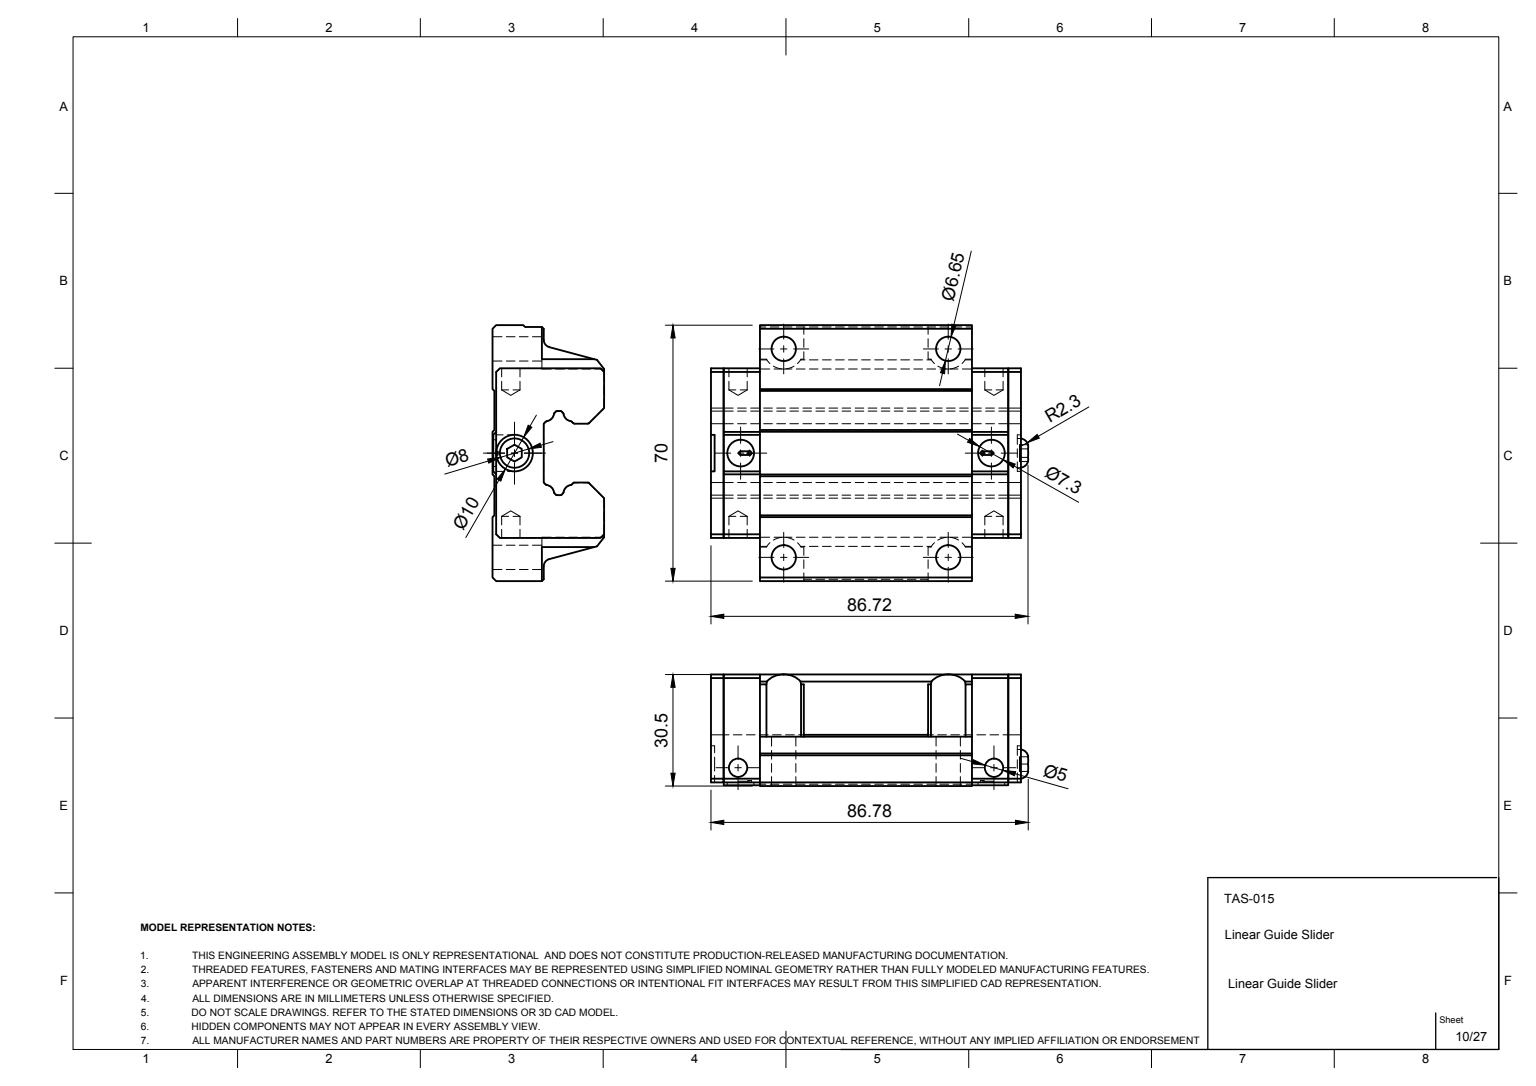
ISO-10303-21;
HEADER;
/* Generated by software containing ST-Developer
 * from STEP Tools, Inc. (www.steptools.com) 
 */

FILE_DESCRIPTION(
/* description */ ('STEP AP214'),
/* implementation_level */ '2;1');

FILE_NAME(
/* name */ 'Linear Guide Slider.step',
/* time_stamp */ '2026-11-15T14:49:54-08:00',
/* author */ (''),
/* organization */ (''),
/* preprocessor_version */ 'ST-DEVELOPER v20.2',
/* originating_system */ 'Autodesk Translation Framework v15.17.0.0',
/* authorisation */ '');

FILE_SCHEMA (('AUTOMOTIVE_DESIGN { 1 0 10303 214 3 1 1 }'));
ENDSEC;

DATA;
#10=MECHANICAL_DESIGN_GEOMETRIC_PRESENTATION_REPRESENTATION('',(#1105),#66721);
#82=(
BOUNDED_CURVE()
B_SPLINE_CURVE(2,(#37654,#37655,#37656),.UNSPECIFIED.,.F.,.F.)
B_SPLINE_CURVE_WITH_KNOTS((3,3),(-1.29356557390797,0.),.UNSPECIFIED.)
CURVE()
GEOMETRIC_REPRESENTATION_ITEM()
RATIONAL_B_SPLINE_CURVE((0.954658532851732,0.77704632554749,1.))
REPRESENTATION_ITEM('')
);
#109=B_SPLINE_CURVE_WITH_KNOTS('',3,(#37621,#37622,#37623,#37624,#37625,
#37626,#37627,#37628,#37629,#37630),.UNSPECIFIED.,.F.,.F.,(4,2,2,2,4),(-0.991617660219933,
-0.988360888345703,-0.882558915285875,-0.776756942226048,-0.773500170351817),
 .UNSPECIFIED.);
#110=B_SPLINE_CURVE_WITH_KNOTS('',3,(#37632,#37633,#37634,#37635,#37636,
#37637,#37638,#37639,#37640,#37641),.UNSPECIFIED.,.F.,.F.,(4,2,2,2,4),(-0.991617660219933,
-0.988360888345703,-0.882558915285875,-0.776756942226048,-0.773500170351817),
 .UNSPECIFIED.);
#111=B_SPLINE_CURVE_WITH_KNOTS('',3,(#37643,#37644,#37645,#37646,#37647,
#37648,#37649,#37650,#37651,#37652),.UNSPECIFIED.,.F.,.F.,(4,2,2,2,4),(-0.991617660219934,
-0.988360888345704,-0.882558915285876,-0.776756942226048,-0.773500170351818),
 .UNSPECIFIED.);
#112=B_SPLINE_CURVE_WITH_KNOTS('',3,(#37661,#37662,#37663,#37664,#37665,
#37666,#37667,#37668,#37669,#37670),.UNSPECIFIED.,.F.,.F.,(4,2,2,2,4),(0.773500170351818,
0.776756942226048,0.882558915285876,0.988360888345703,0.991617660219934),
 .UNSPECIFIED.);
#113=B_SPLINE_CURVE_WITH_KNOTS('',3,(#37672,#37673,#37674,#37675,#37676,
#37677,#37678,#37679,#37680,#37681),.UNSPECIFIED.,.F.,.F.,(4,2,2,2,4),(0.773500170351817,
0.776756942226048,0.882558915285875,0.988360888345703,0.991617660219933),
 .UNSPECIFIED.);
#114=B_SPLINE_CURVE_WITH_KNOTS('',3,(#37682,#37683,#37684,#37685,#37686,
#37687,#37688,#37689,#37690,#37691),.UNSPECIFIED.,.F.,.F.,(4,2,2,2,4),(0.773500170351818,
0.776756942226048,0.882558915285876,0.988360888345704,0.991617660219934),
 .UNSPECIFIED.);
#402=(
BOUNDED_SURFACE()
B_SPLINE_SURFACE(2,2,((#37592,#37593,#37594,#37595,#37596,#37597,#37598,
#37599,#37600),(#37601,#37602,#37603,#37604,#37605,#37606,#37607,#37608,
#37609),(#37610,#37611,#37612,#37613,#37614,#37615,#37616,#37617,#37618)),
 .UNSPECIFIED.,.F.,.T.,.F.)
B_SPLINE_SURFACE_WITH_KNOTS((3,3),(3,2,2,2,3),(0.,1.43998883071719),(-3.14159265358979,
-1.5707963267949,0.,1.5707963267949,3.14159265358979),.UNSPECIFIED.)
GEOMETRIC_REPRESENTATION_ITEM()
RATIONAL_B_SPLINE_SURFACE(((1.,0.707106781186548,1.,0.707106781186548,1.,
0.707106781186548,1.,0.707106781186548,1.),(0.751809411556116,0.531609533071198,
0.751809411556116,0.531609533071198,0.751809411556116,0.531609533071198,
0.751809411556116,0.531609533071198,0.751809411556116),(1.,0.707106781186548,
1.,0.707106781186548,1.,0.707106781186548,1.,0.707106781186548,1.)))
REPRESENTATION_ITEM('')
SURFACE()
);
#524=CONICAL_SURFACE('',#26602,2.5,1.02974425867665);
#525=CONICAL_SURFACE('',#26603,2.5,1.02974425867665);
#526=CONICAL_SURFACE('',#26629,2.5,1.02974425867665);
#527=CONICAL_SURFACE('',#26630,2.5,1.02974425867665);
#642=ELLIPSE('',#26643,6.97960018289555,5.49999999999817);
#643=ELLIPSE('',#26645,6.97960018289945,5.50000000000025);
#644=ELLIPSE('',#26646,6.97960018289465,5.49999999999756);
#645=ELLIPSE('',#26648,6.97960018289959,5.50000000000032);
#646=ELLIPSE('',#26649,6.97960018289765,5.49999999999922);
#647=ELLIPSE('',#26651,6.9796001828989,5.49999999999987);
#648=ELLIPSE('',#26972,21.2503681783598,5.50000000000001);
#649=ELLIPSE('',#26973,21.2503681783597,5.5);
#650=ELLIPSE('',#26978,21.2503681783597,5.5);
#651=ELLIPSE('',#26983,21.2503681783597,5.5);
#652=ELLIPSE('',#26985,21.2503681783597,5.49999999999999);
#653=ELLIPSE('',#26986,21.2503681783597,5.5);
#654=ELLIPSE('',#27079,21.2503681783598,5.50000000000001);
#655=ELLIPSE('',#27081,21.2503681783597,5.49999999999999);
#656=ELLIPSE('',#27086,6.97960018290351,5.50000000000224);
#657=ELLIPSE('',#27091,6.97960018290198,5.50000000000146);
#1043=SHAPE_REPRESENTATION_RELATIONSHIP('SRR','None',#66901,#1074);
#1074=ADVANCED_BREP_SHAPE_REPRESENTATION('',(#1140),#66692);
#1105=STYLED_ITEM('',(#67095),#1140);
#1140=MANIFOLD_SOLID_BREP('Body1',#25671);
#1277=FACE_BOUND('',#4113,.T.);
#1278=FACE_BOUND('',#4116,.T.);
#1279=FACE_BOUND('',#4131,.T.);
#1280=FACE_BOUND('',#4229,.T.);
#1281=FACE_BOUND('',#4242,.T.);
#1282=FACE_BOUND('',#4250,.T.);
#1283=FACE_BOUND('',#4253,.T.);
#1284=FACE_BOUND('',#4258,.T.);
#1285=FACE_BOUND('',#4306,.T.);
#1286=FACE_BOUND('',#4311,.T.);
#1287=FACE_BOUND('',#4313,.T.);
#1288=FACE_BOUND('',#4320,.T.);
#1289=FACE_BOUND('',#4321,.T.);
#1290=FACE_BOUND('',#4330,.T.);
#1291=FACE_BOUND('',#4331,.T.);
#1292=FACE_BOUND('',#4337,.T.);
#1293=FACE_BOUND('',#4343,.T.);
#1294=FACE_BOUND('',#4350,.T.);
#1295=FACE_BOUND('',#4355,.T.);
#1296=FACE_BOUND('',#4390,.T.);
#1297=FACE_BOUND('',#4402,.T.);
#1298=FACE_BOUND('',#4404,.T.);
#1637=PLANE('',#26642);
#1638=PLANE('',#26644);
#1639=PLANE('',#26647);
#1640=PLANE('',#26650);
#1641=PLANE('',#26652);
#1642=PLANE('',#26653);
#1643=PLANE('',#26654);
#1644=PLANE('',#26655);
#1645=PLANE('',#26656);
#1646=PLANE('',#26657);
#1647=PLANE('',#26658);
#1648=PLANE('',#26659);
#1649=PLANE('',#26660);
#1650=PLANE('',#26661);
#1651=PLANE('',#26662);
#1652=PLANE('',#26663);
#1653=PLANE('',#26664);
#1654=PLANE('',#26665);
#1655=PLANE('',#26666);
#1656=PLANE('',#26667);
#1657=PLANE('',#26668);
#1658=PLANE('',#26729);
#1659=PLANE('',#26730);
#1660=PLANE('',#26731);
#1661=PLANE('',#26732);
#1662=PLANE('',#26733);
#1663=PLANE('',#26734);
#1664=PLANE('',#26735);
#1665=PLANE('',#26736);
#1666=PLANE('',#26737);
#1667=PLANE('',#26738);
#1668=PLANE('',#26739);
#1669=PLANE('',#26740);
#1670=PLANE('',#26741);
#1671=PLANE('',#26742);
#1672=PLANE('',#26743);
#1673=PLANE('',#26744);
#1674=PLANE('',#26745);
#1675=PLANE('',#26766);
#1676=PLANE('',#26769);
#1677=PLANE('',#26772);
#1678=PLANE('',#26779);
#1679=PLANE('',#26782);
#1680=PLANE('',#26785);
#1681=PLANE('',#26792);
#1682=PLANE('',#26793);
#1683=PLANE('',#26794);
#1684=PLANE('',#26801);
#1685=PLANE('',#26804);
#1686=PLANE('',#26807);
#1687=PLANE('',#26814);
#1688=PLANE('',#26817);
#1689=PLANE('',#26820);
#1690=PLANE('',#26821);
#1691=PLANE('',#26822);
#1692=PLANE('',#26823);
#1693=PLANE('',#26824);
#1694=PLANE('',#26825);
#1695=PLANE('',#26826);
#1696=PLANE('',#26827);
#1697=PLANE('',#26828);
#1698=PLANE('',#26829);
#1699=PLANE('',#26830);
#1700=PLANE('',#26831);
#1701=PLANE('',#26833);
#1702=PLANE('',#26855);
#1703=PLANE('',#26856);
#1704=PLANE('',#26859);
#1705=PLANE('',#26860);
#1706=PLANE('',#26862);
#1707=PLANE('',#26863);
#1708=PLANE('',#26864);
#1709=PLANE('',#26865);
#1710=PLANE('',#26866);
#1711=PLANE('',#26867);
#1712=PLANE('',#26868);
#1713=PLANE('',#26869);
#1714=PLANE('',#26870);
#1715=PLANE('',#26871);
#1716=PLANE('',#26874);
#1717=PLANE('',#26877);
#1718=PLANE('',#26884);
#1719=PLANE('',#26887);
#1720=PLANE('',#26890);
#1721=PLANE('',#26897);
#1722=PLANE('',#26898);
#1723=PLANE('',#26899);
#1724=PLANE('',#26906);
#1725=PLANE('',#26909);
#1726=PLANE('',#26912);
#1727=PLANE('',#26919);
#1728=PLANE('',#26922);
#1729=PLANE('',#26925);
#1730=PLANE('',#26926);
#1731=PLANE('',#26927);
#1732=PLANE('',#26928);
#1733=PLANE('',#26929);
#1734=PLANE('',#26930);
#1735=PLANE('',#26936);
#1736=PLANE('',#26937);
#1737=PLANE('',#26938);
#1738=PLANE('',#26939);
#1739=PLANE('',#26943);
#1740=PLANE('',#26964);
#1741=PLANE('',#26965);
#1742=PLANE('',#26966);
#1743=PLANE('',#26967);
#1744=PLANE('',#26968);
#1745=PLANE('',#26969);
#1746=PLANE('',#26970);
#1747=PLANE('',#26971);
#1748=PLANE('',#26974);
#1749=PLANE('',#26976);
#1750=PLANE('',#26977);
#1751=PLANE('',#26979);
#1752=PLANE('',#26980);
#1753=PLANE('',#26982);
#1754=PLANE('',#26984);
#1755=PLANE('',#26987);
#1756=PLANE('',#26988);
#1757=PLANE('',#26989);
#1758=PLANE('',#26990);
#1759=PLANE('',#26991);
#1760=PLANE('',#26992);
#1761=PLANE('',#26993);
#1762=PLANE('',#26994);
#1763=PLANE('',#26995);
#1764=PLANE('',#26996);
#1765=PLANE('',#26999);
#1766=PLANE('',#27002);
#1767=PLANE('',#27009);
#1768=PLANE('',#27012);
#1769=PLANE('',#27015);
#1770=PLANE('',#27022);
#1771=PLANE('',#27023);
#1772=PLANE('',#27024);
#1773=PLANE('',#27031);
#1774=PLANE('',#27034);
#1775=PLANE('',#27037);
#1776=PLANE('',#27044);
#1777=PLANE('',#27047);
#1778=PLANE('',#27050);
#1779=PLANE('',#27051);
#1780=PLANE('',#27052);
#1781=PLANE('',#27053);
#1782=PLANE('',#27054);
#1783=PLANE('',#27055);
#1784=PLANE('',#27056);
#1785=PLANE('',#27057);
#1786=PLANE('',#27058);
#1787=PLANE('',#27059);
#1788=PLANE('',#27060);
#1789=PLANE('',#27061);
#1790=PLANE('',#27062);
#1791=PLANE('',#27063);
#1792=PLANE('',#27064);
#1793=PLANE('',#27065);
#1794=PLANE('',#27066);
#1795=PLANE('',#27067);
#1796=PLANE('',#27068);
#1797=PLANE('',#27069);
#1798=PLANE('',#27070);
#1799=PLANE('',#27071);
#1800=PLANE('',#27072);
#1801=PLANE('',#27073);
#1802=PLANE('',#27074);
#1803=PLANE('',#27075);
#1804=PLANE('',#27077);
#1805=PLANE('',#27078);
#1806=PLANE('',#27080);
#1807=PLANE('',#27082);
#1808=PLANE('',#27083);
#1809=PLANE('',#27085);
#1810=PLANE('',#27087);
#1811=PLANE('',#27088);
#1812=PLANE('',#27089);
#1813=PLANE('',#27090);
#1814=PLANE('',#27092);
#1815=PLANE('',#27113);
#1816=PLANE('',#27114);
#1817=PLANE('',#27115);
#1818=PLANE('',#27116);
#1819=PLANE('',#27117);
#1820=PLANE('',#27118);
#1821=PLANE('',#27123);
#1822=PLANE('',#27124);
#1823=PLANE('',#27125);
#1824=PLANE('',#27136);
#1825=PLANE('',#27137);
#1826=PLANE('',#27144);
#1827=PLANE('',#27145);
#1828=PLANE('',#27156);
#1829=PLANE('',#27157);
#1830=PLANE('',#27158);
#1831=PLANE('',#27169);
#1832=PLANE('',#27170);
#1833=PLANE('',#27171);
#1834=PLANE('',#27172);
#1835=PLANE('',#27173);
#1836=PLANE('',#27174);
#1837=PLANE('',#27175);
#1838=PLANE('',#27176);
#1839=PLANE('',#27177);
#1840=PLANE('',#27178);
#1841=PLANE('',#27179);
#1842=PLANE('',#27180);
#1843=PLANE('',#27181);
#1844=PLANE('',#27182);
#1845=PLANE('',#27183);
#1846=PLANE('',#27186);
#1847=PLANE('',#27187);
#2501=FACE_OUTER_BOUND('',#4052,.T.);
#2502=FACE_OUTER_BOUND('',#4053,.T.);
#2503=FACE_OUTER_BOUND('',#4054,.T.);
#2504=FACE_OUTER_BOUND('',#4055,.T.);
#2505=FACE_OUTER_BOUND('',#4056,.T.);
#2506=FACE_OUTER_BOUND('',#4057,.T.);
#2507=FACE_OUTER_BOUND('',#4058,.T.);
#2508=FACE_OUTER_BOUND('',#4059,.T.);
#2509=FACE_OUTER_BOUND('',#4060,.T.);
#2510=FACE_OUTER_BOUND('',#4061,.T.);
#2511=FACE_OUTER_BOUND('',#4062,.T.);
#2512=FACE_OUTER_BOUND('',#4063,.T.);
#2513=FACE_OUTER_BOUND('',#4064,.T.);
#2514=FACE_OUTER_BOUND('',#4065,.T.);
#2515=FACE_OUTER_BOUND('',#4066,.T.);
#2516=FACE_OUTER_BOUND('',#4067,.T.);
#2517=FACE_OUTER_BOUND('',#4068,.T.);
#2518=FACE_OUTER_BOUND('',#4069,.T.);
#2519=FACE_OUTER_BOUND('',#4070,.T.);
#2520=FACE_OUTER_BOUND('',#4071,.T.);
#2521=FACE_OUTER_BOUND('',#4072,.T.);
#2522=FACE_OUTER_BOUND('',#4073,.T.);
#2523=FACE_OUTER_BOUND('',#4074,.T.);
#2524=FACE_OUTER_BOUND('',#4075,.T.);
#2525=FACE_OUTER_BOUND('',#4076,.T.);
#2526=FACE_OUTER_BOUND('',#4077,.T.);
#2527=FACE_OUTER_BOUND('',#4078,.T.);
#2528=FACE_OUTER_BOUND('',#4079,.T.);
#2529=FACE_OUTER_BOUND('',#4080,.T.);
#2530=FACE_OUTER_BOUND('',#4081,.T.);
#2531=FACE_OUTER_BOUND('',#4082,.T.);
#2532=FACE_OUTER_BOUND('',#4083,.T.);
#2533=FACE_OUTER_BOUND('',#4084,.T.);
#2534=FACE_OUTER_BOUND('',#4085,.T.);
#2535=FACE_OUTER_BOUND('',#4086,.T.);
#2536=FACE_OUTER_BOUND('',#4087,.T.);
#2537=FACE_OUTER_BOUND('',#4088,.T.);
#2538=FACE_OUTER_BOUND('',#4089,.T.);
#2539=FACE_OUTER_BOUND('',#4090,.T.);
#2540=FACE_OUTER_BOUND('',#4091,.T.);
#2541=FACE_OUTER_BOUND('',#4092,.T.);
#2542=FACE_OUTER_BOUND('',#4093,.T.);
#2543=FACE_OUTER_BOUND('',#4094,.T.);
#2544=FACE_OUTER_BOUND('',#4095,.T.);
#2545=FACE_OUTER_BOUND('',#4096,.T.);
#2546=FACE_OUTER_BOUND('',#4097,.T.);
#2547=FACE_OUTER_BOUND('',#4098,.T.);
#2548=FACE_OUTER_BOUND('',#4099,.T.);
#2549=FACE_OUTER_BOUND('',#4100,.T.);
#2550=FACE_OUTER_BOUND('',#4101,.T.);
#2551=FACE_OUTER_BOUND('',#4102,.T.);
#2552=FACE_OUTER_BOUND('',#4103,.T.);
#2553=FACE_OUTER_BOUND('',#4104,.T.);
#2554=FACE_OUTER_BOUND('',#4105,.T.);
#2555=FACE_OUTER_BOUND('',#4106,.T.);
#2556=FACE_OUTER_BOUND('',#4107,.T.);
#2557=FACE_OUTER_BOUND('',#4108,.T.);
#2558=FACE_OUTER_BOUND('',#4109,.T.);
#2559=FACE_OUTER_BOUND('',#4110,.T.);
#2560=FACE_OUTER_BOUND('',#4111,.T.);
#2561=FACE_OUTER_BOUND('',#4112,.T.);
#2562=FACE_OUTER_BOUND('',#4114,.T.);
#2563=FACE_OUTER_BOUND('',#4115,.T.);
#2564=FACE_OUTER_BOUND('',#4117,.T.);
#2565=FACE_OUTER_BOUND('',#4118,.T.);
#2566=FACE_OUTER_BOUND('',#4119,.T.);
#2567=FACE_OUTER_BOUND('',#4120,.T.);
#2568=FACE_OUTER_BOUND('',#4121,.T.);
#2569=FACE_OUTER_BOUND('',#4122,.T.);
#2570=FACE_OUTER_BOUND('',#4123,.T.);
#2571=FACE_OUTER_BOUND('',#4124,.T.);
#2572=FACE_OUTER_BOUND('',#4125,.T.);
#2573=FACE_OUTER_BOUND('',#4126,.T.);
#2574=FACE_OUTER_BOUND('',#4127,.T.);
#2575=FACE_OUTER_BOUND('',#4128,.T.);
#2576=FACE_OUTER_BOUND('',#4129,.T.);
#2577=FACE_OUTER_BOUND('',#4130,.T.);
#2578=FACE_OUTER_BOUND('',#4132,.T.);
#2579=FACE_OUTER_BOUND('',#4133,.T.);
#2580=FACE_OUTER_BOUND('',#4134,.T.);
#2581=FACE_OUTER_BOUND('',#4135,.T.);
#2582=FACE_OUTER_BOUND('',#4136,.T.);
#2583=FACE_OUTER_BOUND('',#4137,.T.);
#2584=FACE_OUTER_BOUND('',#4138,.T.);
#2585=FACE_OUTER_BOUND('',#4139,.T.);
#2586=FACE_OUTER_BOUND('',#4140,.T.);
#2587=FACE_OUTER_BOUND('',#4141,.T.);
#2588=FACE_OUTER_BOUND('',#4142,.T.);
#2589=FACE_OUTER_BOUND('',#4143,.T.);
#2590=FACE_OUTER_BOUND('',#4144,.T.);
#2591=FACE_OUTER_BOUND('',#4145,.T.);
#2592=FACE_OUTER_BOUND('',#4146,.T.);
#2593=FACE_OUTER_BOUND('',#4147,.T.);
#2594=FACE_OUTER_BOUND('',#4148,.T.);
#2595=FACE_OUTER_BOUND('',#4149,.T.);
#2596=FACE_OUTER_BOUND('',#4150,.T.);
#2597=FACE_OUTER_BOUND('',#4151,.T.);
#2598=FACE_OUTER_BOUND('',#4152,.T.);
#2599=FACE_OUTER_BOUND('',#4153,.T.);
#2600=FACE_OUTER_BOUND('',#4154,.T.);
#2601=FACE_OUTER_BOUND('',#4155,.T.);
#2602=FACE_OUTER_BOUND('',#4156,.T.);
#2603=FACE_OUTER_BOUND('',#4157,.T.);
#2604=FACE_OUTER_BOUND('',#4158,.T.);
#2605=FACE_OUTER_BOUND('',#4159,.T.);
#2606=FACE_OUTER_BOUND('',#4160,.T.);
#2607=FACE_OUTER_BOUND('',#4161,.T.);
#2608=FACE_OUTER_BOUND('',#4162,.T.);
#2609=FACE_OUTER_BOUND('',#4163,.T.);
#2610=FACE_OUTER_BOUND('',#4164,.T.);
#2611=FACE_OUTER_BOUND('',#4165,.T.);
#2612=FACE_OUTER_BOUND('',#4166,.T.);
#2613=FACE_OUTER_BOUND('',#4167,.T.);
#2614=FACE_OUTER_BOUND('',#4168,.T.);
#2615=FACE_OUTER_BOUND('',#4169,.T.);
#2616=FACE_OUTER_BOUND('',#4170,.T.);
#2617=FACE_OUTER_BOUND('',#4171,.T.);
#2618=FACE_OUTER_BOUND('',#4172,.T.);
#2619=FACE_OUTER_BOUND('',#4173,.T.);
#2620=FACE_OUTER_BOUND('',#4174,.T.);
#2621=FACE_OUTER_BOUND('',#4175,.T.);
#2622=FACE_OUTER_BOUND('',#4176,.T.);
#2623=FACE_OUTER_BOUND('',#4177,.T.);
#2624=FACE_OUTER_BOUND('',#4178,.T.);
#2625=FACE_OUTER_BOUND('',#4179,.T.);
#2626=FACE_OUTER_BOUND('',#4180,.T.);
#2627=FACE_OUTER_BOUND('',#4181,.T.);
#2628=FACE_OUTER_BOUND('',#4182,.T.);
#2629=FACE_OUTER_BOUND('',#4183,.T.);
#2630=FACE_OUTER_BOUND('',#4184,.T.);
#2631=FACE_OUTER_BOUND('',#4185,.T.);
#2632=FACE_OUTER_BOUND('',#4186,.T.);
#2633=FACE_OUTER_BOUND('',#4187,.T.);
#2634=FACE_OUTER_BOUND('',#4188,.T.);
#2635=FACE_OUTER_BOUND('',#4189,.T.);
#2636=FACE_OUTER_BOUND('',#4190,.T.);
#2637=FACE_OUTER_BOUND('',#4191,.T.);
#2638=FACE_OUTER_BOUND('',#4192,.T.);
#2639=FACE_OUTER_BOUND('',#4193,.T.);
#2640=FACE_OUTER_BOUND('',#4194,.T.);
#2641=FACE_OUTER_BOUND('',#4195,.T.);
#2642=FACE_OUTER_BOUND('',#4196,.T.);
#2643=FACE_OUTER_BOUND('',#4197,.T.);
#2644=FACE_OUTER_BOUND('',#4198,.T.);
#2645=FACE_OUTER_BOUND('',#4199,.T.);
#2646=FACE_OUTER_BOUND('',#4200,.T.);
#2647=FACE_OUTER_BOUND('',#4201,.T.);
#2648=FACE_OUTER_BOUND('',#4202,.T.);
#2649=FACE_OUTER_BOUND('',#4203,.T.);
#2650=FACE_OUTER_BOUND('',#4204,.T.);
#2651=FACE_OUTER_BOUND('',#4205,.T.);
#2652=FACE_OUTER_BOUND('',#4206,.T.);
#2653=FACE_OUTER_BOUND('',#4207,.T.);
#2654=FACE_OUTER_BOUND('',#4208,.T.);
#2655=FACE_OUTER_BOUND('',#4209,.T.);
#2656=FACE_OUTER_BOUND('',#4210,.T.);
#2657=FACE_OUTER_BOUND('',#4211,.T.);
#2658=FACE_OUTER_BOUND('',#4212,.T.);
#2659=FACE_OUTER_BOUND('',#4213,.T.);
#2660=FACE_OUTER_BOUND('',#4214,.T.);
#2661=FACE_OUTER_BOUND('',#4215,.T.);
#2662=FACE_OUTER_BOUND('',#4216,.T.);
#2663=FACE_OUTER_BOUND('',#4217,.T.);
#2664=FACE_OUTER_BOUND('',#4218,.T.);
#2665=FACE_OUTER_BOUND('',#4219,.T.);
#2666=FACE_OUTER_BOUND('',#4220,.T.);
#2667=FACE_OUTER_BOUND('',#4221,.T.);
#2668=FACE_OUTER_BOUND('',#4222,.T.);
#2669=FACE_OUTER_BOUND('',#4223,.T.);
#2670=FACE_OUTER_BOUND('',#4224,.T.);
#2671=FACE_OUTER_BOUND('',#4225,.T.);
#2672=FACE_OUTER_BOUND('',#4226,.T.);
#2673=FACE_OUTER_BOUND('',#4227,.T.);
#2674=FACE_OUTER_BOUND('',#4228,.T.);
#2675=FACE_OUTER_BOUND('',#4230,.T.);
#2676=FACE_OUTER_BOUND('',#4231,.T.);
#2677=FACE_OUTER_BOUND('',#4232,.T.);
#2678=FACE_OUTER_BOUND('',#4233,.T.);
#2679=FACE_OUTER_BOUND('',#4234,.T.);
#2680=FACE_OUTER_BOUND('',#4235,.T.);
#2681=FACE_OUTER_BOUND('',#4236,.T.);
#2682=FACE_OUTER_BOUND('',#4237,.T.);
#2683=FACE_OUTER_BOUND('',#4238,.T.);
#2684=FACE_OUTER_BOUND('',#4239,.T.);
#2685=FACE_OUTER_BOUND('',#4240,.T.);
#2686=FACE_OUTER_BOUND('',#4241,.T.);
#2687=FACE_OUTER_BOUND('',#4243,.T.);
#2688=FACE_OUTER_BOUND('',#4244,.T.);
#2689=FACE_OUTER_BOUND('',#4245,.T.);
#2690=FACE_OUTER_BOUND('',#4246,.T.);
#2691=FACE_OUTER_BOUND('',#4247,.T.);
#2692=FACE_OUTER_BOUND('',#4248,.T.);
#2693=FACE_OUTER_BOUND('',#4249,.T.);
#2694=FACE_OUTER_BOUND('',#4251,.T.);
#2695=FACE_OUTER_BOUND('',#4252,.T.);
#2696=FACE_OUTER_BOUND('',#4254,.T.);
#2697=FACE_OUTER_BOUND('',#4255,.T.);
#2698=FACE_OUTER_BOUND('',#4256,.T.);
#2699=FACE_OUTER_BOUND('',#4257,.T.);
#2700=FACE_OUTER_BOUND('',#4259,.T.);
#2701=FACE_OUTER_BOUND('',#4260,.T.);
#2702=FACE_OUTER_BOUND('',#4261,.T.);
#2703=FACE_OUTER_BOUND('',#4262,.T.);
#2704=FACE_OUTER_BOUND('',#4263,.T.);
#2705=FACE_OUTER_BOUND('',#4264,.T.);
#2706=FACE_OUTER_BOUND('',#4265,.T.);
#2707=FACE_OUTER_BOUND('',#4266,.T.);
#2708=FACE_OUTER_BOUND('',#4267,.T.);
#2709=FACE_OUTER_BOUND('',#4268,.T.);
#2710=FACE_OUTER_BOUND('',#4269,.T.);
#2711=FACE_OUTER_BOUND('',#4270,.T.);
#2712=FACE_OUTER_BOUND('',#4271,.T.);
#2713=FACE_OUTER_BOUND('',#4272,.T.);
#2714=FACE_OUTER_BOUND('',#4273,.T.);
#2715=FACE_OUTER_BOUND('',#4274,.T.);
#2716=FACE_OUTER_BOUND('',#4275,.T.);
#2717=FACE_OUTER_BOUND('',#4276,.T.);
#2718=FACE_OUTER_BOUND('',#4277,.T.);
#2719=FACE_OUTER_BOUND('',#4278,.T.);
#2720=FACE_OUTER_BOUND('',#4279,.T.);
#2721=FACE_OUTER_BOUND('',#4280,.T.);
#2722=FACE_OUTER_BOUND('',#4281,.T.);
#2723=FACE_OUTER_BOUND('',#4282,.T.);
#2724=FACE_OUTER_BOUND('',#4283,.T.);
#2725=FACE_OUTER_BOUND('',#4284,.T.);
#2726=FACE_OUTER_BOUND('',#4285,.T.);
#2727=FACE_OUTER_BOUND('',#4286,.T.);
#2728=FACE_OUTER_BOUND('',#4287,.T.);
#2729=FACE_OUTER_BOUND('',#4288,.T.);
#2730=FACE_OUTER_BOUND('',#4289,.T.);
#2731=FACE_OUTER_BOUND('',#4290,.T.);
#2732=FACE_OUTER_BOUND('',#4291,.T.);
#2733=FACE_OUTER_BOUND('',#4292,.T.);
#2734=FACE_OUTER_BOUND('',#4293,.T.);
#2735=FACE_OUTER_BOUND('',#4294,.T.);
#2736=FACE_OUTER_BOUND('',#4295,.T.);
#2737=FACE_OUTER_BOUND('',#4296,.T.);
#2738=FACE_OUTER_BOUND('',#4297,.T.);
#2739=FACE_OUTER_BOUND('',#4298,.T.);
#2740=FACE_OUTER_BOUND('',#4299,.T.);
#2741=FACE_OUTER_BOUND('',#4300,.T.);
#2742=FACE_OUTER_BOUND('',#4301,.T.);
#2743=FACE_OUTER_BOUND('',#4302,.T.);
#2744=FACE_OUTER_BOUND('',#4303,.T.);
#2745=FACE_OUTER_BOUND('',#4304,.T.);
#2746=FACE_OUTER_BOUND('',#4305,.T.);
#2747=FACE_OUTER_BOUND('',#4307,.T.);
#2748=FACE_OUTER_BOUND('',#4308,.T.);
#2749=FACE_OUTER_BOUND('',#4309,.T.);
#2750=FACE_OUTER_BOUND('',#4310,.T.);
#2751=FACE_OUTER_BOUND('',#4312,.T.);
#2752=FACE_OUTER_BOUND('',#4314,.T.);
#2753=FACE_OUTER_BOUND('',#4315,.T.);
#2754=FACE_OUTER_BOUND('',#4316,.T.);
#2755=FACE_OUTER_BOUND('',#4317,.T.);
#2756=FACE_OUTER_BOUND('',#4318,.T.);
#2757=FACE_OUTER_BOUND('',#4319,.T.);
#2758=FACE_OUTER_BOUND('',#4322,.T.);
#2759=FACE_OUTER_BOUND('',#4323,.T.);
#2760=FACE_OUTER_BOUND('',#4324,.T.);
#2761=FACE_OUTER_BOUND('',#4325,.T.);
#2762=FACE_OUTER_BOUND('',#4326,.T.);
#2763=FACE_OUTER_BOUND('',#4327,.T.);
#2764=FACE_OUTER_BOUND('',#4328,.T.);
#2765=FACE_OUTER_BOUND('',#4329,.T.);
#2766=FACE_OUTER_BOUND('',#4332,.T.);
#2767=FACE_OUTER_BOUND('',#4333,.T.);
#2768=FACE_OUTER_BOUND('',#4334,.T.);
#2769=FACE_OUTER_BOUND('',#4335,.T.);
#2770=FACE_OUTER_BOUND('',#4336,.T.);
#2771=FACE_OUTER_BOUND('',#4338,.T.);
#2772=FACE_OUTER_BOUND('',#4339,.T.);
#2773=FACE_OUTER_BOUND('',#4340,.T.);
#2774=FACE_OUTER_BOUND('',#4341,.T.);
#2775=FACE_OUTER_BOUND('',#4342,.T.);
#2776=FACE_OUTER_BOUND('',#4344,.T.);
#2777=FACE_OUTER_BOUND('',#4345,.T.);
#2778=FACE_OUTER_BOUND('',#4346,.T.);
#2779=FACE_OUTER_BOUND('',#4347,.T.);
#2780=FACE_OUTER_BOUND('',#4348,.T.);
#2781=FACE_OUTER_BOUND('',#4349,.T.);
#2782=FACE_OUTER_BOUND('',#4351,.T.);
#2783=FACE_OUTER_BOUND('',#4352,.T.);
#2784=FACE_OUTER_BOUND('',#4353,.T.);
#2785=FACE_OUTER_BOUND('',#4354,.T.);
#2786=FACE_OUTER_BOUND('',#4356,.T.);
#2787=FACE_OUTER_BOUND('',#4357,.T.);
#2788=FACE_OUTER_BOUND('',#4358,.T.);
#2789=FACE_OUTER_BOUND('',#4359,.T.);
#2790=FACE_OUTER_BOUND('',#4360,.T.);
#2791=FACE_OUTER_BOUND('',#4361,.T.);
#2792=FACE_OUTER_BOUND('',#4362,.T.);
#2793=FACE_OUTER_BOUND('',#4363,.T.);
#2794=FACE_OUTER_BOUND('',#4364,.T.);
#2795=FACE_OUTER_BOUND('',#4365,.T.);
#2796=FACE_OUTER_BOUND('',#4366,.T.);
#2797=FACE_OUTER_BOUND('',#4367,.T.);
#2798=FACE_OUTER_BOUND('',#4368,.T.);
#2799=FACE_OUTER_BOUND('',#4369,.T.);
#2800=FACE_OUTER_BOUND('',#4370,.T.);
#2801=FACE_OUTER_BOUND('',#4371,.T.);
#2802=FACE_OUTER_BOUND('',#4372,.T.);
#2803=FACE_OUTER_BOUND('',#4373,.T.);
#2804=FACE_OUTER_BOUND('',#4374,.T.);
#2805=FACE_OUTER_BOUND('',#4375,.T.);
#2806=FACE_OUTER_BOUND('',#4376,.T.);
#2807=FACE_OUTER_BOUND('',#4377,.T.);
#2808=FACE_OUTER_BOUND('',#4378,.T.);
#2809=FACE_OUTER_BOUND('',#4379,.T.);
#2810=FACE_OUTER_BOUND('',#4380,.T.);
#2811=FACE_OUTER_BOUND('',#4381,.T.);
#2812=FACE_OUTER_BOUND('',#4382,.T.);
#2813=FACE_OUTER_BOUND('',#4383,.T.);
#2814=FACE_OUTER_BOUND('',#4384,.T.);
#2815=FACE_OUTER_BOUND('',#4385,.T.);
#2816=FACE_OUTER_BOUND('',#4386,.T.);
#2817=FACE_OUTER_BOUND('',#4387,.T.);
#2818=FACE_OUTER_BOUND('',#4388,.T.);
#2819=FACE_OUTER_BOUND('',#4389,.T.);
#2820=FACE_OUTER_BOUND('',#4391,.T.);
#2821=FACE_OUTER_BOUND('',#4392,.T.);
#2822=FACE_OUTER_BOUND('',#4393,.T.);
#2823=FACE_OUTER_BOUND('',#4394,.T.);
#2824=FACE_OUTER_BOUND('',#4395,.T.);
#2825=FACE_OUTER_BOUND('',#4396,.T.);
#2826=FACE_OUTER_BOUND('',#4397,.T.);
#2827=FACE_OUTER_BOUND('',#4398,.T.);
#2828=FACE_OUTER_BOUND('',#4399,.T.);
#2829=FACE_OUTER_BOUND('',#4400,.T.);
#2830=FACE_OUTER_BOUND('',#4401,.T.);
#2831=FACE_OUTER_BOUND('',#4403,.T.);
#2832=FACE_OUTER_BOUND('',#4405,.T.);
#2833=FACE_OUTER_BOUND('',#4406,.T.);
#2834=FACE_OUTER_BOUND('',#4407,.T.);
#2835=FACE_OUTER_BOUND('',#4408,.T.);
#2836=FACE_OUTER_BOUND('',#4409,.T.);
#2837=FACE_OUTER_BOUND('',#4410,.T.);
#2838=FACE_OUTER_BOUND('',#4411,.T.);
#2839=FACE_OUTER_BOUND('',#4412,.T.);
#4052=EDGE_LOOP('',(#17884,#17885,#17886,#17887));
#4053=EDGE_LOOP('',(#17888,#17889,#17890,#17891));
#4054=EDGE_LOOP('',(#17892,#17893,#17894,#17895));
#4055=EDGE_LOOP('',(#17896,#17897,#17898));
#4056=EDGE_LOOP('',(#17899,#17900,#17901));
#4057=EDGE_LOOP('',(#17902,#17903,#17904,#17905));
#4058=EDGE_LOOP('',(#17906,#17907,#17908,#17909));
#4059=EDGE_LOOP('',(#17910,#17911,#17912,#17913));
#4060=EDGE_LOOP('',(#17914,#17915,#17916,#17917));
#4061=EDGE_LOOP('',(#17918,#17919,#17920,#17921));
#4062=EDGE_LOOP('',(#17922,#17923,#17924,#17925));
#4063=EDGE_LOOP('',(#17926,#17927,#17928,#17929));
#4064=EDGE_LOOP('',(#17930,#17931,#17932,#17933,#17934,#17935,#17936));
#4065=EDGE_LOOP('',(#17937,#17938,#17939));
#4066=EDGE_LOOP('',(#17940,#17941,#17942));
#4067=EDGE_LOOP('',(#17943,#17944,#17945,#17946,#17947,#17948,#17949));
#4068=EDGE_LOOP('',(#17950,#17951,#17952,#17953,#17954,#17955,#17956,#17957,
#17958,#17959));
#4069=EDGE_LOOP('',(#17960,#17961,#17962,#17963,#17964));
#4070=EDGE_LOOP('',(#17965,#17966,#17967,#17968));
#4071=EDGE_LOOP('',(#17969,#17970,#17971,#17972));
#4072=EDGE_LOOP('',(#17973,#17974,#17975,#17976));
#4073=EDGE_LOOP('',(#17977,#17978,#17979,#17980));
#4074=EDGE_LOOP('',(#17981,#17982,#17983,#17984));
#4075=EDGE_LOOP('',(#17985,#17986,#17987,#17988));
#4076=EDGE_LOOP('',(#17989,#17990,#17991,#17992));
#4077=EDGE_LOOP('',(#17993,#17994,#17995,#17996));
#4078=EDGE_LOOP('',(#17997,#17998,#17999,#18000));
#4079=EDGE_LOOP('',(#18001,#18002,#18003,#18004));
#4080=EDGE_LOOP('',(#18005,#18006,#18007,#18008));
#4081=EDGE_LOOP('',(#18009,#18010,#18011,#18012));
#4082=EDGE_LOOP('',(#18013,#18014,#18015,#18016));
#4083=EDGE_LOOP('',(#18017,#18018,#18019,#18020));
#4084=EDGE_LOOP('',(#18021,#18022,#18023,#18024));
#4085=EDGE_LOOP('',(#18025,#18026,#18027,#18028));
#4086=EDGE_LOOP('',(#18029,#18030,#18031,#18032));
#4087=EDGE_LOOP('',(#18033,#18034,#18035,#18036));
#4088=EDGE_LOOP('',(#18037,#18038,#18039,#18040));
#4089=EDGE_LOOP('',(#18041,#18042,#18043,#18044));
#4090=EDGE_LOOP('',(#18045,#18046,#18047,#18048));
#4091=EDGE_LOOP('',(#18049,#18050,#18051,#18052));
#4092=EDGE_LOOP('',(#18053,#18054,#18055,#18056));
#4093=EDGE_LOOP('',(#18057,#18058,#18059,#18060));
#4094=EDGE_LOOP('',(#18061,#18062,#18063,#18064));
#4095=EDGE_LOOP('',(#18065,#18066,#18067,#18068));
#4096=EDGE_LOOP('',(#18069,#18070,#18071,#18072));
#4097=EDGE_LOOP('',(#18073,#18074,#18075,#18076));
#4098=EDGE_LOOP('',(#18077,#18078,#18079,#18080));
#4099=EDGE_LOOP('',(#18081,#18082,#18083,#18084));
#4100=EDGE_LOOP('',(#18085,#18086,#18087,#18088));
#4101=EDGE_LOOP('',(#18089,#18090,#18091,#18092));
#4102=EDGE_LOOP('',(#18093,#18094,#18095,#18096));
#4103=EDGE_LOOP('',(#18097,#18098,#18099,#18100));
#4104=EDGE_LOOP('',(#18101,#18102,#18103,#18104));
#4105=EDGE_LOOP('',(#18105,#18106,#18107,#18108));
#4106=EDGE_LOOP('',(#18109,#18110,#18111,#18112));
#4107=EDGE_LOOP('',(#18113,#18114,#18115,#18116));
#4108=EDGE_LOOP('',(#18117,#18118,#18119,#18120));
#4109=EDGE_LOOP('',(#18121,#18122,#18123,#18124));
#4110=EDGE_LOOP('',(#18125,#18126,#18127,#18128));
#4111=EDGE_LOOP('',(#18129,#18130,#18131,#18132));
#4112=EDGE_LOOP('',(#18133));
#4113=EDGE_LOOP('',(#18134));
#4114=EDGE_LOOP('',(#18135,#18136,#18137,#18138));
#4115=EDGE_LOOP('',(#18139,#18140,#18141,#18142,#18143,#18144,#18145,#18146,
#18147,#18148,#18149,#18150,#18151,#18152,#18153,#18154,#18155,#18156,#18157,
#18158,#18159,#18160,#18161,#18162,#18163,#18164,#18165,#18166,#18167,#18168,
#18169,#18170,#18171,#18172,#18173,#18174,#18175,#18176,#18177,#18178,#18179,
#18180,#18181,#18182));
#4116=EDGE_LOOP('',(#18183));
#4117=EDGE_LOOP('',(#18184,#18185,#18186,#18187));
#4118=EDGE_LOOP('',(#18188,#18189,#18190,#18191));
#4119=EDGE_LOOP('',(#18192,#18193,#18194,#18195));
#4120=EDGE_LOOP('',(#18196,#18197,#18198,#18199));
#4121=EDGE_LOOP('',(#18200,#18201,#18202,#18203));
#4122=EDGE_LOOP('',(#18204,#18205,#18206,#18207));
#4123=EDGE_LOOP('',(#18208,#18209,#18210,#18211));
#4124=EDGE_LOOP('',(#18212,#18213,#18214,#18215));
#4125=EDGE_LOOP('',(#18216,#18217,#18218,#18219));
#4126=EDGE_LOOP('',(#18220,#18221,#18222,#18223));
#4127=EDGE_LOOP('',(#18224,#18225,#18226,#18227));
#4128=EDGE_LOOP('',(#18228,#18229,#18230,#18231));
#4129=EDGE_LOOP('',(#18232,#18233,#18234,#18235,#18236,#18237));
#4130=EDGE_LOOP('',(#18238,#18239,#18240,#18241,#18242,#18243,#18244,#18245,
#18246,#18247,#18248,#18249,#18250,#18251,#18252,#18253,#18254,#18255,#18256,
#18257,#18258,#18259,#18260,#18261,#18262,#18263,#18264,#18265,#18266,#18267,
#18268,#18269,#18270,#18271,#18272,#18273,#18274,#18275,#18276,#18277,#18278,
#18279,#18280,#18281));
#4131=EDGE_LOOP('',(#18282,#18283,#18284,#18285,#18286,#18287,#18288,#18289,
#18290,#18291,#18292,#18293,#18294,#18295,#18296,#18297,#18298,#18299,#18300,
#18301,#18302,#18303,#18304,#18305,#18306,#18307,#18308,#18309,#18310,#18311,
#18312,#18313,#18314,#18315,#18316,#18317,#18318,#18319,#18320,#18321,#18322,
#18323,#18324,#18325));
#4132=EDGE_LOOP('',(#18326,#18327,#18328,#18329));
#4133=EDGE_LOOP('',(#18330,#18331,#18332,#18333));
#4134=EDGE_LOOP('',(#18334,#18335,#18336,#18337));
#4135=EDGE_LOOP('',(#18338,#18339,#18340,#18341));
#4136=EDGE_LOOP('',(#18342,#18343,#18344,#18345));
#4137=EDGE_LOOP('',(#18346,#18347,#18348,#18349));
#4138=EDGE_LOOP('',(#18350,#18351,#18352,#18353));
#4139=EDGE_LOOP('',(#18354,#18355,#18356,#18357));
#4140=EDGE_LOOP('',(#18358,#18359,#18360,#18361));
#4141=EDGE_LOOP('',(#18362,#18363,#18364,#18365));
#4142=EDGE_LOOP('',(#18366,#18367,#18368,#18369));
#4143=EDGE_LOOP('',(#18370,#18371,#18372,#18373));
#4144=EDGE_LOOP('',(#18374,#18375,#18376,#18377));
#4145=EDGE_LOOP('',(#18378,#18379,#18380,#18381));
#4146=EDGE_LOOP('',(#18382,#18383,#18384,#18385));
#4147=EDGE_LOOP('',(#18386,#18387,#18388,#18389));
#4148=EDGE_LOOP('',(#18390,#18391,#18392,#18393));
#4149=EDGE_LOOP('',(#18394,#18395,#18396,#18397));
#4150=EDGE_LOOP('',(#18398,#18399,#18400,#18401));
#4151=EDGE_LOOP('',(#18402,#18403,#18404,#18405));
#4152=EDGE_LOOP('',(#18406,#18407,#18408,#18409));
#4153=EDGE_LOOP('',(#18410,#18411,#18412,#18413));
#4154=EDGE_LOOP('',(#18414,#18415,#18416,#18417));
#4155=EDGE_LOOP('',(#18418,#18419,#18420,#18421));
#4156=EDGE_LOOP('',(#18422,#18423,#18424,#18425));
#4157=EDGE_LOOP('',(#18426,#18427,#18428,#18429));
#4158=EDGE_LOOP('',(#18430,#18431,#18432,#18433));
#4159=EDGE_LOOP('',(#18434,#18435,#18436,#18437));
#4160=EDGE_LOOP('',(#18438,#18439,#18440,#18441));
#4161=EDGE_LOOP('',(#18442,#18443,#18444,#18445));
#4162=EDGE_LOOP('',(#18446,#18447,#18448,#18449));
#4163=EDGE_LOOP('',(#18450,#18451,#18452,#18453));
#4164=EDGE_LOOP('',(#18454,#18455,#18456,#18457));
#4165=EDGE_LOOP('',(#18458,#18459,#18460,#18461));
#4166=EDGE_LOOP('',(#18462,#18463,#18464,#18465));
#4167=EDGE_LOOP('',(#18466,#18467,#18468,#18469));
#4168=EDGE_LOOP('',(#18470,#18471,#18472,#18473));
#4169=EDGE_LOOP('',(#18474,#18475,#18476,#18477));
#4170=EDGE_LOOP('',(#18478,#18479,#18480,#18481));
#4171=EDGE_LOOP('',(#18482,#18483,#18484,#18485));
#4172=EDGE_LOOP('',(#18486,#18487,#18488,#18489));
#4173=EDGE_LOOP('',(#18490,#18491,#18492,#18493));
#4174=EDGE_LOOP('',(#18494,#18495,#18496,#18497));
#4175=EDGE_LOOP('',(#18498,#18499,#18500,#18501));
#4176=EDGE_LOOP('',(#18502));
#4177=EDGE_LOOP('',(#18503,#18504,#18505,#18506));
#4178=EDGE_LOOP('',(#18507,#18508,#18509,#18510,#18511,#18512,#18513,#18514,
#18515,#18516,#18517,#18518,#18519,#18520,#18521,#18522,#18523,#18524,#18525,
#18526,#18527,#18528,#18529,#18530,#18531,#18532,#18533,#18534,#18535,#18536,
#18537,#18538,#18539,#18540,#18541,#18542,#18543,#18544,#18545,#18546,#18547,
#18548,#18549,#18550,#18551,#18552,#18553,#18554));
#4179=EDGE_LOOP('',(#18555,#18556,#18557,#18558));
#4180=EDGE_LOOP('',(#18559,#18560,#18561,#18562));
#4181=EDGE_LOOP('',(#18563,#18564,#18565,#18566));
#4182=EDGE_LOOP('',(#18567));
#4183=EDGE_LOOP('',(#18568,#18569,#18570,#18571));
#4184=EDGE_LOOP('',(#18572,#18573,#18574,#18575));
#4185=EDGE_LOOP('',(#18576,#18577,#18578,#18579));
#4186=EDGE_LOOP('',(#18580,#18581,#18582,#18583));
#4187=EDGE_LOOP('',(#18584,#18585,#18586,#18587));
#4188=EDGE_LOOP('',(#18588,#18589,#18590,#18591,#18592,#18593,#18594,#18595));
#4189=EDGE_LOOP('',(#18596,#18597,#18598,#18599));
#4190=EDGE_LOOP('',(#18600,#18601,#18602,#18603));
#4191=EDGE_LOOP('',(#18604,#18605,#18606,#18607));
#4192=EDGE_LOOP('',(#18608,#18609,#18610,#18611));
#4193=EDGE_LOOP('',(#18612,#18613,#18614,#18615));
#4194=EDGE_LOOP('',(#18616,#18617,#18618,#18619));
#4195=EDGE_LOOP('',(#18620,#18621,#18622,#18623));
#4196=EDGE_LOOP('',(#18624,#18625,#18626,#18627));
#4197=EDGE_LOOP('',(#18628,#18629,#18630,#18631));
#4198=EDGE_LOOP('',(#18632,#18633,#18634,#18635));
#4199=EDGE_LOOP('',(#18636,#18637,#18638,#18639));
#4200=EDGE_LOOP('',(#18640,#18641,#18642,#18643));
#4201=EDGE_LOOP('',(#18644,#18645,#18646,#18647));
#4202=EDGE_LOOP('',(#18648,#18649,#18650,#18651));
#4203=EDGE_LOOP('',(#18652,#18653,#18654,#18655));
#4204=EDGE_LOOP('',(#18656,#18657,#18658,#18659));
#4205=EDGE_LOOP('',(#18660,#18661,#18662,#18663));
#4206=EDGE_LOOP('',(#18664,#18665,#18666,#18667));
#4207=EDGE_LOOP('',(#18668,#18669,#18670,#18671));
#4208=EDGE_LOOP('',(#18672,#18673,#18674,#18675));
#4209=EDGE_LOOP('',(#18676,#18677,#18678,#18679));
#4210=EDGE_LOOP('',(#18680,#18681,#18682,#18683));
#4211=EDGE_LOOP('',(#18684,#18685,#18686,#18687));
#4212=EDGE_LOOP('',(#18688,#18689,#18690,#18691));
#4213=EDGE_LOOP('',(#18692,#18693,#18694,#18695));
#4214=EDGE_LOOP('',(#18696,#18697,#18698,#18699));
#4215=EDGE_LOOP('',(#18700,#18701,#18702,#18703));
#4216=EDGE_LOOP('',(#18704,#18705,#18706,#18707));
#4217=EDGE_LOOP('',(#18708,#18709,#18710,#18711));
#4218=EDGE_LOOP('',(#18712,#18713,#18714,#18715));
#4219=EDGE_LOOP('',(#18716,#18717,#18718,#18719));
#4220=EDGE_LOOP('',(#18720,#18721,#18722,#18723));
#4221=EDGE_LOOP('',(#18724,#18725,#18726,#18727));
#4222=EDGE_LOOP('',(#18728,#18729,#18730,#18731));
#4223=EDGE_LOOP('',(#18732,#18733,#18734,#18735));
#4224=EDGE_LOOP('',(#18736,#18737,#18738,#18739));
#4225=EDGE_LOOP('',(#18740,#18741,#18742,#18743));
#4226=EDGE_LOOP('',(#18744,#18745,#18746,#18747));
#4227=EDGE_LOOP('',(#18748,#18749,#18750,#18751));
#4228=EDGE_LOOP('',(#18752));
#4229=EDGE_LOOP('',(#18753,#18754,#18755,#18756));
#4230=EDGE_LOOP('',(#18757,#18758,#18759,#18760));
#4231=EDGE_LOOP('',(#18761,#18762,#18763,#18764));
#4232=EDGE_LOOP('',(#18765,#18766,#18767,#18768));
#4233=EDGE_LOOP('',(#18769,#18770,#18771,#18772));
#4234=EDGE_LOOP('',(#18773,#18774,#18775,#18776));
#4235=EDGE_LOOP('',(#18777,#18778,#18779,#18780));
#4236=EDGE_LOOP('',(#18781,#18782,#18783,#18784,#18785,#18786));
#4237=EDGE_LOOP('',(#18787,#18788,#18789,#18790));
#4238=EDGE_LOOP('',(#18791,#18792,#18793,#18794));
#4239=EDGE_LOOP('',(#18795,#18796,#18797,#18798,#18799,#18800));
#4240=EDGE_LOOP('',(#18801,#18802,#18803,#18804));
#4241=EDGE_LOOP('',(#18805,#18806,#18807,#18808,#18809,#18810,#18811,#18812,
#18813,#18814,#18815,#18816,#18817,#18818,#18819,#18820,#18821,#18822,#18823,
#18824,#18825,#18826,#18827,#18828,#18829,#18830,#18831,#18832,#18833,#18834,
#18835,#18836,#18837,#18838,#18839,#18840,#18841,#18842,#18843,#18844,#18845,
#18846,#18847,#18848));
#4242=EDGE_LOOP('',(#18849,#18850,#18851,#18852,#18853,#18854,#18855,#18856,
#18857,#18858,#18859,#18860,#18861,#18862,#18863,#18864,#18865,#18866,#18867,
#18868,#18869,#18870,#18871,#18872,#18873,#18874,#18875,#18876,#18877,#18878,
#18879,#18880,#18881,#18882,#18883,#18884,#18885,#18886,#18887,#18888,#18889,
#18890,#18891,#18892));
#4243=EDGE_LOOP('',(#18893,#18894,#18895,#18896));
#4244=EDGE_LOOP('',(#18897,#18898,#18899,#18900));
#4245=EDGE_LOOP('',(#18901,#18902,#18903,#18904,#18905,#18906));
#4246=EDGE_LOOP('',(#18907,#18908,#18909,#18910));
#4247=EDGE_LOOP('',(#18911,#18912,#18913,#18914,#18915,#18916));
#4248=EDGE_LOOP('',(#18917,#18918,#18919,#18920));
#4249=EDGE_LOOP('',(#18921));
#4250=EDGE_LOOP('',(#18922,#18923,#18924,#18925));
#4251=EDGE_LOOP('',(#18926,#18927,#18928,#18929,#18930,#18931,#18932,#18933));
#4252=EDGE_LOOP('',(#18934,#18935,#18936,#18937,#18938,#18939));
#4253=EDGE_LOOP('',(#18940));
#4254=EDGE_LOOP('',(#18941,#18942,#18943,#18944));
#4255=EDGE_LOOP('',(#18945,#18946,#18947,#18948));
#4256=EDGE_LOOP('',(#18949,#18950,#18951,#18952));
#4257=EDGE_LOOP('',(#18953,#18954,#18955,#18956,#18957,#18958));
#4258=EDGE_LOOP('',(#18959));
#4259=EDGE_LOOP('',(#18960,#18961,#18962,#18963));
#4260=EDGE_LOOP('',(#18964,#18965,#18966,#18967,#18968,#18969,#18970,#18971));
#4261=EDGE_LOOP('',(#18972,#18973,#18974,#18975));
#4262=EDGE_LOOP('',(#18976,#18977,#18978,#18979));
#4263=EDGE_LOOP('',(#18980,#18981,#18982,#18983));
#4264=EDGE_LOOP('',(#18984,#18985,#18986,#18987));
#4265=EDGE_LOOP('',(#18988,#18989,#18990,#18991));
#4266=EDGE_LOOP('',(#18992,#18993,#18994,#18995));
#4267=EDGE_LOOP('',(#18996,#18997,#18998,#18999));
#4268=EDGE_LOOP('',(#19000,#19001,#19002,#19003));
#4269=EDGE_LOOP('',(#19004,#19005,#19006,#19007));
#4270=EDGE_LOOP('',(#19008,#19009,#19010,#19011));
#4271=EDGE_LOOP('',(#19012,#19013,#19014,#19015));
#4272=EDGE_LOOP('',(#19016,#19017,#19018,#19019));
#4273=EDGE_LOOP('',(#19020,#19021,#19022,#19023));
#4274=EDGE_LOOP('',(#19024,#19025,#19026,#19027));
#4275=EDGE_LOOP('',(#19028,#19029,#19030,#19031));
#4276=EDGE_LOOP('',(#19032,#19033,#19034,#19035));
#4277=EDGE_LOOP('',(#19036,#19037,#19038,#19039));
#4278=EDGE_LOOP('',(#19040,#19041,#19042,#19043));
#4279=EDGE_LOOP('',(#19044,#19045,#19046,#19047));
#4280=EDGE_LOOP('',(#19048,#19049,#19050,#19051));
#4281=EDGE_LOOP('',(#19052,#19053,#19054,#19055));
#4282=EDGE_LOOP('',(#19056,#19057,#19058,#19059));
#4283=EDGE_LOOP('',(#19060,#19061,#19062,#19063));
#4284=EDGE_LOOP('',(#19064,#19065,#19066,#19067));
#4285=EDGE_LOOP('',(#19068,#19069,#19070,#19071));
#4286=EDGE_LOOP('',(#19072,#19073,#19074,#19075));
#4287=EDGE_LOOP('',(#19076,#19077,#19078,#19079));
#4288=EDGE_LOOP('',(#19080,#19081,#19082,#19083));
#4289=EDGE_LOOP('',(#19084,#19085,#19086,#19087));
#4290=EDGE_LOOP('',(#19088,#19089,#19090,#19091));
#4291=EDGE_LOOP('',(#19092,#19093,#19094,#19095));
#4292=EDGE_LOOP('',(#19096,#19097,#19098,#19099));
#4293=EDGE_LOOP('',(#19100,#19101,#19102,#19103));
#4294=EDGE_LOOP('',(#19104,#19105,#19106,#19107));
#4295=EDGE_LOOP('',(#19108,#19109,#19110,#19111));
#4296=EDGE_LOOP('',(#19112,#19113,#19114,#19115));
#4297=EDGE_LOOP('',(#19116,#19117,#19118,#19119));
#4298=EDGE_LOOP('',(#19120,#19121,#19122,#19123));
#4299=EDGE_LOOP('',(#19124,#19125,#19126,#19127));
#4300=EDGE_LOOP('',(#19128,#19129,#19130,#19131));
#4301=EDGE_LOOP('',(#19132,#19133,#19134,#19135));
#4302=EDGE_LOOP('',(#19136,#19137,#19138,#19139));
#4303=EDGE_LOOP('',(#19140,#19141,#19142,#19143));
#4304=EDGE_LOOP('',(#19144,#19145,#19146,#19147));
#4305=EDGE_LOOP('',(#19148,#19149,#19150,#19151));
#4306=EDGE_LOOP('',(#19152));
#4307=EDGE_LOOP('',(#19153,#19154,#19155,#19156));
#4308=EDGE_LOOP('',(#19157,#19158,#19159,#19160));
#4309=EDGE_LOOP('',(#19161,#19162,#19163,#19164));
#4310=EDGE_LOOP('',(#19165,#19166,#19167,#19168));
#4311=EDGE_LOOP('',(#19169));
#4312=EDGE_LOOP('',(#19170,#19171,#19172,#19173));
#4313=EDGE_LOOP('',(#19174));
#4314=EDGE_LOOP('',(#19175,#19176,#19177,#19178));
#4315=EDGE_LOOP('',(#19179,#19180,#19181,#19182));
#4316=EDGE_LOOP('',(#19183,#19184,#19185,#19186));
#4317=EDGE_LOOP('',(#19187,#19188,#19189,#19190,#19191,#19192));
#4318=EDGE_LOOP('',(#19193,#19194,#19195,#19196));
#4319=EDGE_LOOP('',(#19197,#19198,#19199,#19200));
#4320=EDGE_LOOP('',(#19201));
#4321=EDGE_LOOP('',(#19202));
#4322=EDGE_LOOP('',(#19203,#19204,#19205,#19206));
#4323=EDGE_LOOP('',(#19207,#19208,#19209,#19210));
#4324=EDGE_LOOP('',(#19211,#19212,#19213,#19214));
#4325=EDGE_LOOP('',(#19215,#19216,#19217,#19218));
#4326=EDGE_LOOP('',(#19219,#19220,#19221,#19222));
#4327=EDGE_LOOP('',(#19223,#19224,#19225,#19226));
#4328=EDGE_LOOP('',(#19227,#19228,#19229,#19230));
#4329=EDGE_LOOP('',(#19231,#19232,#19233,#19234));
#4330=EDGE_LOOP('',(#19235));
#4331=EDGE_LOOP('',(#19236));
#4332=EDGE_LOOP('',(#19237,#19238,#19239,#19240));
#4333=EDGE_LOOP('',(#19241,#19242,#19243,#19244));
#4334=EDGE_LOOP('',(#19245,#19246,#19247,#19248));
#4335=EDGE_LOOP('',(#19249,#19250,#19251,#19252,#19253,#19254));
#4336=EDGE_LOOP('',(#19255,#19256,#19257,#19258,#19259,#19260));
#4337=EDGE_LOOP('',(#19261));
#4338=EDGE_LOOP('',(#19262,#19263,#19264,#19265));
#4339=EDGE_LOOP('',(#19266,#19267,#19268,#19269));
#4340=EDGE_LOOP('',(#19270,#19271,#19272,#19273));
#4341=EDGE_LOOP('',(#19274,#19275,#19276,#19277));
#4342=EDGE_LOOP('',(#19278,#19279,#19280,#19281,#19282,#19283));
#4343=EDGE_LOOP('',(#19284));
#4344=EDGE_LOOP('',(#19285,#19286,#19287,#19288));
#4345=EDGE_LOOP('',(#19289,#19290,#19291,#19292));
#4346=EDGE_LOOP('',(#19293,#19294,#19295,#19296));
#4347=EDGE_LOOP('',(#19297,#19298,#19299,#19300,#19301,#19302,#19303,#19304,
#19305,#19306,#19307,#19308,#19309,#19310,#19311,#19312,#19313,#19314,#19315,
#19316,#19317,#19318,#19319,#19320,#19321,#19322,#19323,#19324,#19325,#19326,
#19327,#19328,#19329,#19330,#19331,#19332));
#4348=EDGE_LOOP('',(#19333,#19334,#19335,#19336));
#4349=EDGE_LOOP('',(#19337,#19338,#19339,#19340,#19341,#19342,#19343,#19344,
#19345,#19346,#19347,#19348,#19349,#19350,#19351,#19352,#19353,#19354,#19355,
#19356,#19357,#19358,#19359,#19360,#19361,#19362,#19363,#19364,#19365,#19366,
#19367,#19368,#19369,#19370,#19371,#19372,#19373,#19374,#19375,#19376,#19377,
#19378,#19379,#19380,#19381,#19382,#19383,#19384));
#4350=EDGE_LOOP('',(#19385,#19386,#19387,#19388,#19389,#19390,#19391,#19392,
#19393,#19394,#19395,#19396,#19397,#19398,#19399,#19400,#19401,#19402,#19403,
#19404,#19405,#19406,#19407,#19408,#19409,#19410,#19411,#19412,#19413,#19414,
#19415,#19416,#19417,#19418,#19419,#19420,#19421,#19422,#19423,#19424,#19425,
#19426,#19427,#19428));
#4351=EDGE_LOOP('',(#19429,#19430,#19431,#19432,#19433,#19434,#19435,#19436,
#19437,#19438,#19439,#19440,#19441,#19442,#19443,#19444,#19445,#19446,#19447,
#19448,#19449,#19450,#19451,#19452,#19453,#19454,#19455,#19456,#19457,#19458,
#19459,#19460,#19461,#19462,#19463,#19464));
#4352=EDGE_LOOP('',(#19465,#19466,#19467,#19468));
#4353=EDGE_LOOP('',(#19469,#19470,#19471,#19472));
#4354=EDGE_LOOP('',(#19473,#19474,#19475,#19476));
#4355=EDGE_LOOP('',(#19477));
#4356=EDGE_LOOP('',(#19478,#19479,#19480,#19481));
#4357=EDGE_LOOP('',(#19482,#19483,#19484,#19485));
#4358=EDGE_LOOP('',(#19486,#19487,#19488,#19489));
#4359=EDGE_LOOP('',(#19490,#19491,#19492,#19493));
#4360=EDGE_LOOP('',(#19494,#19495,#19496,#19497));
#4361=EDGE_LOOP('',(#19498,#19499,#19500,#19501));
#4362=EDGE_LOOP('',(#19502,#19503,#19504,#19505,#19506,#19507,#19508,#19509,
#19510,#19511));
#4363=EDGE_LOOP('',(#19512,#19513,#19514,#19515));
#4364=EDGE_LOOP('',(#19516,#19517,#19518,#19519));
#4365=EDGE_LOOP('',(#19520,#19521,#19522,#19523));
#4366=EDGE_LOOP('',(#19524,#19525,#19526,#19527));
#4367=EDGE_LOOP('',(#19528,#19529,#19530,#19531));
#4368=EDGE_LOOP('',(#19532,#19533,#19534,#19535));
#4369=EDGE_LOOP('',(#19536,#19537,#19538,#19539));
#4370=EDGE_LOOP('',(#19540,#19541,#19542,#19543));
#4371=EDGE_LOOP('',(#19544,#19545,#19546,#19547));
#4372=EDGE_LOOP('',(#19548,#19549,#19550,#19551));
#4373=EDGE_LOOP('',(#19552,#19553,#19554,#19555));
#4374=EDGE_LOOP('',(#19556,#19557,#19558,#19559));
#4375=EDGE_LOOP('',(#19560,#19561,#19562,#19563));
#4376=EDGE_LOOP('',(#19564,#19565,#19566,#19567));
#4377=EDGE_LOOP('',(#19568,#19569,#19570,#19571));
#4378=EDGE_LOOP('',(#19572,#19573,#19574,#19575));
#4379=EDGE_LOOP('',(#19576,#19577,#19578,#19579));
#4380=EDGE_LOOP('',(#19580,#19581,#19582,#19583));
#4381=EDGE_LOOP('',(#19584,#19585,#19586,#19587));
#4382=EDGE_LOOP('',(#19588,#19589,#19590,#19591));
#4383=EDGE_LOOP('',(#19592,#19593,#19594,#19595));
#4384=EDGE_LOOP('',(#19596,#19597,#19598,#19599));
#4385=EDGE_LOOP('',(#19600,#19601,#19602,#19603));
#4386=EDGE_LOOP('',(#19604,#19605,#19606,#19607));
#4387=EDGE_LOOP('',(#19608,#19609,#19610,#19611));
#4388=EDGE_LOOP('',(#19612,#19613,#19614,#19615));
#4389=EDGE_LOOP('',(#19616,#19617,#19618,#19619));
#4390=EDGE_LOOP('',(#19620));
#4391=EDGE_LOOP('',(#19621,#19622,#19623,#19624));
#4392=EDGE_LOOP('',(#19625,#19626,#19627,#19628));
#4393=EDGE_LOOP('',(#19629,#19630,#19631,#19632,#19633,#19634,#19635,#19636,
#19637,#19638));
#4394=EDGE_LOOP('',(#19639,#19640,#19641,#19642));
#4395=EDGE_LOOP('',(#19643,#19644,#19645,#19646));
#4396=EDGE_LOOP('',(#19647,#19648,#19649,#19650));
#4397=EDGE_LOOP('',(#19651,#19652,#19653,#19654));
#4398=EDGE_LOOP('',(#19655,#19656,#19657,#19658));
#4399=EDGE_LOOP('',(#19659,#19660,#19661,#19662));
#4400=EDGE_LOOP('',(#19663,#19664,#19665,#19666));
#4401=EDGE_LOOP('',(#19667,#19668,#19669,#19670));
#4402=EDGE_LOOP('',(#19671));
#4403=EDGE_LOOP('',(#19672,#19673,#19674,#19675,#19676,#19677,#19678,#19679,
#19680,#19681,#19682,#19683,#19684,#19685,#19686,#19687,#19688,#19689,#19690,
#19691,#19692,#19693,#19694,#19695,#19696,#19697,#19698,#19699,#19700,#19701,
#19702,#19703,#19704,#19705,#19706,#19707,#19708,#19709,#19710,#19711,#19712,
#19713,#19714,#19715,#19716,#19717,#19718,#19719));
#4404=EDGE_LOOP('',(#19720,#19721,#19722,#19723,#19724,#19725,#19726,#19727,
#19728,#19729,#19730,#19731,#19732,#19733,#19734,#19735,#19736,#19737,#19738,
#19739,#19740,#19741,#19742,#19743,#19744,#19745,#19746,#19747,#19748,#19749,
#19750,#19751,#19752,#19753,#19754,#19755,#19756,#19757,#19758,#19759,#19760,
#19761,#19762,#19763));
#4405=EDGE_LOOP('',(#19764,#19765,#19766,#19767));
#4406=EDGE_LOOP('',(#19768,#19769,#19770,#19771));
#4407=EDGE_LOOP('',(#19772,#19773,#19774,#19775));
#4408=EDGE_LOOP('',(#19776,#19777,#19778,#19779));
#4409=EDGE_LOOP('',(#19780,#19781,#19782,#19783,#19784,#19785,#19786));
#4410=EDGE_LOOP('',(#19787,#19788,#19789,#19790,#19791,#19792,#19793));
#4411=EDGE_LOOP('',(#19794,#19795,#19796,#19797,#19798,#19799,#19800));
#4412=EDGE_LOOP('',(#19801,#19802,#19803,#19804,#19805,#19806,#19807));
#5822=LINE('',#37500,#7811);
#5823=LINE('',#37506,#7812);
#5824=LINE('',#37512,#7813);
#5825=LINE('',#37516,#7814);
#5826=LINE('',#37519,#7815);
#5827=LINE('',#37524,#7816);
#5828=LINE('',#37530,#7817);
#5829=LINE('',#37536,#7818);
#5830=LINE('',#37542,#7819);
#5831=LINE('',#37548,#7820);
#5832=LINE('',#37554,#7821);
#5833=LINE('',#37560,#7822);
#5834=LINE('',#37566,#7823);
#5835=LINE('',#37570,#7824);
#5836=LINE('',#37573,#7825);
#5837=LINE('',#37576,#7826);
#5838=LINE('',#37579,#7827);
#5839=LINE('',#37584,#7828);
#5840=LINE('',#37586,#7829);
#5841=LINE('',#37590,#7830);
#5842=LINE('',#37695,#7831);
#5843=LINE('',#37700,#7832);
#5844=LINE('',#37707,#7833);
#5845=LINE('',#37709,#7834);
#5846=LINE('',#37710,#7835);
#5847=LINE('',#37715,#7836);
#5848=LINE('',#37718,#7837);
#5849=LINE('',#37724,#7838);
#5850=LINE('',#37727,#7839);
#5851=LINE('',#37732,#7840);
#5852=LINE('',#37734,#7841);
#5853=LINE('',#37735,#7842);
#5854=LINE('',#37739,#7843);
#5855=LINE('',#37741,#7844);
#5856=LINE('',#37743,#7845);
#5857=LINE('',#37744,#7846);
#5858=LINE('',#37748,#7847);
#5859=LINE('',#37750,#7848);
#5860=LINE('',#37752,#7849);
#5861=LINE('',#37753,#7850);
#5862=LINE('',#37757,#7851);
#5863=LINE('',#37759,#7852);
#5864=LINE('',#37761,#7853);
#5865=LINE('',#37762,#7854);
#5866=LINE('',#37766,#7855);
#5867=LINE('',#37768,#7856);
#5868=LINE('',#37770,#7857);
#5869=LINE('',#37771,#7858);
#5870=LINE('',#37775,#7859);
#5871=LINE('',#37777,#7860);
#5872=LINE('',#37779,#7861);
#5873=LINE('',#37780,#7862);
#5874=LINE('',#37784,#7863);
#5875=LINE('',#37786,#7864);
#5876=LINE('',#37788,#7865);
#5877=LINE('',#37789,#7866);
#5878=LINE('',#37793,#7867);
#5879=LINE('',#37795,#7868);
#5880=LINE('',#37797,#7869);
#5881=LINE('',#37798,#7870);
#5882=LINE('',#37802,#7871);
#5883=LINE('',#37804,#7872);
#5884=LINE('',#37806,#7873);
#5885=LINE('',#37807,#7874);
#5886=LINE('',#37811,#7875);
#5887=LINE('',#37813,#7876);
#5888=LINE('',#37815,#7877);
#5889=LINE('',#37816,#7878);
#5890=LINE('',#37819,#7879);
#5891=LINE('',#37821,#7880);
#5892=LINE('',#37822,#7881);
#5893=LINE('',#37826,#7882);
#5894=LINE('',#37828,#7883);
#5895=LINE('',#37830,#7884);
#5896=LINE('',#37831,#7885);
#5897=LINE('',#37834,#7886);
#5898=LINE('',#37836,#7887);
#5899=LINE('',#37837,#7888);
#5900=LINE('',#37841,#7889);
#5901=LINE('',#37843,#7890);
#5902=LINE('',#37845,#7891);
#5903=LINE('',#37846,#7892);
#5904=LINE('',#37850,#7893);
#5905=LINE('',#37852,#7894);
#5906=LINE('',#37854,#7895);
#5907=LINE('',#37855,#7896);
#5908=LINE('',#37859,#7897);
#5909=LINE('',#37861,#7898);
#5910=LINE('',#37863,#7899);
#5911=LINE('',#37864,#7900);
#5912=LINE('',#37868,#7901);
#5913=LINE('',#37870,#7902);
#5914=LINE('',#37872,#7903);
#5915=LINE('',#37873,#7904);
#5916=LINE('',#37875,#7905);
#5917=LINE('',#37876,#7906);
#5918=LINE('',#37882,#7907);
#5919=LINE('',#37885,#7908);
#5920=LINE('',#37891,#7909);
#5921=LINE('',#37894,#7910);
#5922=LINE('',#37900,#7911);
#5923=LINE('',#37903,#7912);
#5924=LINE('',#37909,#7913);
#5925=LINE('',#37912,#7914);
#5926=LINE('',#37965,#7915);
#5927=LINE('',#37967,#7916);
#5928=LINE('',#37969,#7917);
#5929=LINE('',#37970,#7918);
#5930=LINE('',#37973,#7919);
#5931=LINE('',#37975,#7920);
#5932=LINE('',#37976,#7921);
#5933=LINE('',#37978,#7922);
#5934=LINE('',#37980,#7923);
#5935=LINE('',#37981,#7924);
#5936=LINE('',#37984,#7925);
#5937=LINE('',#37985,#7926);
#5938=LINE('',#37988,#7927);
#5939=LINE('',#37989,#7928);
#5940=LINE('',#37991,#7929);
#5941=LINE('',#37994,#7930);
#5942=LINE('',#37995,#7931);
#5943=LINE('',#37998,#7932);
#5944=LINE('',#37999,#7933);
#5945=LINE('',#38001,#7934);
#5946=LINE('',#38004,#7935);
#5947=LINE('',#38006,#7936);
#5948=LINE('',#38007,#7937);
#5949=LINE('',#38010,#7938);
#5950=LINE('',#38011,#7939);
#5951=LINE('',#38014,#7940);
#5952=LINE('',#38015,#7941);
#5953=LINE('',#38018,#7942);
#5954=LINE('',#38019,#7943);
#5955=LINE('',#38022,#7944);
#5956=LINE('',#38023,#7945);
#5957=LINE('',#38025,#7946);
#5958=LINE('',#38030,#7947);
#5959=LINE('',#38034,#7948);
#5960=LINE('',#38038,#7949);
#5961=LINE('',#38046,#7950);
#5962=LINE('',#38050,#7951);
#5963=LINE('',#38054,#7952);
#5964=LINE('',#38062,#7953);
#5965=LINE('',#38064,#7954);
#5966=LINE('',#38066,#7955);
#5967=LINE('',#38074,#7956);
#5968=LINE('',#38078,#7957);
#5969=LINE('',#38082,#7958);
#5970=LINE('',#38090,#7959);
#5971=LINE('',#38094,#7960);
#5972=LINE('',#38098,#7961);
#5973=LINE('',#38100,#7962);
#5974=LINE('',#38102,#7963);
#5975=LINE('',#38104,#7964);
#5976=LINE('',#38106,#7965);
#5977=LINE('',#38108,#7966);
#5978=LINE('',#38110,#7967);
#5979=LINE('',#38112,#7968);
#5980=LINE('',#38114,#7969);
#5981=LINE('',#38115,#7970);
#5982=LINE('',#38119,#7971);
#5983=LINE('',#38120,#7972);
#5984=LINE('',#38121,#7973);
#5985=LINE('',#38125,#7974);
#5986=LINE('',#38128,#7975);
#5987=LINE('',#38129,#7976);
#5988=LINE('',#38133,#7977);
#5989=LINE('',#38136,#7978);
#5990=LINE('',#38137,#7979);
#5991=LINE('',#38141,#7980);
#5992=LINE('',#38145,#7981);
#5993=LINE('',#38149,#7982);
#5994=LINE('',#38152,#7983);
#5995=LINE('',#38153,#7984);
#5996=LINE('',#38157,#7985);
#5997=LINE('',#38160,#7986);
#5998=LINE('',#38161,#7987);
#5999=LINE('',#38165,#7988);
#6000=LINE('',#38168,#7989);
#6001=LINE('',#38169,#7990);
#6002=LINE('',#38173,#7991);
#6003=LINE('',#38177,#7992);
#6004=LINE('',#38181,#7993);
#6005=LINE('',#38184,#7994);
#6006=LINE('',#38185,#7995);
#6007=LINE('',#38188,#7996);
#6008=LINE('',#38189,#7997);
#6009=LINE('',#38192,#7998);
#6010=LINE('',#38193,#7999);
#6011=LINE('',#38197,#8000);
#6012=LINE('',#38201,#8001);
#6013=LINE('',#38205,#8002);
#6014=LINE('',#38208,#8003);
#6015=LINE('',#38209,#8004);
#6016=LINE('',#38213,#8005);
#6017=LINE('',#38216,#8006);
#6018=LINE('',#38217,#8007);
#6019=LINE('',#38221,#8008);
#6020=LINE('',#38224,#8009);
#6021=LINE('',#38225,#8010);
#6022=LINE('',#38229,#8011);
#6023=LINE('',#38233,#8012);
#6024=LINE('',#38237,#8013);
#6025=LINE('',#38240,#8014);
#6026=LINE('',#38241,#8015);
#6027=LINE('',#38245,#8016);
#6028=LINE('',#38248,#8017);
#6029=LINE('',#38249,#8018);
#6030=LINE('',#38253,#8019);
#6031=LINE('',#38256,#8020);
#6032=LINE('',#38257,#8021);
#6033=LINE('',#38260,#8022);
#6034=LINE('',#38261,#8023);
#6035=LINE('',#38264,#8024);
#6036=LINE('',#38265,#8025);
#6037=LINE('',#38268,#8026);
#6038=LINE('',#38269,#8027);
#6039=LINE('',#38272,#8028);
#6040=LINE('',#38273,#8029);
#6041=LINE('',#38276,#8030);
#6042=LINE('',#38277,#8031);
#6043=LINE('',#38280,#8032);
#6044=LINE('',#38281,#8033);
#6045=LINE('',#38284,#8034);
#6046=LINE('',#38285,#8035);
#6047=LINE('',#38288,#8036);
#6048=LINE('',#38289,#8037);
#6049=LINE('',#38291,#8038);
#6050=LINE('',#38295,#8039);
#6051=LINE('',#38298,#8040);
#6052=LINE('',#38302,#8041);
#6053=LINE('',#38304,#8042);
#6054=LINE('',#38308,#8043);
#6055=LINE('',#38310,#8044);
#6056=LINE('',#38312,#8045);
#6057=LINE('',#38314,#8046);
#6058=LINE('',#38316,#8047);
#6059=LINE('',#38318,#8048);
#6060=LINE('',#38320,#8049);
#6061=LINE('',#38324,#8050);
#6062=LINE('',#38328,#8051);
#6063=LINE('',#38336,#8052);
#6064=LINE('',#38340,#8053);
#6065=LINE('',#38344,#8054);
#6066=LINE('',#38352,#8055);
#6067=LINE('',#38354,#8056);
#6068=LINE('',#38356,#8057);
#6069=LINE('',#38364,#8058);
#6070=LINE('',#38368,#8059);
#6071=LINE('',#38372,#8060);
#6072=LINE('',#38380,#8061);
#6073=LINE('',#38384,#8062);
#6074=LINE('',#38388,#8063);
#6075=LINE('',#38390,#8064);
#6076=LINE('',#38392,#8065);
#6077=LINE('',#38394,#8066);
#6078=LINE('',#38395,#8067);
#6079=LINE('',#38398,#8068);
#6080=LINE('',#38399,#8069);
#6081=LINE('',#38402,#8070);
#6082=LINE('',#38403,#8071);
#6083=LINE('',#38409,#8072);
#6084=LINE('',#38412,#8073);
#6085=LINE('',#38416,#8074);
#6086=LINE('',#38417,#8075);
#6087=LINE('',#38418,#8076);
#6088=LINE('',#38421,#8077);
#6089=LINE('',#38422,#8078);
#6090=LINE('',#38425,#8079);
#6091=LINE('',#38426,#8080);
#6092=LINE('',#38429,#8081);
#6093=LINE('',#38430,#8082);
#6094=LINE('',#38434,#8083);
#6095=LINE('',#38435,#8084);
#6096=LINE('',#38437,#8085);
#6097=LINE('',#38438,#8086);
#6098=LINE('',#38439,#8087);
#6099=LINE('',#38442,#8088);
#6100=LINE('',#38443,#8089);
#6101=LINE('',#38446,#8090);
#6102=LINE('',#38447,#8091);
#6103=LINE('',#38450,#8092);
#6104=LINE('',#38451,#8093);
#6105=LINE('',#38454,#8094);
#6106=LINE('',#38455,#8095);
#6107=LINE('',#38458,#8096);
#6108=LINE('',#38459,#8097);
#6109=LINE('',#38463,#8098);
#6110=LINE('',#38466,#8099);
#6111=LINE('',#38467,#8100);
#6112=LINE('',#38471,#8101);
#6113=LINE('',#38474,#8102);
#6114=LINE('',#38475,#8103);
#6115=LINE('',#38479,#8104);
#6116=LINE('',#38483,#8105);
#6117=LINE('',#38487,#8106);
#6118=LINE('',#38490,#8107);
#6119=LINE('',#38491,#8108);
#6120=LINE('',#38495,#8109);
#6121=LINE('',#38498,#8110);
#6122=LINE('',#38499,#8111);
#6123=LINE('',#38503,#8112);
#6124=LINE('',#38506,#8113);
#6125=LINE('',#38507,#8114);
#6126=LINE('',#38511,#8115);
#6127=LINE('',#38515,#8116);
#6128=LINE('',#38519,#8117);
#6129=LINE('',#38522,#8118);
#6130=LINE('',#38523,#8119);
#6131=LINE('',#38526,#8120);
#6132=LINE('',#38527,#8121);
#6133=LINE('',#38530,#8122);
#6134=LINE('',#38531,#8123);
#6135=LINE('',#38535,#8124);
#6136=LINE('',#38539,#8125);
#6137=LINE('',#38543,#8126);
#6138=LINE('',#38546,#8127);
#6139=LINE('',#38547,#8128);
#6140=LINE('',#38551,#8129);
#6141=LINE('',#38554,#8130);
#6142=LINE('',#38555,#8131);
#6143=LINE('',#38559,#8132);
#6144=LINE('',#38562,#8133);
#6145=LINE('',#38563,#8134);
#6146=LINE('',#38567,#8135);
#6147=LINE('',#38571,#8136);
#6148=LINE('',#38575,#8137);
#6149=LINE('',#38578,#8138);
#6150=LINE('',#38579,#8139);
#6151=LINE('',#38583,#8140);
#6152=LINE('',#38586,#8141);
#6153=LINE('',#38587,#8142);
#6154=LINE('',#38591,#8143);
#6155=LINE('',#38593,#8144);
#6156=LINE('',#38598,#8145);
#6157=LINE('',#38600,#8146);
#6158=LINE('',#38602,#8147);
#6159=LINE('',#38603,#8148);
#6160=LINE('',#38607,#8149);
#6161=LINE('',#38609,#8150);
#6162=LINE('',#38611,#8151);
#6163=LINE('',#38612,#8152);
#6164=LINE('',#38615,#8153);
#6165=LINE('',#38616,#8154);
#6166=LINE('',#38619,#8155);
#6167=LINE('',#38620,#8156);
#6168=LINE('',#38628,#8157);
#6169=LINE('',#38631,#8158);
#6170=LINE('',#38633,#8159);
#6171=LINE('',#38635,#8160);
#6172=LINE('',#38636,#8161);
#6173=LINE('',#38639,#8162);
#6174=LINE('',#38641,#8163);
#6175=LINE('',#38642,#8164);
#6176=LINE('',#38646,#8165);
#6177=LINE('',#38648,#8166);
#6178=LINE('',#38650,#8167);
#6179=LINE('',#38651,#8168);
#6180=LINE('',#38654,#8169);
#6181=LINE('',#38657,#8170);
#6182=LINE('',#38658,#8171);
#6183=LINE('',#38661,#8172);
#6184=LINE('',#38666,#8173);
#6185=LINE('',#38668,#8174);
#6186=LINE('',#38670,#8175);
#6187=LINE('',#38672,#8176);
#6188=LINE('',#38674,#8177);
#6189=LINE('',#38676,#8178);
#6190=LINE('',#38678,#8179);
#6191=LINE('',#38680,#8180);
#6192=LINE('',#38682,#8181);
#6193=LINE('',#38684,#8182);
#6194=LINE('',#38688,#8183);
#6195=LINE('',#38692,#8184);
#6196=LINE('',#38700,#8185);
#6197=LINE('',#38704,#8186);
#6198=LINE('',#38708,#8187);
#6199=LINE('',#38716,#8188);
#6200=LINE('',#38718,#8189);
#6201=LINE('',#38720,#8190);
#6202=LINE('',#38728,#8191);
#6203=LINE('',#38732,#8192);
#6204=LINE('',#38736,#8193);
#6205=LINE('',#38744,#8194);
#6206=LINE('',#38748,#8195);
#6207=LINE('',#38751,#8196);
#6208=LINE('',#38754,#8197);
#6209=LINE('',#38755,#8198);
#6210=LINE('',#38758,#8199);
#6211=LINE('',#38759,#8200);
#6212=LINE('',#38763,#8201);
#6213=LINE('',#38764,#8202);
#6214=LINE('',#38765,#8203);
#6215=LINE('',#38768,#8204);
#6216=LINE('',#38770,#8205);
#6217=LINE('',#38771,#8206);
#6218=LINE('',#38774,#8207);
#6219=LINE('',#38776,#8208);
#6220=LINE('',#38777,#8209);
#6221=LINE('',#38780,#8210);
#6222=LINE('',#38782,#8211);
#6223=LINE('',#38783,#8212);
#6224=LINE('',#38792,#8213);
#6225=LINE('',#38794,#8214);
#6226=LINE('',#38795,#8215);
#6227=LINE('',#38799,#8216);
#6228=LINE('',#38800,#8217);
#6229=LINE('',#38801,#8218);
#6230=LINE('',#38806,#8219);
#6231=LINE('',#38807,#8220);
#6232=LINE('',#38811,#8221);
#6233=LINE('',#38812,#8222);
#6234=LINE('',#38813,#8223);
#6235=LINE('',#38816,#8224);
#6236=LINE('',#38817,#8225);
#6237=LINE('',#38823,#8226);
#6238=LINE('',#38824,#8227);
#6239=LINE('',#38831,#8228);
#6240=LINE('',#38832,#8229);
#6241=LINE('',#38833,#8230);
#6242=LINE('',#38836,#8231);
#6243=LINE('',#38837,#8232);
#6244=LINE('',#38840,#8233);
#6245=LINE('',#38841,#8234);
#6246=LINE('',#38844,#8235);
#6247=LINE('',#38845,#8236);
#6248=LINE('',#38848,#8237);
#6249=LINE('',#38849,#8238);
#6250=LINE('',#38852,#8239);
#6251=LINE('',#38853,#8240);
#6252=LINE('',#38856,#8241);
#6253=LINE('',#38857,#8242);
#6254=LINE('',#38860,#8243);
#6255=LINE('',#38861,#8244);
#6256=LINE('',#38864,#8245);
#6257=LINE('',#38865,#8246);
#6258=LINE('',#38868,#8247);
#6259=LINE('',#38869,#8248);
#6260=LINE('',#38873,#8249);
#6261=LINE('',#38876,#8250);
#6262=LINE('',#38877,#8251);
#6263=LINE('',#38881,#8252);
#6264=LINE('',#38884,#8253);
#6265=LINE('',#38885,#8254);
#6266=LINE('',#38889,#8255);
#6267=LINE('',#38893,#8256);
#6268=LINE('',#38897,#8257);
#6269=LINE('',#38900,#8258);
#6270=LINE('',#38901,#8259);
#6271=LINE('',#38905,#8260);
#6272=LINE('',#38908,#8261);
#6273=LINE('',#38909,#8262);
#6274=LINE('',#38913,#8263);
#6275=LINE('',#38916,#8264);
#6276=LINE('',#38917,#8265);
#6277=LINE('',#38921,#8266);
#6278=LINE('',#38925,#8267);
#6279=LINE('',#38929,#8268);
#6280=LINE('',#38932,#8269);
#6281=LINE('',#38933,#8270);
#6282=LINE('',#38936,#8271);
#6283=LINE('',#38937,#8272);
#6284=LINE('',#38940,#8273);
#6285=LINE('',#38941,#8274);
#6286=LINE('',#38945,#8275);
#6287=LINE('',#38949,#8276);
#6288=LINE('',#38953,#8277);
#6289=LINE('',#38956,#8278);
#6290=LINE('',#38957,#8279);
#6291=LINE('',#38961,#8280);
#6292=LINE('',#38964,#8281);
#6293=LINE('',#38965,#8282);
#6294=LINE('',#38969,#8283);
#6295=LINE('',#38972,#8284);
#6296=LINE('',#38973,#8285);
#6297=LINE('',#38977,#8286);
#6298=LINE('',#38981,#8287);
#6299=LINE('',#38985,#8288);
#6300=LINE('',#38988,#8289);
#6301=LINE('',#38989,#8290);
#6302=LINE('',#38993,#8291);
#6303=LINE('',#38996,#8292);
#6304=LINE('',#38997,#8293);
#6305=LINE('',#39001,#8294);
#6306=LINE('',#39003,#8295);
#6307=LINE('',#39007,#8296);
#6308=LINE('',#39009,#8297);
#6309=LINE('',#39011,#8298);
#6310=LINE('',#39012,#8299);
#6311=LINE('',#39015,#8300);
#6312=LINE('',#39017,#8301);
#6313=LINE('',#39018,#8302);
#6314=LINE('',#39021,#8303);
#6315=LINE('',#39023,#8304);
#6316=LINE('',#39024,#8305);
#6317=LINE('',#39027,#8306);
#6318=LINE('',#39029,#8307);
#6319=LINE('',#39030,#8308);
#6320=LINE('',#39033,#8309);
#6321=LINE('',#39035,#8310);
#6322=LINE('',#39036,#8311);
#6323=LINE('',#39040,#8312);
#6324=LINE('',#39042,#8313);
#6325=LINE('',#39044,#8314);
#6326=LINE('',#39045,#8315);
#6327=LINE('',#39048,#8316);
#6328=LINE('',#39050,#8317);
#6329=LINE('',#39051,#8318);
#6330=LINE('',#39054,#8319);
#6331=LINE('',#39056,#8320);
#6332=LINE('',#39057,#8321);
#6333=LINE('',#39059,#8322);
#6334=LINE('',#39060,#8323);
#6335=LINE('',#39063,#8324);
#6336=LINE('',#39065,#8325);
#6337=LINE('',#39067,#8326);
#6338=LINE('',#39068,#8327);
#6339=LINE('',#39071,#8328);
#6340=LINE('',#39073,#8329);
#6341=LINE('',#39074,#8330);
#6342=LINE('',#39078,#8331);
#6343=LINE('',#39079,#8332);
#6344=LINE('',#39080,#8333);
#6345=LINE('',#39084,#8334);
#6346=LINE('',#39085,#8335);
#6347=LINE('',#39086,#8336);
#6348=LINE('',#39090,#8337);
#6349=LINE('',#39091,#8338);
#6350=LINE('',#39092,#8339);
#6351=LINE('',#39096,#8340);
#6352=LINE('',#39097,#8341);
#6353=LINE('',#39098,#8342);
#6354=LINE('',#39101,#8343);
#6355=LINE('',#39103,#8344);
#6356=LINE('',#39104,#8345);
#6357=LINE('',#39108,#8346);
#6358=LINE('',#39109,#8347);
#6359=LINE('',#39110,#8348);
#6360=LINE('',#39114,#8349);
#6361=LINE('',#39115,#8350);
#6362=LINE('',#39116,#8351);
#6363=LINE('',#39120,#8352);
#6364=LINE('',#39121,#8353);
#6365=LINE('',#39122,#8354);
#6366=LINE('',#39125,#8355);
#6367=LINE('',#39127,#8356);
#6368=LINE('',#39128,#8357);
#6369=LINE('',#39131,#8358);
#6370=LINE('',#39133,#8359);
#6371=LINE('',#39134,#8360);
#6372=LINE('',#39137,#8361);
#6373=LINE('',#39139,#8362);
#6374=LINE('',#39140,#8363);
#6375=LINE('',#39143,#8364);
#6376=LINE('',#39145,#8365);
#6377=LINE('',#39146,#8366);
#6378=LINE('',#39149,#8367);
#6379=LINE('',#39150,#8368);
#6380=LINE('',#39151,#8369);
#6381=LINE('',#39156,#8370);
#6382=LINE('',#39157,#8371);
#6383=LINE('',#39161,#8372);
#6384=LINE('',#39162,#8373);
#6385=LINE('',#39163,#8374);
#6386=LINE('',#39168,#8375);
#6387=LINE('',#39169,#8376);
#6388=LINE('',#39174,#8377);
#6389=LINE('',#39175,#8378);
#6390=LINE('',#39179,#8379);
#6391=LINE('',#39180,#8380);
#6392=LINE('',#39181,#8381);
#6393=LINE('',#39183,#8382);
#6394=LINE('',#39188,#8383);
#6395=LINE('',#39189,#8384);
#6396=LINE('',#39192,#8385);
#6397=LINE('',#39194,#8386);
#6398=LINE('',#39195,#8387);
#6399=LINE('',#39198,#8388);
#6400=LINE('',#39200,#8389);
#6401=LINE('',#39201,#8390);
#6402=LINE('',#39203,#8391);
#6403=LINE('',#39205,#8392);
#6404=LINE('',#39206,#8393);
#6405=LINE('',#39209,#8394);
#6406=LINE('',#39212,#8395);
#6407=LINE('',#39214,#8396);
#6408=LINE('',#39218,#8397);
#6409=LINE('',#39222,#8398);
#6410=LINE('',#39230,#8399);
#6411=LINE('',#39234,#8400);
#6412=LINE('',#39238,#8401);
#6413=LINE('',#39246,#8402);
#6414=LINE('',#39248,#8403);
#6415=LINE('',#39250,#8404);
#6416=LINE('',#39258,#8405);
#6417=LINE('',#39262,#8406);
#6418=LINE('',#39266,#8407);
#6419=LINE('',#39274,#8408);
#6420=LINE('',#39278,#8409);
#6421=LINE('',#39282,#8410);
#6422=LINE('',#39283,#8411);
#6423=LINE('',#39286,#8412);
#6424=LINE('',#39288,#8413);
#6425=LINE('',#39290,#8414);
#6426=LINE('',#39292,#8415);
#6427=LINE('',#39294,#8416);
#6428=LINE('',#39296,#8417);
#6429=LINE('',#39298,#8418);
#6430=LINE('',#39300,#8419);
#6431=LINE('',#39302,#8420);
#6432=LINE('',#39304,#8421);
#6433=LINE('',#39306,#8422);
#6434=LINE('',#39308,#8423);
#6435=LINE('',#39309,#8424);
#6436=LINE('',#39313,#8425);
#6437=LINE('',#39314,#8426);
#6438=LINE('',#39315,#8427);
#6439=LINE('',#39319,#8428);
#6440=LINE('',#39320,#8429);
#6441=LINE('',#39321,#8430);
#6442=LINE('',#39324,#8431);
#6443=LINE('',#39325,#8432);
#6444=LINE('',#39328,#8433);
#6445=LINE('',#39329,#8434);
#6446=LINE('',#39332,#8435);
#6447=LINE('',#39333,#8436);
#6448=LINE('',#39336,#8437);
#6449=LINE('',#39339,#8438);
#6450=LINE('',#39342,#8439);
#6451=LINE('',#39345,#8440);
#6452=LINE('',#39347,#8441);
#6453=LINE('',#39350,#8442);
#6454=LINE('',#39351,#8443);
#6455=LINE('',#39353,#8444);
#6456=LINE('',#39358,#8445);
#6457=LINE('',#39359,#8446);
#6458=LINE('',#39364,#8447);
#6459=LINE('',#39365,#8448);
#6460=LINE('',#39372,#8449);
#6461=LINE('',#39373,#8450);
#6462=LINE('',#39378,#8451);
#6463=LINE('',#39379,#8452);
#6464=LINE('',#39381,#8453);
#6465=LINE('',#39383,#8454);
#6466=LINE('',#39388,#8455);
#6467=LINE('',#39389,#8456);
#6468=LINE('',#39394,#8457);
#6469=LINE('',#39395,#8458);
#6470=LINE('',#39400,#8459);
#6471=LINE('',#39402,#8460);
#6472=LINE('',#39403,#8461);
#6473=LINE('',#39405,#8462);
#6474=LINE('',#39410,#8463);
#6475=LINE('',#39411,#8464);
#6476=LINE('',#39416,#8465);
#6477=LINE('',#39417,#8466);
#6478=LINE('',#39424,#8467);
#6479=LINE('',#39425,#8468);
#6480=LINE('',#39430,#8469);
#6481=LINE('',#39431,#8470);
#6482=LINE('',#39433,#8471);
#6483=LINE('',#39435,#8472);
#6484=LINE('',#39437,#8473);
#6485=LINE('',#39442,#8474);
#6486=LINE('',#39443,#8475);
#6487=LINE('',#39448,#8476);
#6488=LINE('',#39449,#8477);
#6489=LINE('',#39454,#8478);
#6490=LINE('',#39457,#8479);
#6491=LINE('',#39460,#8480);
#6492=LINE('',#39463,#8481);
#6493=LINE('',#39467,#8482);
#6494=LINE('',#39468,#8483);
#6495=LINE('',#39469,#8484);
#6496=LINE('',#39472,#8485);
#6497=LINE('',#39473,#8486);
#6498=LINE('',#39476,#8487);
#6499=LINE('',#39477,#8488);
#6500=LINE('',#39479,#8489);
#6501=LINE('',#39482,#8490);
#6502=LINE('',#39483,#8491);
#6503=LINE('',#39485,#8492);
#6504=LINE('',#39487,#8493);
#6505=LINE('',#39489,#8494);
#6506=LINE('',#39491,#8495);
#6507=LINE('',#39493,#8496);
#6508=LINE('',#39495,#8497);
#6509=LINE('',#39498,#8498);
#6510=LINE('',#39499,#8499);
#6511=LINE('',#39501,#8500);
#6512=LINE('',#39505,#8501);
#6513=LINE('',#39506,#8502);
#6514=LINE('',#39510,#8503);
#6515=LINE('',#39512,#8504);
#7811=VECTOR('',#30203,2.5);
#7812=VECTOR('',#30210,2.5);
#7813=VECTOR('',#30217,3.65);
#7814=VECTOR('',#30222,2.5);
#7815=VECTOR('',#30225,2.5);
#7816=VECTOR('',#30230,3.32349999999999);
#7817=VECTOR('',#30237,3.3235);
#7818=VECTOR('',#30244,3.32349999999999);
#7819=VECTOR('',#30251,3.3235);
#7820=VECTOR('',#30258,2.5);
#7821=VECTOR('',#30265,2.5);
#7822=VECTOR('',#30272,3.65);
#7823=VECTOR('',#30279,0.500000000000006);
#7824=VECTOR('',#30282,1000.);
#7825=VECTOR('',#30285,1000.);
#7826=VECTOR('',#30288,2.5);
#7827=VECTOR('',#30291,2.5);
#7828=VECTOR('',#30296,0.5);
#7829=VECTOR('',#30297,1000.);
#7830=VECTOR('',#30300,1000.);
#7831=VECTOR('',#30311,4.);
#7832=VECTOR('',#30316,4.99995);
#7833=VECTOR('',#30323,1000.);
#7834=VECTOR('',#30324,1000.);
#7835=VECTOR('',#30325,1000.);
#7836=VECTOR('',#30330,1000.);
#7837=VECTOR('',#30333,1000.);
#7838=VECTOR('',#30338,1000.);
#7839=VECTOR('',#30341,1000.);
#7840=VECTOR('',#30346,1000.);
#7841=VECTOR('',#30347,1000.);
#7842=VECTOR('',#30348,1000.);
#7843=VECTOR('',#30351,1000.);
#7844=VECTOR('',#30352,1000.);
#7845=VECTOR('',#30353,1000.);
#7846=VECTOR('',#30354,1000.);
#7847=VECTOR('',#30357,1000.);
#7848=VECTOR('',#30358,1000.);
#7849=VECTOR('',#30359,1000.);
#7850=VECTOR('',#30360,1000.);
#7851=VECTOR('',#30363,1000.);
#7852=VECTOR('',#30364,1000.);
#7853=VECTOR('',#30365,1000.);
#7854=VECTOR('',#30366,1000.);
#7855=VECTOR('',#30369,1000.);
#7856=VECTOR('',#30370,1000.);
#7857=VECTOR('',#30371,1000.);
#7858=VECTOR('',#30372,1000.);
#7859=VECTOR('',#30375,1000.);
#7860=VECTOR('',#30376,1000.);
#7861=VECTOR('',#30377,1000.);
#7862=VECTOR('',#30378,1000.);
#7863=VECTOR('',#30381,1000.);
#7864=VECTOR('',#30382,1000.);
#7865=VECTOR('',#30383,1000.);
#7866=VECTOR('',#30384,1000.);
#7867=VECTOR('',#30387,1000.);
#7868=VECTOR('',#30388,1000.);
#7869=VECTOR('',#30389,1000.);
#7870=VECTOR('',#30390,1000.);
#7871=VECTOR('',#30393,1000.);
#7872=VECTOR('',#30394,1000.);
#7873=VECTOR('',#30395,1000.);
#7874=VECTOR('',#30396,1000.);
#7875=VECTOR('',#30399,1000.);
#7876=VECTOR('',#30400,1000.);
#7877=VECTOR('',#30401,1000.);
#7878=VECTOR('',#30402,1000.);
#7879=VECTOR('',#30405,1000.);
#7880=VECTOR('',#30406,1000.);
#7881=VECTOR('',#30407,1000.);
#7882=VECTOR('',#30410,1000.);
#7883=VECTOR('',#30411,1000.);
#7884=VECTOR('',#30412,1000.);
#7885=VECTOR('',#30413,1000.);
#7886=VECTOR('',#30416,1000.);
#7887=VECTOR('',#30417,1000.);
#7888=VECTOR('',#30418,1000.);
#7889=VECTOR('',#30421,1000.);
#7890=VECTOR('',#30422,1000.);
#7891=VECTOR('',#30423,1000.);
#7892=VECTOR('',#30424,1000.);
#7893=VECTOR('',#30427,1000.);
#7894=VECTOR('',#30428,1000.);
#7895=VECTOR('',#30429,1000.);
#7896=VECTOR('',#30430,1000.);
#7897=VECTOR('',#30433,1000.);
#7898=VECTOR('',#30434,1000.);
#7899=VECTOR('',#30435,1000.);
#7900=VECTOR('',#30436,1000.);
#7901=VECTOR('',#30439,1000.);
#7902=VECTOR('',#30440,1000.);
#7903=VECTOR('',#30441,1000.);
#7904=VECTOR('',#30442,1000.);
#7905=VECTOR('',#30445,1000.);
#7906=VECTOR('',#30446,1000.);
#7907=VECTOR('',#30451,1000.);
#7908=VECTOR('',#30454,1000.);
#7909=VECTOR('',#30459,1000.);
#7910=VECTOR('',#30462,1000.);
#7911=VECTOR('',#30467,1000.);
#7912=VECTOR('',#30470,1000.);
#7913=VECTOR('',#30475,1000.);
#7914=VECTOR('',#30478,1000.);
#7915=VECTOR('',#30579,1000.);
#7916=VECTOR('',#30580,1000.);
#7917=VECTOR('',#30581,1000.);
#7918=VECTOR('',#30582,1000.);
#7919=VECTOR('',#30585,1000.);
#7920=VECTOR('',#30586,1000.);
#7921=VECTOR('',#30587,1000.);
#7922=VECTOR('',#30588,1000.);
#7923=VECTOR('',#30589,1000.);
#7924=VECTOR('',#30590,1000.);
#7925=VECTOR('',#30593,1000.);
#7926=VECTOR('',#30594,1000.);
#7927=VECTOR('',#30597,1000.);
#7928=VECTOR('',#30598,1000.);
#7929=VECTOR('',#30601,1000.);
#7930=VECTOR('',#30604,1000.);
#7931=VECTOR('',#30605,1000.);
#7932=VECTOR('',#30608,1000.);
#7933=VECTOR('',#30609,1000.);
#7934=VECTOR('',#30612,1000.);
#7935=VECTOR('',#30615,1000.);
#7936=VECTOR('',#30616,1000.);
#7937=VECTOR('',#30617,1000.);
#7938=VECTOR('',#30620,1000.);
#7939=VECTOR('',#30621,1000.);
#7940=VECTOR('',#30624,1000.);
#7941=VECTOR('',#30625,1000.);
#7942=VECTOR('',#30628,1000.);
#7943=VECTOR('',#30629,1000.);
#7944=VECTOR('',#30632,1000.);
#7945=VECTOR('',#30633,1000.);
#7946=VECTOR('',#30636,1000.);
#7947=VECTOR('',#30641,1000.);
#7948=VECTOR('',#30644,1000.);
#7949=VECTOR('',#30647,1000.);
#7950=VECTOR('',#30654,1000.);
#7951=VECTOR('',#30657,1000.);
#7952=VECTOR('',#30660,1000.);
#7953=VECTOR('',#30667,1000.);
#7954=VECTOR('',#30668,1000.);
#7955=VECTOR('',#30669,1000.);
#7956=VECTOR('',#30676,1000.);
#7957=VECTOR('',#30679,1000.);
#7958=VECTOR('',#30682,1000.);
#7959=VECTOR('',#30689,1000.);
#7960=VECTOR('',#30692,1000.);
#7961=VECTOR('',#30695,1000.);
#7962=VECTOR('',#30696,1000.);
#7963=VECTOR('',#30697,1000.);
#7964=VECTOR('',#30698,1000.);
#7965=VECTOR('',#30699,1000.);
#7966=VECTOR('',#30700,1000.);
#7967=VECTOR('',#30701,1000.);
#7968=VECTOR('',#30702,1000.);
#7969=VECTOR('',#30703,1000.);
#7970=VECTOR('',#30704,1000.);
#7971=VECTOR('',#30707,1000.);
#7972=VECTOR('',#30708,1000.);
#7973=VECTOR('',#30709,1000.);
#7974=VECTOR('',#30714,1000.);
#7975=VECTOR('',#30717,1000.);
#7976=VECTOR('',#30718,1000.);
#7977=VECTOR('',#30723,1000.);
#7978=VECTOR('',#30726,1000.);
#7979=VECTOR('',#30727,1000.);
#7980=VECTOR('',#30732,1000.);
#7981=VECTOR('',#30737,1000.);
#7982=VECTOR('',#30742,1000.);
#7983=VECTOR('',#30745,1000.);
#7984=VECTOR('',#30746,1000.);
#7985=VECTOR('',#30751,1000.);
#7986=VECTOR('',#30754,1000.);
#7987=VECTOR('',#30755,1000.);
#7988=VECTOR('',#30760,1000.);
#7989=VECTOR('',#30763,1000.);
#7990=VECTOR('',#30764,1000.);
#7991=VECTOR('',#30769,1000.);
#7992=VECTOR('',#30774,1000.);
#7993=VECTOR('',#30779,1000.);
#7994=VECTOR('',#30782,1000.);
#7995=VECTOR('',#30783,1000.);
#7996=VECTOR('',#30786,1000.);
#7997=VECTOR('',#30787,1000.);
#7998=VECTOR('',#30790,1000.);
#7999=VECTOR('',#30791,1000.);
#8000=VECTOR('',#30796,1000.);
#8001=VECTOR('',#30801,1000.);
#8002=VECTOR('',#30806,1000.);
#8003=VECTOR('',#30809,1000.);
#8004=VECTOR('',#30810,1000.);
#8005=VECTOR('',#30815,1000.);
#8006=VECTOR('',#30818,1000.);
#8007=VECTOR('',#30819,1000.);
#8008=VECTOR('',#30824,1000.);
#8009=VECTOR('',#30827,1000.);
#8010=VECTOR('',#30828,1000.);
#8011=VECTOR('',#30833,1000.);
#8012=VECTOR('',#30838,1000.);
#8013=VECTOR('',#30843,1000.);
#8014=VECTOR('',#30846,1000.);
#8015=VECTOR('',#30847,1000.);
#8016=VECTOR('',#30852,1000.);
#8017=VECTOR('',#30855,1000.);
#8018=VECTOR('',#30856,1000.);
#8019=VECTOR('',#30861,1000.);
#8020=VECTOR('',#30864,1000.);
#8021=VECTOR('',#30865,1000.);
#8022=VECTOR('',#30868,1000.);
#8023=VECTOR('',#30869,1000.);
#8024=VECTOR('',#30872,1000.);
#8025=VECTOR('',#30873,1000.);
#8026=VECTOR('',#30876,1000.);
#8027=VECTOR('',#30877,1000.);
#8028=VECTOR('',#30880,1000.);
#8029=VECTOR('',#30881,1000.);
#8030=VECTOR('',#30884,1000.);
#8031=VECTOR('',#30885,1000.);
#8032=VECTOR('',#30888,1000.);
#8033=VECTOR('',#30889,1000.);
#8034=VECTOR('',#30892,1000.);
#8035=VECTOR('',#30893,1000.);
#8036=VECTOR('',#30896,1000.);
#8037=VECTOR('',#30897,1000.);
#8038=VECTOR('',#30900,1000.);
#8039=VECTOR('',#30905,1000.);
#8040=VECTOR('',#30908,1000.);
#8041=VECTOR('',#30911,1000.);
#8042=VECTOR('',#30912,1000.);
#8043=VECTOR('',#30915,1000.);
#8044=VECTOR('',#30916,1000.);
#8045=VECTOR('',#30917,1000.);
#8046=VECTOR('',#30918,1000.);
#8047=VECTOR('',#30919,1000.);
#8048=VECTOR('',#30920,1000.);
#8049=VECTOR('',#30921,1000.);
#8050=VECTOR('',#30924,1000.);
#8051=VECTOR('',#30927,1000.);
#8052=VECTOR('',#30934,1000.);
#8053=VECTOR('',#30937,1000.);
#8054=VECTOR('',#30940,1000.);
#8055=VECTOR('',#30947,1000.);
#8056=VECTOR('',#30948,1000.);
#8057=VECTOR('',#30949,1000.);
#8058=VECTOR('',#30956,1000.);
#8059=VECTOR('',#30959,1000.);
#8060=VECTOR('',#30962,1000.);
#8061=VECTOR('',#30969,1000.);
#8062=VECTOR('',#30972,1000.);
#8063=VECTOR('',#30975,1000.);
#8064=VECTOR('',#30976,1000.);
#8065=VECTOR('',#30977,1000.);
#8066=VECTOR('',#30978,1000.);
#8067=VECTOR('',#30979,1000.);
#8068=VECTOR('',#30982,1000.);
#8069=VECTOR('',#30983,1000.);
#8070=VECTOR('',#30986,1000.);
#8071=VECTOR('',#30987,1000.);
#8072=VECTOR('',#30996,1000.);
#8073=VECTOR('',#30999,1000.);
#8074=VECTOR('',#31002,1000.);
#8075=VECTOR('',#31003,1000.);
#8076=VECTOR('',#31004,1000.);
#8077=VECTOR('',#31007,1000.);
#8078=VECTOR('',#31008,1000.);
#8079=VECTOR('',#31011,1000.);
#8080=VECTOR('',#31012,1000.);
#8081=VECTOR('',#31015,1000.);
#8082=VECTOR('',#31016,1000.);
#8083=VECTOR('',#31019,1000.);
#8084=VECTOR('',#31020,1000.);
#8085=VECTOR('',#31021,1000.);
#8086=VECTOR('',#31022,1000.);
#8087=VECTOR('',#31023,1000.);
#8088=VECTOR('',#31026,1000.);
#8089=VECTOR('',#31027,1000.);
#8090=VECTOR('',#31030,1000.);
#8091=VECTOR('',#31031,1000.);
#8092=VECTOR('',#31034,1000.);
#8093=VECTOR('',#31035,1000.);
#8094=VECTOR('',#31038,1000.);
#8095=VECTOR('',#31039,1000.);
#8096=VECTOR('',#31042,1000.);
#8097=VECTOR('',#31043,1000.);
#8098=VECTOR('',#31048,1000.);
#8099=VECTOR('',#31051,1000.);
#8100=VECTOR('',#31052,1000.);
#8101=VECTOR('',#31057,1000.);
#8102=VECTOR('',#31060,1000.);
#8103=VECTOR('',#31061,1000.);
#8104=VECTOR('',#31066,1000.);
#8105=VECTOR('',#31071,1000.);
#8106=VECTOR('',#31076,1000.);
#8107=VECTOR('',#31079,1000.);
#8108=VECTOR('',#31080,1000.);
#8109=VECTOR('',#31085,1000.);
#8110=VECTOR('',#31088,1000.);
#8111=VECTOR('',#31089,1000.);
#8112=VECTOR('',#31094,1000.);
#8113=VECTOR('',#31097,1000.);
#8114=VECTOR('',#31098,1000.);
#8115=VECTOR('',#31103,1000.);
#8116=VECTOR('',#31108,1000.);
#8117=VECTOR('',#31113,1000.);
#8118=VECTOR('',#31116,1000.);
#8119=VECTOR('',#31117,1000.);
#8120=VECTOR('',#31120,1000.);
#8121=VECTOR('',#31121,1000.);
#8122=VECTOR('',#31124,1000.);
#8123=VECTOR('',#31125,1000.);
#8124=VECTOR('',#31130,1000.);
#8125=VECTOR('',#31135,1000.);
#8126=VECTOR('',#31140,1000.);
#8127=VECTOR('',#31143,1000.);
#8128=VECTOR('',#31144,1000.);
#8129=VECTOR('',#31149,1000.);
#8130=VECTOR('',#31152,1000.);
#8131=VECTOR('',#31153,1000.);
#8132=VECTOR('',#31158,1000.);
#8133=VECTOR('',#31161,1000.);
#8134=VECTOR('',#31162,1000.);
#8135=VECTOR('',#31167,1000.);
#8136=VECTOR('',#31172,1000.);
#8137=VECTOR('',#31177,1000.);
#8138=VECTOR('',#31180,1000.);
#8139=VECTOR('',#31181,1000.);
#8140=VECTOR('',#31186,1000.);
#8141=VECTOR('',#31189,1000.);
#8142=VECTOR('',#31190,1000.);
#8143=VECTOR('',#31195,1000.);
#8144=VECTOR('',#31198,1000.);
#8145=VECTOR('',#31203,1000.);
#8146=VECTOR('',#31204,1000.);
#8147=VECTOR('',#31205,1000.);
#8148=VECTOR('',#31206,1000.);
#8149=VECTOR('',#31209,1000.);
#8150=VECTOR('',#31210,1000.);
#8151=VECTOR('',#31211,1000.);
#8152=VECTOR('',#31212,1000.);
#8153=VECTOR('',#31215,1000.);
#8154=VECTOR('',#31216,1000.);
#8155=VECTOR('',#31219,1000.);
#8156=VECTOR('',#31220,1000.);
#8157=VECTOR('',#31231,1000.);
#8158=VECTOR('',#31234,1000.);
#8159=VECTOR('',#31235,1000.);
#8160=VECTOR('',#31236,1000.);
#8161=VECTOR('',#31237,1000.);
#8162=VECTOR('',#31240,1000.);
#8163=VECTOR('',#31241,1000.);
#8164=VECTOR('',#31242,1000.);
#8165=VECTOR('',#31245,1000.);
#8166=VECTOR('',#31246,1000.);
#8167=VECTOR('',#31247,1000.);
#8168=VECTOR('',#31248,1000.);
#8169=VECTOR('',#31251,1000.);
#8170=VECTOR('',#31254,1000.);
#8171=VECTOR('',#31255,1000.);
#8172=VECTOR('',#31258,1000.);
#8173=VECTOR('',#31263,1000.);
#8174=VECTOR('',#31264,1000.);
#8175=VECTOR('',#31265,1000.);
#8176=VECTOR('',#31266,1000.);
#8177=VECTOR('',#31267,1000.);
#8178=VECTOR('',#31268,1000.);
#8179=VECTOR('',#31269,1000.);
#8180=VECTOR('',#31270,1000.);
#8181=VECTOR('',#31271,1000.);
#8182=VECTOR('',#31272,1000.);
#8183=VECTOR('',#31275,1000.);
#8184=VECTOR('',#31278,1000.);
#8185=VECTOR('',#31285,1000.);
#8186=VECTOR('',#31288,1000.);
#8187=VECTOR('',#31291,1000.);
#8188=VECTOR('',#31298,1000.);
#8189=VECTOR('',#31299,1000.);
#8190=VECTOR('',#31300,1000.);
#8191=VECTOR('',#31307,1000.);
#8192=VECTOR('',#31310,1000.);
#8193=VECTOR('',#31313,1000.);
#8194=VECTOR('',#31320,1000.);
#8195=VECTOR('',#31323,1000.);
#8196=VECTOR('',#31326,1000.);
#8197=VECTOR('',#31329,1000.);
#8198=VECTOR('',#31330,1000.);
#8199=VECTOR('',#31333,1000.);
#8200=VECTOR('',#31334,1000.);
#8201=VECTOR('',#31337,1000.);
#8202=VECTOR('',#31338,1000.);
#8203=VECTOR('',#31339,1000.);
#8204=VECTOR('',#31342,1000.);
#8205=VECTOR('',#31343,1000.);
#8206=VECTOR('',#31344,1000.);
#8207=VECTOR('',#31347,1000.);
#8208=VECTOR('',#31348,1000.);
#8209=VECTOR('',#31349,1000.);
#8210=VECTOR('',#31352,1000.);
#8211=VECTOR('',#31353,1000.);
#8212=VECTOR('',#31354,1000.);
#8213=VECTOR('',#31367,1000.);
#8214=VECTOR('',#31368,1000.);
#8215=VECTOR('',#31369,1000.);
#8216=VECTOR('',#31372,1000.);
#8217=VECTOR('',#31373,1000.);
#8218=VECTOR('',#31374,1000.);
#8219=VECTOR('',#31379,1000.);
#8220=VECTOR('',#31380,1000.);
#8221=VECTOR('',#31383,1000.);
#8222=VECTOR('',#31384,1000.);
#8223=VECTOR('',#31385,1000.);
#8224=VECTOR('',#31388,1000.);
#8225=VECTOR('',#31389,1000.);
#8226=VECTOR('',#31396,1000.);
#8227=VECTOR('',#31397,1000.);
#8228=VECTOR('',#31406,1000.);
#8229=VECTOR('',#31407,1000.);
#8230=VECTOR('',#31408,1000.);
#8231=VECTOR('',#31411,1000.);
#8232=VECTOR('',#31412,1000.);
#8233=VECTOR('',#31415,1000.);
#8234=VECTOR('',#31416,1000.);
#8235=VECTOR('',#31419,1000.);
#8236=VECTOR('',#31420,1000.);
#8237=VECTOR('',#31423,1000.);
#8238=VECTOR('',#31424,1000.);
#8239=VECTOR('',#31427,1000.);
#8240=VECTOR('',#31428,1000.);
#8241=VECTOR('',#31431,1000.);
#8242=VECTOR('',#31432,1000.);
#8243=VECTOR('',#31435,1000.);
#8244=VECTOR('',#31436,1000.);
#8245=VECTOR('',#31439,1000.);
#8246=VECTOR('',#31440,1000.);
#8247=VECTOR('',#31443,1000.);
#8248=VECTOR('',#31444,1000.);
#8249=VECTOR('',#31449,1000.);
#8250=VECTOR('',#31452,1000.);
#8251=VECTOR('',#31453,1000.);
#8252=VECTOR('',#31458,1000.);
#8253=VECTOR('',#31461,1000.);
#8254=VECTOR('',#31462,1000.);
#8255=VECTOR('',#31467,1000.);
#8256=VECTOR('',#31472,1000.);
#8257=VECTOR('',#31477,1000.);
#8258=VECTOR('',#31480,1000.);
#8259=VECTOR('',#31481,1000.);
#8260=VECTOR('',#31486,1000.);
#8261=VECTOR('',#31489,1000.);
#8262=VECTOR('',#31490,1000.);
#8263=VECTOR('',#31495,1000.);
#8264=VECTOR('',#31498,1000.);
#8265=VECTOR('',#31499,1000.);
#8266=VECTOR('',#31504,1000.);
#8267=VECTOR('',#31509,1000.);
#8268=VECTOR('',#31514,1000.);
#8269=VECTOR('',#31517,1000.);
#8270=VECTOR('',#31518,1000.);
#8271=VECTOR('',#31521,1000.);
#8272=VECTOR('',#31522,1000.);
#8273=VECTOR('',#31525,1000.);
#8274=VECTOR('',#31526,1000.);
#8275=VECTOR('',#31531,1000.);
#8276=VECTOR('',#31536,1000.);
#8277=VECTOR('',#31541,1000.);
#8278=VECTOR('',#31544,1000.);
#8279=VECTOR('',#31545,1000.);
#8280=VECTOR('',#31550,1000.);
#8281=VECTOR('',#31553,1000.);
#8282=VECTOR('',#31554,1000.);
#8283=VECTOR('',#31559,1000.);
#8284=VECTOR('',#31562,1000.);
#8285=VECTOR('',#31563,1000.);
#8286=VECTOR('',#31568,1000.);
#8287=VECTOR('',#31573,1000.);
#8288=VECTOR('',#31578,1000.);
#8289=VECTOR('',#31581,1000.);
#8290=VECTOR('',#31582,1000.);
#8291=VECTOR('',#31587,1000.);
#8292=VECTOR('',#31590,1000.);
#8293=VECTOR('',#31591,1000.);
#8294=VECTOR('',#31596,1000.);
#8295=VECTOR('',#31599,1000.);
#8296=VECTOR('',#31602,1000.);
#8297=VECTOR('',#31603,1000.);
#8298=VECTOR('',#31604,1000.);
#8299=VECTOR('',#31605,1000.);
#8300=VECTOR('',#31608,1000.);
#8301=VECTOR('',#31609,1000.);
#8302=VECTOR('',#31610,1000.);
#8303=VECTOR('',#31613,1000.);
#8304=VECTOR('',#31614,1000.);
#8305=VECTOR('',#31615,1000.);
#8306=VECTOR('',#31618,1000.);
#8307=VECTOR('',#31619,1000.);
#8308=VECTOR('',#31620,1000.);
#8309=VECTOR('',#31623,1000.);
#8310=VECTOR('',#31624,1000.);
#8311=VECTOR('',#31625,1000.);
#8312=VECTOR('',#31628,1000.);
#8313=VECTOR('',#31629,1000.);
#8314=VECTOR('',#31630,1000.);
#8315=VECTOR('',#31631,1000.);
#8316=VECTOR('',#31634,1000.);
#8317=VECTOR('',#31635,1000.);
#8318=VECTOR('',#31636,1000.);
#8319=VECTOR('',#31639,1000.);
#8320=VECTOR('',#31640,1000.);
#8321=VECTOR('',#31641,1000.);
#8322=VECTOR('',#31644,1000.);
#8323=VECTOR('',#31645,1000.);
#8324=VECTOR('',#31648,1000.);
#8325=VECTOR('',#31649,1000.);
#8326=VECTOR('',#31650,1000.);
#8327=VECTOR('',#31651,1000.);
#8328=VECTOR('',#31654,1000.);
#8329=VECTOR('',#31655,1000.);
#8330=VECTOR('',#31656,1000.);
#8331=VECTOR('',#31659,1000.);
#8332=VECTOR('',#31660,1000.);
#8333=VECTOR('',#31661,1000.);
#8334=VECTOR('',#31664,1000.);
#8335=VECTOR('',#31665,1000.);
#8336=VECTOR('',#31666,1000.);
#8337=VECTOR('',#31669,1000.);
#8338=VECTOR('',#31670,1000.);
#8339=VECTOR('',#31671,1000.);
#8340=VECTOR('',#31674,1000.);
#8341=VECTOR('',#31675,1000.);
#8342=VECTOR('',#31676,1000.);
#8343=VECTOR('',#31679,1000.);
#8344=VECTOR('',#31680,1000.);
#8345=VECTOR('',#31681,1000.);
#8346=VECTOR('',#31684,1000.);
#8347=VECTOR('',#31685,1000.);
#8348=VECTOR('',#31686,1000.);
#8349=VECTOR('',#31689,1000.);
#8350=VECTOR('',#31690,1000.);
#8351=VECTOR('',#31691,1000.);
#8352=VECTOR('',#31694,1000.);
#8353=VECTOR('',#31695,1000.);
#8354=VECTOR('',#31696,1000.);
#8355=VECTOR('',#31699,1000.);
#8356=VECTOR('',#31700,1000.);
#8357=VECTOR('',#31701,1000.);
#8358=VECTOR('',#31704,1000.);
#8359=VECTOR('',#31705,1000.);
#8360=VECTOR('',#31706,1000.);
#8361=VECTOR('',#31709,1000.);
#8362=VECTOR('',#31710,1000.);
#8363=VECTOR('',#31711,1000.);
#8364=VECTOR('',#31714,1000.);
#8365=VECTOR('',#31715,1000.);
#8366=VECTOR('',#31716,1000.);
#8367=VECTOR('',#31719,1000.);
#8368=VECTOR('',#31720,1000.);
#8369=VECTOR('',#31721,1000.);
#8370=VECTOR('',#31726,1000.);
#8371=VECTOR('',#31727,1000.);
#8372=VECTOR('',#31730,1000.);
#8373=VECTOR('',#31731,1000.);
#8374=VECTOR('',#31732,1000.);
#8375=VECTOR('',#31737,1000.);
#8376=VECTOR('',#31738,1000.);
#8377=VECTOR('',#31743,1000.);
#8378=VECTOR('',#31744,1000.);
#8379=VECTOR('',#31747,1000.);
#8380=VECTOR('',#31748,1000.);
#8381=VECTOR('',#31749,1000.);
#8382=VECTOR('',#31752,1000.);
#8383=VECTOR('',#31759,1000.);
#8384=VECTOR('',#31760,1000.);
#8385=VECTOR('',#31763,1000.);
#8386=VECTOR('',#31764,1000.);
#8387=VECTOR('',#31765,1000.);
#8388=VECTOR('',#31768,1000.);
#8389=VECTOR('',#31769,1000.);
#8390=VECTOR('',#31770,1000.);
#8391=VECTOR('',#31773,1000.);
#8392=VECTOR('',#31774,1000.);
#8393=VECTOR('',#31775,1000.);
#8394=VECTOR('',#31780,1000.);
#8395=VECTOR('',#31783,1000.);
#8396=VECTOR('',#31784,1000.);
#8397=VECTOR('',#31787,1000.);
#8398=VECTOR('',#31790,1000.);
#8399=VECTOR('',#31797,1000.);
#8400=VECTOR('',#31800,1000.);
#8401=VECTOR('',#31803,1000.);
#8402=VECTOR('',#31810,1000.);
#8403=VECTOR('',#31811,1000.);
#8404=VECTOR('',#31812,1000.);
#8405=VECTOR('',#31819,1000.);
#8406=VECTOR('',#31822,1000.);
#8407=VECTOR('',#31825,1000.);
#8408=VECTOR('',#31832,1000.);
#8409=VECTOR('',#31835,1000.);
#8410=VECTOR('',#31838,1000.);
#8411=VECTOR('',#31839,1000.);
#8412=VECTOR('',#31842,1000.);
#8413=VECTOR('',#31843,1000.);
#8414=VECTOR('',#31844,1000.);
#8415=VECTOR('',#31845,1000.);
#8416=VECTOR('',#31846,1000.);
#8417=VECTOR('',#31847,1000.);
#8418=VECTOR('',#31848,1000.);
#8419=VECTOR('',#31849,1000.);
#8420=VECTOR('',#31850,1000.);
#8421=VECTOR('',#31851,1000.);
#8422=VECTOR('',#31852,1000.);
#8423=VECTOR('',#31853,1000.);
#8424=VECTOR('',#31854,1000.);
#8425=VECTOR('',#31857,1000.);
#8426=VECTOR('',#31858,1000.);
#8427=VECTOR('',#31859,1000.);
#8428=VECTOR('',#31862,1000.);
#8429=VECTOR('',#31863,1000.);
#8430=VECTOR('',#31864,1000.);
#8431=VECTOR('',#31867,1000.);
#8432=VECTOR('',#31868,1000.);
#8433=VECTOR('',#31871,1000.);
#8434=VECTOR('',#31872,1000.);
#8435=VECTOR('',#31875,1000.);
#8436=VECTOR('',#31876,1000.);
#8437=VECTOR('',#31879,1000.);
#8438=VECTOR('',#31882,1000.);
#8439=VECTOR('',#31885,1000.);
#8440=VECTOR('',#31888,1000.);
#8441=VECTOR('',#31891,1000.);
#8442=VECTOR('',#31894,1000.);
#8443=VECTOR('',#31895,1000.);
#8444=VECTOR('',#31898,1000.);
#8445=VECTOR('',#31903,1000.);
#8446=VECTOR('',#31904,1000.);
#8447=VECTOR('',#31909,1000.);
#8448=VECTOR('',#31910,1000.);
#8449=VECTOR('',#31919,1000.);
#8450=VECTOR('',#31920,1000.);
#8451=VECTOR('',#31925,1000.);
#8452=VECTOR('',#31926,1000.);
#8453=VECTOR('',#31929,1000.);
#8454=VECTOR('',#31932,1000.);
#8455=VECTOR('',#31937,1000.);
#8456=VECTOR('',#31938,1000.);
#8457=VECTOR('',#31943,1000.);
#8458=VECTOR('',#31944,1000.);
#8459=VECTOR('',#31951,1000.);
#8460=VECTOR('',#31952,1000.);
#8461=VECTOR('',#31953,1000.);
#8462=VECTOR('',#31956,1000.);
#8463=VECTOR('',#31961,1000.);
#8464=VECTOR('',#31962,1000.);
#8465=VECTOR('',#31967,1000.);
#8466=VECTOR('',#31968,1000.);
#8467=VECTOR('',#31977,1000.);
#8468=VECTOR('',#31978,1000.);
#8469=VECTOR('',#31983,1000.);
#8470=VECTOR('',#31984,1000.);
#8471=VECTOR('',#31987,1000.);
#8472=VECTOR('',#31990,1000.);
#8473=VECTOR('',#31993,1000.);
#8474=VECTOR('',#31998,1000.);
#8475=VECTOR('',#31999,1000.);
#8476=VECTOR('',#32004,1000.);
#8477=VECTOR('',#32005,1000.);
#8478=VECTOR('',#32012,1000.);
#8479=VECTOR('',#32015,1000.);
#8480=VECTOR('',#32018,1000.);
#8481=VECTOR('',#32021,1000.);
#8482=VECTOR('',#32024,1000.);
#8483=VECTOR('',#32025,1000.);
#8484=VECTOR('',#32026,1000.);
#8485=VECTOR('',#32029,1000.);
#8486=VECTOR('',#32030,1000.);
#8487=VECTOR('',#32033,1000.);
#8488=VECTOR('',#32034,1000.);
#8489=VECTOR('',#32037,1000.);
#8490=VECTOR('',#32040,1000.);
#8491=VECTOR('',#32041,1000.);
#8492=VECTOR('',#32044,1000.);
#8493=VECTOR('',#32047,1000.);
#8494=VECTOR('',#32050,1000.);
#8495=VECTOR('',#32053,1000.);
#8496=VECTOR('',#32056,1000.);
#8497=VECTOR('',#32059,1000.);
#8498=VECTOR('',#32062,1000.);
#8499=VECTOR('',#32063,1000.);
#8500=VECTOR('',#32066,1000.);
#8501=VECTOR('',#32071,1000.);
#8502=VECTOR('',#32072,1000.);
#8503=VECTOR('',#32077,1000.);
#8504=VECTOR('',#32080,1000.);
#9707=CIRCLE('',#26594,2.5);
#9708=CIRCLE('',#26595,2.5);
#9709=CIRCLE('',#26597,2.5);
#9710=CIRCLE('',#26598,2.5);
#9711=CIRCLE('',#26600,3.65);
#9712=CIRCLE('',#26601,3.65);
#9713=CIRCLE('',#26605,3.3235);
#9714=CIRCLE('',#26606,3.3235);
#9715=CIRCLE('',#26608,3.3235);
#9716=CIRCLE('',#26609,3.3235);
#9717=CIRCLE('',#26611,3.3235);
#9718=CIRCLE('',#26612,3.32349999999999);
#9719=CIRCLE('',#26614,3.32349999999999);
#9720=CIRCLE('',#26615,3.3235);
#9721=CIRCLE('',#26617,2.5);
#9722=CIRCLE('',#26618,2.5);
#9723=CIRCLE('',#26620,2.5);
#9724=CIRCLE('',#26621,2.5);
#9725=CIRCLE('',#26623,3.65);
#9726=CIRCLE('',#26624,3.65);
#9727=CIRCLE('',#26626,0.500000000000004);
#9728=CIRCLE('',#26627,0.500000000000004);
#9729=CIRCLE('',#26628,0.500000000000006);
#9730=CIRCLE('',#26632,0.5);
#9731=CIRCLE('',#26633,0.5);
#9732=CIRCLE('',#26634,0.5);
#9733=CIRCLE('',#26635,4.);
#9734=CIRCLE('',#26636,4.);
#9735=CIRCLE('',#26638,4.);
#9736=CIRCLE('',#26640,4.99995);
#9737=CIRCLE('',#26641,4.99995);
#9738=CIRCLE('',#26670,2.3);
#9739=CIRCLE('',#26671,2.3);
#9740=CIRCLE('',#26673,2.3);
#9741=CIRCLE('',#26674,2.3);
#9742=CIRCLE('',#26676,2.3);
#9743=CIRCLE('',#26677,2.3);
#9744=CIRCLE('',#26679,2.3);
#9745=CIRCLE('',#26680,2.3);
#9746=CIRCLE('',#26682,0.5);
#9747=CIRCLE('',#26683,0.5);
#9748=CIRCLE('',#26685,0.5);
#9749=CIRCLE('',#26686,0.5);
#9750=CIRCLE('',#26688,0.5);
#9751=CIRCLE('',#26689,0.5);
#9752=CIRCLE('',#26691,0.5);
#9753=CIRCLE('',#26692,0.5);
#9754=CIRCLE('',#26694,0.5);
#9755=CIRCLE('',#26695,0.5);
#9756=CIRCLE('',#26697,0.5);
#9757=CIRCLE('',#26698,0.5);
#9758=CIRCLE('',#26700,0.5);
#9759=CIRCLE('',#26701,0.5);
#9760=CIRCLE('',#26703,0.5);
#9761=CIRCLE('',#26704,0.5);
#9762=CIRCLE('',#26706,0.5);
#9763=CIRCLE('',#26707,0.5);
#9764=CIRCLE('',#26709,0.5);
#9765=CIRCLE('',#26710,0.5);
#9766=CIRCLE('',#26712,0.5);
#9767=CIRCLE('',#26713,0.5);
#9768=CIRCLE('',#26715,0.499999999999999);
#9769=CIRCLE('',#26716,0.5);
#9770=CIRCLE('',#26718,0.5);
#9771=CIRCLE('',#26719,0.5);
#9772=CIRCLE('',#26721,0.5);
#9773=CIRCLE('',#26722,0.5);
#9774=CIRCLE('',#26724,0.5);
#9775=CIRCLE('',#26725,0.5);
#9776=CIRCLE('',#26727,0.500000000000001);
#9777=CIRCLE('',#26728,0.5);
#9778=CIRCLE('',#26746,0.450000000000001);
#9779=CIRCLE('',#26747,0.450000000000001);
#9780=CIRCLE('',#26748,0.55);
#9781=CIRCLE('',#26749,2.25);
#9782=CIRCLE('',#26750,0.549999999999998);
#9783=CIRCLE('',#26751,0.55);
#9784=CIRCLE('',#26752,0.55);
#9785=CIRCLE('',#26753,0.55);
#9786=CIRCLE('',#26754,2.25);
#9787=CIRCLE('',#26755,0.55);
#9788=CIRCLE('',#26756,0.550000000000001);
#9789=CIRCLE('',#26757,2.25);
#9790=CIRCLE('',#26758,0.550000000000002);
#9791=CIRCLE('',#26759,0.55);
#9792=CIRCLE('',#26760,0.55);
#9793=CIRCLE('',#26761,0.55);
#9794=CIRCLE('',#26762,2.25);
#9795=CIRCLE('',#26763,0.55);
#9796=CIRCLE('',#26764,0.450000000000001);
#9797=CIRCLE('',#26765,0.450000000000001);
#9798=CIRCLE('',#26768,0.450000000000001);
#9799=CIRCLE('',#26771,0.450000000000001);
#9800=CIRCLE('',#26774,0.55);
#9801=CIRCLE('',#26776,2.25);
#9802=CIRCLE('',#26778,0.549999999999998);
#9803=CIRCLE('',#26781,0.55);
#9804=CIRCLE('',#26784,0.55);
#9805=CIRCLE('',#26787,0.55);
#9806=CIRCLE('',#26789,2.25);
#9807=CIRCLE('',#26791,0.55);
#9808=CIRCLE('',#26796,0.550000000000001);
#9809=CIRCLE('',#26798,2.25);
#9810=CIRCLE('',#26800,0.550000000000002);
#9811=CIRCLE('',#26803,0.55);
#9812=CIRCLE('',#26806,0.55);
#9813=CIRCLE('',#26809,0.55);
#9814=CIRCLE('',#26811,2.25);
#9815=CIRCLE('',#26813,0.55);
#9816=CIRCLE('',#26816,0.450000000000001);
#9817=CIRCLE('',#26819,0.450000000000001);
#9818=CIRCLE('',#26832,0.5);
#9819=CIRCLE('',#26834,4.99995);
#9820=CIRCLE('',#26835,0.5);
#9821=CIRCLE('',#26836,0.5);
#9822=CIRCLE('',#26837,0.5);
#9823=CIRCLE('',#26838,2.3);
#9824=CIRCLE('',#26839,0.5);
#9825=CIRCLE('',#26840,0.5);
#9826=CIRCLE('',#26841,0.5);
#9827=CIRCLE('',#26842,0.5);
#9828=CIRCLE('',#26843,2.3);
#9829=CIRCLE('',#26844,0.5);
#9830=CIRCLE('',#26845,0.5);
#9831=CIRCLE('',#26846,2.3);
#9832=CIRCLE('',#26847,0.5);
#9833=CIRCLE('',#26848,0.5);
#9834=CIRCLE('',#26849,0.5);
#9835=CIRCLE('',#26850,0.5);
#9836=CIRCLE('',#26851,2.3);
#9837=CIRCLE('',#26852,0.5);
#9838=CIRCLE('',#26853,0.5);
#9839=CIRCLE('',#26854,0.5);
#9840=CIRCLE('',#26858,0.5);
#9841=CIRCLE('',#26861,0.500000000000006);
#9842=CIRCLE('',#26873,0.5);
#9843=CIRCLE('',#26876,0.5);
#9844=CIRCLE('',#26879,0.5);
#9845=CIRCLE('',#26881,2.3);
#9846=CIRCLE('',#26883,0.499999999999999);
#9847=CIRCLE('',#26886,0.5);
#9848=CIRCLE('',#26889,0.5);
#9849=CIRCLE('',#26892,0.5);
#9850=CIRCLE('',#26894,2.3);
#9851=CIRCLE('',#26896,0.500000000000001);
#9852=CIRCLE('',#26901,0.5);
#9853=CIRCLE('',#26903,2.3);
#9854=CIRCLE('',#26905,0.5);
#9855=CIRCLE('',#26908,0.5);
#9856=CIRCLE('',#26911,0.5);
#9857=CIRCLE('',#26914,0.5);
#9858=CIRCLE('',#26916,2.3);
#9859=CIRCLE('',#26918,0.5);
#9860=CIRCLE('',#26921,0.5);
#9861=CIRCLE('',#26924,0.5);
#9862=CIRCLE('',#26932,0.500000000000006);
#9863=CIRCLE('',#26934,2.);
#9864=CIRCLE('',#26935,2.);
#9865=CIRCLE('',#26940,2.);
#9866=CIRCLE('',#26942,2.);
#9867=CIRCLE('',#26944,0.450000000000001);
#9868=CIRCLE('',#26945,0.450000000000001);
#9869=CIRCLE('',#26946,0.55);
#9870=CIRCLE('',#26947,2.25);
#9871=CIRCLE('',#26948,0.55);
#9872=CIRCLE('',#26949,0.55);
#9873=CIRCLE('',#26950,0.55);
#9874=CIRCLE('',#26951,0.550000000000002);
#9875=CIRCLE('',#26952,2.25);
#9876=CIRCLE('',#26953,0.550000000000001);
#9877=CIRCLE('',#26954,0.55);
#9878=CIRCLE('',#26955,2.25);
#9879=CIRCLE('',#26956,0.55);
#9880=CIRCLE('',#26957,0.55);
#9881=CIRCLE('',#26958,0.55);
#9882=CIRCLE('',#26959,0.549999999999998);
#9883=CIRCLE('',#26960,2.25);
#9884=CIRCLE('',#26961,0.55);
#9885=CIRCLE('',#26962,0.450000000000001);
#9886=CIRCLE('',#26963,0.450000000000001);
#9887=CIRCLE('',#26975,5.5);
#9888=CIRCLE('',#26981,5.5);
#9889=CIRCLE('',#26998,0.450000000000001);
#9890=CIRCLE('',#27001,0.450000000000001);
#9891=CIRCLE('',#27004,0.55);
#9892=CIRCLE('',#27006,2.25);
#9893=CIRCLE('',#27008,0.55);
#9894=CIRCLE('',#27011,0.55);
#9895=CIRCLE('',#27014,0.55);
#9896=CIRCLE('',#27017,0.550000000000002);
#9897=CIRCLE('',#27019,2.25);
#9898=CIRCLE('',#27021,0.550000000000001);
#9899=CIRCLE('',#27026,0.55);
#9900=CIRCLE('',#27028,2.25);
#9901=CIRCLE('',#27030,0.55);
#9902=CIRCLE('',#27033,0.55);
#9903=CIRCLE('',#27036,0.55);
#9904=CIRCLE('',#27039,0.549999999999998);
#9905=CIRCLE('',#27041,2.25);
#9906=CIRCLE('',#27043,0.55);
#9907=CIRCLE('',#27046,0.450000000000001);
#9908=CIRCLE('',#27049,0.450000000000001);
#9909=CIRCLE('',#27076,5.50000000000001);
#9910=CIRCLE('',#27084,5.49999999999999);
#9911=CIRCLE('',#27093,0.5);
#9912=CIRCLE('',#27094,0.5);
#9913=CIRCLE('',#27095,0.5);
#9914=CIRCLE('',#27096,2.3);
#9915=CIRCLE('',#27097,0.499999999999999);
#9916=CIRCLE('',#27098,0.5);
#9917=CIRCLE('',#27099,0.5);
#9918=CIRCLE('',#27100,0.5);
#9919=CIRCLE('',#27101,2.3);
#9920=CIRCLE('',#27102,0.500000000000001);
#9921=CIRCLE('',#27103,0.5);
#9922=CIRCLE('',#27104,2.3);
#9923=CIRCLE('',#27105,0.5);
#9924=CIRCLE('',#27106,0.5);
#9925=CIRCLE('',#27107,0.5);
#9926=CIRCLE('',#27108,0.5);
#9927=CIRCLE('',#27109,2.3);
#9928=CIRCLE('',#27110,0.5);
#9929=CIRCLE('',#27111,0.5);
#9930=CIRCLE('',#27112,0.5);
#9931=CIRCLE('',#27120,0.5);
#9932=CIRCLE('',#27122,0.5);
#9933=CIRCLE('',#27127,0.5);
#9934=CIRCLE('',#27129,0.5);
#9935=CIRCLE('',#27131,2.3);
#9936=CIRCLE('',#27133,0.5);
#9937=CIRCLE('',#27135,0.5);
#9938=CIRCLE('',#27139,0.5);
#9939=CIRCLE('',#27141,0.5);
#9940=CIRCLE('',#27143,2.3);
#9941=CIRCLE('',#27147,0.500000000000001);
#9942=CIRCLE('',#27149,0.5);
#9943=CIRCLE('',#27151,2.3);
#9944=CIRCLE('',#27153,0.5);
#9945=CIRCLE('',#27155,0.5);
#9946=CIRCLE('',#27160,0.499999999999999);
#9947=CIRCLE('',#27162,0.5);
#9948=CIRCLE('',#27164,2.3);
#9949=CIRCLE('',#27166,0.5);
#9950=CIRCLE('',#27168,0.5);
#9951=CIRCLE('',#27185,4.99995);
#11068=VERTEX_POINT('',#37497);
#11069=VERTEX_POINT('',#37499);
#11070=VERTEX_POINT('',#37503);
#11071=VERTEX_POINT('',#37505);
#11072=VERTEX_POINT('',#37509);
#11073=VERTEX_POINT('',#37511);
#11074=VERTEX_POINT('',#37515);
#11075=VERTEX_POINT('',#37518);
#11076=VERTEX_POINT('',#37521);
#11077=VERTEX_POINT('',#37523);
#11078=VERTEX_POINT('',#37527);
#11079=VERTEX_POINT('',#37529);
#11080=VERTEX_POINT('',#37533);
#11081=VERTEX_POINT('',#37535);
#11082=VERTEX_POINT('',#37539);
#11083=VERTEX_POINT('',#37541);
#11084=VERTEX_POINT('',#37545);
#11085=VERTEX_POINT('',#37547);
#11086=VERTEX_POINT('',#37551);
#11087=VERTEX_POINT('',#37553);
#11088=VERTEX_POINT('',#37557);
#11089=VERTEX_POINT('',#37559);
#11090=VERTEX_POINT('',#37563);
#11091=VERTEX_POINT('',#37565);
#11092=VERTEX_POINT('',#37567);
#11093=VERTEX_POINT('',#37569);
#11094=VERTEX_POINT('',#37571);
#11095=VERTEX_POINT('',#37575);
#11096=VERTEX_POINT('',#37578);
#11097=VERTEX_POINT('',#37581);
#11098=VERTEX_POINT('',#37583);
#11099=VERTEX_POINT('',#37585);
#11100=VERTEX_POINT('',#37587);
#11101=VERTEX_POINT('',#37589);
#11102=VERTEX_POINT('',#37619);
#11103=VERTEX_POINT('',#37620);
#11104=VERTEX_POINT('',#37631);
#11105=VERTEX_POINT('',#37642);
#11106=VERTEX_POINT('',#37653);
#11107=VERTEX_POINT('',#37657);
#11108=VERTEX_POINT('',#37660);
#11109=VERTEX_POINT('',#37671);
#11110=VERTEX_POINT('',#37693);
#11111=VERTEX_POINT('',#37697);
#11112=VERTEX_POINT('',#37699);
#11113=VERTEX_POINT('',#37703);
#11114=VERTEX_POINT('',#37704);
#11115=VERTEX_POINT('',#37706);
#11116=VERTEX_POINT('',#37708);
#11117=VERTEX_POINT('',#37712);
#11118=VERTEX_POINT('',#37714);
#11119=VERTEX_POINT('',#37716);
#11120=VERTEX_POINT('',#37720);
#11121=VERTEX_POINT('',#37721);
#11122=VERTEX_POINT('',#37723);
#11123=VERTEX_POINT('',#37725);
#11124=VERTEX_POINT('',#37729);
#11125=VERTEX_POINT('',#37731);
#11126=VERTEX_POINT('',#37733);
#11127=VERTEX_POINT('',#37737);
#11128=VERTEX_POINT('',#37738);
#11129=VERTEX_POINT('',#37740);
#11130=VERTEX_POINT('',#37742);
#11131=VERTEX_POINT('',#37746);
#11132=VERTEX_POINT('',#37747);
#11133=VERTEX_POINT('',#37749);
#11134=VERTEX_POINT('',#37751);
#11135=VERTEX_POINT('',#37755);
#11136=VERTEX_POINT('',#37756);
#11137=VERTEX_POINT('',#37758);
#11138=VERTEX_POINT('',#37760);
#11139=VERTEX_POINT('',#37764);
#11140=VERTEX_POINT('',#37765);
#11141=VERTEX_POINT('',#37767);
#11142=VERTEX_POINT('',#37769);
#11143=VERTEX_POINT('',#37773);
#11144=VERTEX_POINT('',#37774);
#11145=VERTEX_POINT('',#37776);
#11146=VERTEX_POINT('',#37778);
#11147=VERTEX_POINT('',#37782);
#11148=VERTEX_POINT('',#37783);
#11149=VERTEX_POINT('',#37785);
#11150=VERTEX_POINT('',#37787);
#11151=VERTEX_POINT('',#37791);
#11152=VERTEX_POINT('',#37792);
#11153=VERTEX_POINT('',#37794);
#11154=VERTEX_POINT('',#37796);
#11155=VERTEX_POINT('',#37800);
#11156=VERTEX_POINT('',#37801);
#11157=VERTEX_POINT('',#37803);
#11158=VERTEX_POINT('',#37805);
#11159=VERTEX_POINT('',#37809);
#11160=VERTEX_POINT('',#37810);
#11161=VERTEX_POINT('',#37812);
#11162=VERTEX_POINT('',#37814);
#11163=VERTEX_POINT('',#37818);
#11164=VERTEX_POINT('',#37820);
#11165=VERTEX_POINT('',#37824);
#11166=VERTEX_POINT('',#37825);
#11167=VERTEX_POINT('',#37827);
#11168=VERTEX_POINT('',#37829);
#11169=VERTEX_POINT('',#37833);
#11170=VERTEX_POINT('',#37835);
#11171=VERTEX_POINT('',#37839);
#11172=VERTEX_POINT('',#37840);
#11173=VERTEX_POINT('',#37842);
#11174=VERTEX_POINT('',#37844);
#11175=VERTEX_POINT('',#37848);
#11176=VERTEX_POINT('',#37849);
#11177=VERTEX_POINT('',#37851);
#11178=VERTEX_POINT('',#37853);
#11179=VERTEX_POINT('',#37857);
#11180=VERTEX_POINT('',#37858);
#11181=VERTEX_POINT('',#37860);
#11182=VERTEX_POINT('',#37862);
#11183=VERTEX_POINT('',#37866);
#11184=VERTEX_POINT('',#37867);
#11185=VERTEX_POINT('',#37869);
#11186=VERTEX_POINT('',#37871);
#11187=VERTEX_POINT('',#37878);
#11188=VERTEX_POINT('',#37879);
#11189=VERTEX_POINT('',#37881);
#11190=VERTEX_POINT('',#37883);
#11191=VERTEX_POINT('',#37887);
#11192=VERTEX_POINT('',#37888);
#11193=VERTEX_POINT('',#37890);
#11194=VERTEX_POINT('',#37892);
#11195=VERTEX_POINT('',#37896);
#11196=VERTEX_POINT('',#37897);
#11197=VERTEX_POINT('',#37899);
#11198=VERTEX_POINT('',#37901);
#11199=VERTEX_POINT('',#37905);
#11200=VERTEX_POINT('',#37906);
#11201=VERTEX_POINT('',#37908);
#11202=VERTEX_POINT('',#37910);
#11203=VERTEX_POINT('',#37963);
#11204=VERTEX_POINT('',#37964);
#11205=VERTEX_POINT('',#37966);
#11206=VERTEX_POINT('',#37968);
#11207=VERTEX_POINT('',#37972);
#11208=VERTEX_POINT('',#37974);
#11209=VERTEX_POINT('',#37977);
#11210=VERTEX_POINT('',#37979);
#11211=VERTEX_POINT('',#37983);
#11212=VERTEX_POINT('',#37987);
#11213=VERTEX_POINT('',#37993);
#11214=VERTEX_POINT('',#37997);
#11215=VERTEX_POINT('',#38003);
#11216=VERTEX_POINT('',#38005);
#11217=VERTEX_POINT('',#38009);
#11218=VERTEX_POINT('',#38013);
#11219=VERTEX_POINT('',#38017);
#11220=VERTEX_POINT('',#38021);
#11221=VERTEX_POINT('',#38028);
#11222=VERTEX_POINT('',#38029);
#11223=VERTEX_POINT('',#38031);
#11224=VERTEX_POINT('',#38033);
#11225=VERTEX_POINT('',#38035);
#11226=VERTEX_POINT('',#38037);
#11227=VERTEX_POINT('',#38039);
#11228=VERTEX_POINT('',#38041);
#11229=VERTEX_POINT('',#38043);
#11230=VERTEX_POINT('',#38045);
#11231=VERTEX_POINT('',#38047);
#11232=VERTEX_POINT('',#38049);
#11233=VERTEX_POINT('',#38051);
#11234=VERTEX_POINT('',#38053);
#11235=VERTEX_POINT('',#38055);
#11236=VERTEX_POINT('',#38057);
#11237=VERTEX_POINT('',#38059);
#11238=VERTEX_POINT('',#38061);
#11239=VERTEX_POINT('',#38063);
#11240=VERTEX_POINT('',#38065);
#11241=VERTEX_POINT('',#38067);
#11242=VERTEX_POINT('',#38069);
#11243=VERTEX_POINT('',#38071);
#11244=VERTEX_POINT('',#38073);
#11245=VERTEX_POINT('',#38075);
#11246=VERTEX_POINT('',#38077);
#11247=VERTEX_POINT('',#38079);
#11248=VERTEX_POINT('',#38081);
#11249=VERTEX_POINT('',#38083);
#11250=VERTEX_POINT('',#38085);
#11251=VERTEX_POINT('',#38087);
#11252=VERTEX_POINT('',#38089);
#11253=VERTEX_POINT('',#38091);
#11254=VERTEX_POINT('',#38093);
#11255=VERTEX_POINT('',#38095);
#11256=VERTEX_POINT('',#38097);
#11257=VERTEX_POINT('',#38099);
#11258=VERTEX_POINT('',#38101);
#11259=VERTEX_POINT('',#38103);
#11260=VERTEX_POINT('',#38105);
#11261=VERTEX_POINT('',#38107);
#11262=VERTEX_POINT('',#38109);
#11263=VERTEX_POINT('',#38111);
#11264=VERTEX_POINT('',#38113);
#11265=VERTEX_POINT('',#38117);
#11266=VERTEX_POINT('',#38118);
#11267=VERTEX_POINT('',#38123);
#11268=VERTEX_POINT('',#38127);
#11269=VERTEX_POINT('',#38131);
#11270=VERTEX_POINT('',#38135);
#11271=VERTEX_POINT('',#38139);
#11272=VERTEX_POINT('',#38143);
#11273=VERTEX_POINT('',#38147);
#11274=VERTEX_POINT('',#38151);
#11275=VERTEX_POINT('',#38155);
#11276=VERTEX_POINT('',#38159);
#11277=VERTEX_POINT('',#38163);
#11278=VERTEX_POINT('',#38167);
#11279=VERTEX_POINT('',#38171);
#11280=VERTEX_POINT('',#38175);
#11281=VERTEX_POINT('',#38179);
#11282=VERTEX_POINT('',#38183);
#11283=VERTEX_POINT('',#38187);
#11284=VERTEX_POINT('',#38191);
#11285=VERTEX_POINT('',#38195);
#11286=VERTEX_POINT('',#38199);
#11287=VERTEX_POINT('',#38203);
#11288=VERTEX_POINT('',#38207);
#11289=VERTEX_POINT('',#38211);
#11290=VERTEX_POINT('',#38215);
#11291=VERTEX_POINT('',#38219);
#11292=VERTEX_POINT('',#38223);
#11293=VERTEX_POINT('',#38227);
#11294=VERTEX_POINT('',#38231);
#11295=VERTEX_POINT('',#38235);
#11296=VERTEX_POINT('',#38239);
#11297=VERTEX_POINT('',#38243);
#11298=VERTEX_POINT('',#38247);
#11299=VERTEX_POINT('',#38251);
#11300=VERTEX_POINT('',#38255);
#11301=VERTEX_POINT('',#38259);
#11302=VERTEX_POINT('',#38263);
#11303=VERTEX_POINT('',#38267);
#11304=VERTEX_POINT('',#38271);
#11305=VERTEX_POINT('',#38275);
#11306=VERTEX_POINT('',#38279);
#11307=VERTEX_POINT('',#38283);
#11308=VERTEX_POINT('',#38287);
#11309=VERTEX_POINT('',#38294);
#11310=VERTEX_POINT('',#38296);
#11311=VERTEX_POINT('',#38300);
#11312=VERTEX_POINT('',#38301);
#11313=VERTEX_POINT('',#38303);
#11314=VERTEX_POINT('',#38305);
#11315=VERTEX_POINT('',#38307);
#11316=VERTEX_POINT('',#38309);
#11317=VERTEX_POINT('',#38311);
#11318=VERTEX_POINT('',#38313);
#11319=VERTEX_POINT('',#38315);
#11320=VERTEX_POINT('',#38317);
#11321=VERTEX_POINT('',#38319);
#11322=VERTEX_POINT('',#38321);
#11323=VERTEX_POINT('',#38323);
#11324=VERTEX_POINT('',#38325);
#11325=VERTEX_POINT('',#38327);
#11326=VERTEX_POINT('',#38329);
#11327=VERTEX_POINT('',#38331);
#11328=VERTEX_POINT('',#38333);
#11329=VERTEX_POINT('',#38335);
#11330=VERTEX_POINT('',#38337);
#11331=VERTEX_POINT('',#38339);
#11332=VERTEX_POINT('',#38341);
#11333=VERTEX_POINT('',#38343);
#11334=VERTEX_POINT('',#38345);
#11335=VERTEX_POINT('',#38347);
#11336=VERTEX_POINT('',#38349);
#11337=VERTEX_POINT('',#38351);
#11338=VERTEX_POINT('',#38353);
#11339=VERTEX_POINT('',#38355);
#11340=VERTEX_POINT('',#38357);
#11341=VERTEX_POINT('',#38359);
#11342=VERTEX_POINT('',#38361);
#11343=VERTEX_POINT('',#38363);
#11344=VERTEX_POINT('',#38365);
#11345=VERTEX_POINT('',#38367);
#11346=VERTEX_POINT('',#38369);
#11347=VERTEX_POINT('',#38371);
#11348=VERTEX_POINT('',#38373);
#11349=VERTEX_POINT('',#38375);
#11350=VERTEX_POINT('',#38377);
#11351=VERTEX_POINT('',#38379);
#11352=VERTEX_POINT('',#38381);
#11353=VERTEX_POINT('',#38383);
#11354=VERTEX_POINT('',#38385);
#11355=VERTEX_POINT('',#38387);
#11356=VERTEX_POINT('',#38389);
#11357=VERTEX_POINT('',#38391);
#11358=VERTEX_POINT('',#38393);
#11359=VERTEX_POINT('',#38397);
#11360=VERTEX_POINT('',#38401);
#11361=VERTEX_POINT('',#38408);
#11362=VERTEX_POINT('',#38410);
#11363=VERTEX_POINT('',#38414);
#11364=VERTEX_POINT('',#38415);
#11365=VERTEX_POINT('',#38420);
#11366=VERTEX_POINT('',#38424);
#11367=VERTEX_POINT('',#38428);
#11368=VERTEX_POINT('',#38432);
#11369=VERTEX_POINT('',#38433);
#11370=VERTEX_POINT('',#38436);
#11371=VERTEX_POINT('',#38441);
#11372=VERTEX_POINT('',#38445);
#11373=VERTEX_POINT('',#38449);
#11374=VERTEX_POINT('',#38453);
#11375=VERTEX_POINT('',#38457);
#11376=VERTEX_POINT('',#38461);
#11377=VERTEX_POINT('',#38465);
#11378=VERTEX_POINT('',#38469);
#11379=VERTEX_POINT('',#38473);
#11380=VERTEX_POINT('',#38477);
#11381=VERTEX_POINT('',#38481);
#11382=VERTEX_POINT('',#38485);
#11383=VERTEX_POINT('',#38489);
#11384=VERTEX_POINT('',#38493);
#11385=VERTEX_POINT('',#38497);
#11386=VERTEX_POINT('',#38501);
#11387=VERTEX_POINT('',#38505);
#11388=VERTEX_POINT('',#38509);
#11389=VERTEX_POINT('',#38513);
#11390=VERTEX_POINT('',#38517);
#11391=VERTEX_POINT('',#38521);
#11392=VERTEX_POINT('',#38525);
#11393=VERTEX_POINT('',#38529);
#11394=VERTEX_POINT('',#38533);
#11395=VERTEX_POINT('',#38537);
#11396=VERTEX_POINT('',#38541);
#11397=VERTEX_POINT('',#38545);
#11398=VERTEX_POINT('',#38549);
#11399=VERTEX_POINT('',#38553);
#11400=VERTEX_POINT('',#38557);
#11401=VERTEX_POINT('',#38561);
#11402=VERTEX_POINT('',#38565);
#11403=VERTEX_POINT('',#38569);
#11404=VERTEX_POINT('',#38573);
#11405=VERTEX_POINT('',#38577);
#11406=VERTEX_POINT('',#38581);
#11407=VERTEX_POINT('',#38585);
#11408=VERTEX_POINT('',#38589);
#11409=VERTEX_POINT('',#38596);
#11410=VERTEX_POINT('',#38597);
#11411=VERTEX_POINT('',#38599);
#11412=VERTEX_POINT('',#38601);
#11413=VERTEX_POINT('',#38605);
#11414=VERTEX_POINT('',#38606);
#11415=VERTEX_POINT('',#38608);
#11416=VERTEX_POINT('',#38610);
#11417=VERTEX_POINT('',#38614);
#11418=VERTEX_POINT('',#38618);
#11419=VERTEX_POINT('',#38624);
#11420=VERTEX_POINT('',#38626);
#11421=VERTEX_POINT('',#38630);
#11422=VERTEX_POINT('',#38632);
#11423=VERTEX_POINT('',#38634);
#11424=VERTEX_POINT('',#38638);
#11425=VERTEX_POINT('',#38640);
#11426=VERTEX_POINT('',#38644);
#11427=VERTEX_POINT('',#38645);
#11428=VERTEX_POINT('',#38647);
#11429=VERTEX_POINT('',#38649);
#11430=VERTEX_POINT('',#38653);
#11431=VERTEX_POINT('',#38656);
#11432=VERTEX_POINT('',#38660);
#11433=VERTEX_POINT('',#38664);
#11434=VERTEX_POINT('',#38665);
#11435=VERTEX_POINT('',#38667);
#11436=VERTEX_POINT('',#38669);
#11437=VERTEX_POINT('',#38671);
#11438=VERTEX_POINT('',#38673);
#11439=VERTEX_POINT('',#38675);
#11440=VERTEX_POINT('',#38677);
#11441=VERTEX_POINT('',#38679);
#11442=VERTEX_POINT('',#38681);
#11443=VERTEX_POINT('',#38683);
#11444=VERTEX_POINT('',#38685);
#11445=VERTEX_POINT('',#38687);
#11446=VERTEX_POINT('',#38689);
#11447=VERTEX_POINT('',#38691);
#11448=VERTEX_POINT('',#38693);
#11449=VERTEX_POINT('',#38695);
#11450=VERTEX_POINT('',#38697);
#11451=VERTEX_POINT('',#38699);
#11452=VERTEX_POINT('',#38701);
#11453=VERTEX_POINT('',#38703);
#11454=VERTEX_POINT('',#38705);
#11455=VERTEX_POINT('',#38707);
#11456=VERTEX_POINT('',#38709);
#11457=VERTEX_POINT('',#38711);
#11458=VERTEX_POINT('',#38713);
#11459=VERTEX_POINT('',#38715);
#11460=VERTEX_POINT('',#38717);
#11461=VERTEX_POINT('',#38719);
#11462=VERTEX_POINT('',#38721);
#11463=VERTEX_POINT('',#38723);
#11464=VERTEX_POINT('',#38725);
#11465=VERTEX_POINT('',#38727);
#11466=VERTEX_POINT('',#38729);
#11467=VERTEX_POINT('',#38731);
#11468=VERTEX_POINT('',#38733);
#11469=VERTEX_POINT('',#38735);
#11470=VERTEX_POINT('',#38737);
#11471=VERTEX_POINT('',#38739);
#11472=VERTEX_POINT('',#38741);
#11473=VERTEX_POINT('',#38743);
#11474=VERTEX_POINT('',#38745);
#11475=VERTEX_POINT('',#38747);
#11476=VERTEX_POINT('',#38749);
#11477=VERTEX_POINT('',#38753);
#11478=VERTEX_POINT('',#38757);
#11479=VERTEX_POINT('',#38761);
#11480=VERTEX_POINT('',#38762);
#11481=VERTEX_POINT('',#38767);
#11482=VERTEX_POINT('',#38769);
#11483=VERTEX_POINT('',#38773);
#11484=VERTEX_POINT('',#38775);
#11485=VERTEX_POINT('',#38779);
#11486=VERTEX_POINT('',#38781);
#11487=VERTEX_POINT('',#38789);
#11488=VERTEX_POINT('',#38791);
#11489=VERTEX_POINT('',#38793);
#11490=VERTEX_POINT('',#38797);
#11491=VERTEX_POINT('',#38798);
#11492=VERTEX_POINT('',#38803);
#11493=VERTEX_POINT('',#38805);
#11494=VERTEX_POINT('',#38809);
#11495=VERTEX_POINT('',#38810);
#11496=VERTEX_POINT('',#38815);
#11497=VERTEX_POINT('',#38820);
#11498=VERTEX_POINT('',#38822);
#11499=VERTEX_POINT('',#38829);
#11500=VERTEX_POINT('',#38830);
#11501=VERTEX_POINT('',#38835);
#11502=VERTEX_POINT('',#38839);
#11503=VERTEX_POINT('',#38843);
#11504=VERTEX_POINT('',#38847);
#11505=VERTEX_POINT('',#38851);
#11506=VERTEX_POINT('',#38855);
#11507=VERTEX_POINT('',#38859);
#11508=VERTEX_POINT('',#38863);
#11509=VERTEX_POINT('',#38867);
#11510=VERTEX_POINT('',#38871);
#11511=VERTEX_POINT('',#38875);
#11512=VERTEX_POINT('',#38879);
#11513=VERTEX_POINT('',#38883);
#11514=VERTEX_POINT('',#38887);
#11515=VERTEX_POINT('',#38891);
#11516=VERTEX_POINT('',#38895);
#11517=VERTEX_POINT('',#38899);
#11518=VERTEX_POINT('',#38903);
#11519=VERTEX_POINT('',#38907);
#11520=VERTEX_POINT('',#38911);
#11521=VERTEX_POINT('',#38915);
#11522=VERTEX_POINT('',#38919);
#11523=VERTEX_POINT('',#38923);
#11524=VERTEX_POINT('',#38927);
#11525=VERTEX_POINT('',#38931);
#11526=VERTEX_POINT('',#38935);
#11527=VERTEX_POINT('',#38939);
#11528=VERTEX_POINT('',#38943);
#11529=VERTEX_POINT('',#38947);
#11530=VERTEX_POINT('',#38951);
#11531=VERTEX_POINT('',#38955);
#11532=VERTEX_POINT('',#38959);
#11533=VERTEX_POINT('',#38963);
#11534=VERTEX_POINT('',#38967);
#11535=VERTEX_POINT('',#38971);
#11536=VERTEX_POINT('',#38975);
#11537=VERTEX_POINT('',#38979);
#11538=VERTEX_POINT('',#38983);
#11539=VERTEX_POINT('',#38987);
#11540=VERTEX_POINT('',#38991);
#11541=VERTEX_POINT('',#38995);
#11542=VERTEX_POINT('',#38999);
#11543=VERTEX_POINT('',#39005);
#11544=VERTEX_POINT('',#39006);
#11545=VERTEX_POINT('',#39008);
#11546=VERTEX_POINT('',#39010);
#11547=VERTEX_POINT('',#39014);
#11548=VERTEX_POINT('',#39016);
#11549=VERTEX_POINT('',#39020);
#11550=VERTEX_POINT('',#39022);
#11551=VERTEX_POINT('',#39026);
#11552=VERTEX_POINT('',#39028);
#11553=VERTEX_POINT('',#39032);
#11554=VERTEX_POINT('',#39034);
#11555=VERTEX_POINT('',#39038);
#11556=VERTEX_POINT('',#39039);
#11557=VERTEX_POINT('',#39041);
#11558=VERTEX_POINT('',#39043);
#11559=VERTEX_POINT('',#39047);
#11560=VERTEX_POINT('',#39049);
#11561=VERTEX_POINT('',#39053);
#11562=VERTEX_POINT('',#39055);
#11563=VERTEX_POINT('',#39062);
#11564=VERTEX_POINT('',#39064);
#11565=VERTEX_POINT('',#39066);
#11566=VERTEX_POINT('',#39070);
#11567=VERTEX_POINT('',#39072);
#11568=VERTEX_POINT('',#39076);
#11569=VERTEX_POINT('',#39077);
#11570=VERTEX_POINT('',#39082);
#11571=VERTEX_POINT('',#39083);
#11572=VERTEX_POINT('',#39088);
#11573=VERTEX_POINT('',#39089);
#11574=VERTEX_POINT('',#39094);
#11575=VERTEX_POINT('',#39095);
#11576=VERTEX_POINT('',#39100);
#11577=VERTEX_POINT('',#39102);
#11578=VERTEX_POINT('',#39106);
#11579=VERTEX_POINT('',#39107);
#11580=VERTEX_POINT('',#39112);
#11581=VERTEX_POINT('',#39113);
#11582=VERTEX_POINT('',#39118);
#11583=VERTEX_POINT('',#39119);
#11584=VERTEX_POINT('',#39124);
#11585=VERTEX_POINT('',#39126);
#11586=VERTEX_POINT('',#39130);
#11587=VERTEX_POINT('',#39132);
#11588=VERTEX_POINT('',#39136);
#11589=VERTEX_POINT('',#39138);
#11590=VERTEX_POINT('',#39142);
#11591=VERTEX_POINT('',#39144);
#11592=VERTEX_POINT('',#39148);
#11593=VERTEX_POINT('',#39153);
#11594=VERTEX_POINT('',#39155);
#11595=VERTEX_POINT('',#39159);
#11596=VERTEX_POINT('',#39160);
#11597=VERTEX_POINT('',#39165);
#11598=VERTEX_POINT('',#39167);
#11599=VERTEX_POINT('',#39171);
#11600=VERTEX_POINT('',#39173);
#11601=VERTEX_POINT('',#39177);
#11602=VERTEX_POINT('',#39178);
#11603=VERTEX_POINT('',#39187);
#11604=VERTEX_POINT('',#39191);
#11605=VERTEX_POINT('',#39193);
#11606=VERTEX_POINT('',#39197);
#11607=VERTEX_POINT('',#39199);
#11608=VERTEX_POINT('',#39204);
#11609=VERTEX_POINT('',#39211);
#11610=VERTEX_POINT('',#39213);
#11611=VERTEX_POINT('',#39215);
#11612=VERTEX_POINT('',#39217);
#11613=VERTEX_POINT('',#39219);
#11614=VERTEX_POINT('',#39221);
#11615=VERTEX_POINT('',#39223);
#11616=VERTEX_POINT('',#39225);
#11617=VERTEX_POINT('',#39227);
#11618=VERTEX_POINT('',#39229);
#11619=VERTEX_POINT('',#39231);
#11620=VERTEX_POINT('',#39233);
#11621=VERTEX_POINT('',#39235);
#11622=VERTEX_POINT('',#39237);
#11623=VERTEX_POINT('',#39239);
#11624=VERTEX_POINT('',#39241);
#11625=VERTEX_POINT('',#39243);
#11626=VERTEX_POINT('',#39245);
#11627=VERTEX_POINT('',#39247);
#11628=VERTEX_POINT('',#39249);
#11629=VERTEX_POINT('',#39251);
#11630=VERTEX_POINT('',#39253);
#11631=VERTEX_POINT('',#39255);
#11632=VERTEX_POINT('',#39257);
#11633=VERTEX_POINT('',#39259);
#11634=VERTEX_POINT('',#39261);
#11635=VERTEX_POINT('',#39263);
#11636=VERTEX_POINT('',#39265);
#11637=VERTEX_POINT('',#39267);
#11638=VERTEX_POINT('',#39269);
#11639=VERTEX_POINT('',#39271);
#11640=VERTEX_POINT('',#39273);
#11641=VERTEX_POINT('',#39275);
#11642=VERTEX_POINT('',#39277);
#11643=VERTEX_POINT('',#39279);
#11644=VERTEX_POINT('',#39281);
#11645=VERTEX_POINT('',#39285);
#11646=VERTEX_POINT('',#39287);
#11647=VERTEX_POINT('',#39289);
#11648=VERTEX_POINT('',#39291);
#11649=VERTEX_POINT('',#39293);
#11650=VERTEX_POINT('',#39295);
#11651=VERTEX_POINT('',#39297);
#11652=VERTEX_POINT('',#39299);
#11653=VERTEX_POINT('',#39301);
#11654=VERTEX_POINT('',#39303);
#11655=VERTEX_POINT('',#39305);
#11656=VERTEX_POINT('',#39307);
#11657=VERTEX_POINT('',#39311);
#11658=VERTEX_POINT('',#39312);
#11659=VERTEX_POINT('',#39317);
#11660=VERTEX_POINT('',#39318);
#11661=VERTEX_POINT('',#39323);
#11662=VERTEX_POINT('',#39327);
#11663=VERTEX_POINT('',#39331);
#11664=VERTEX_POINT('',#39335);
#11665=VERTEX_POINT('',#39337);
#11666=VERTEX_POINT('',#39341);
#11667=VERTEX_POINT('',#39343);
#11668=VERTEX_POINT('',#39349);
#11669=VERTEX_POINT('',#39355);
#11670=VERTEX_POINT('',#39356);
#11671=VERTEX_POINT('',#39361);
#11672=VERTEX_POINT('',#39362);
#11673=VERTEX_POINT('',#39369);
#11674=VERTEX_POINT('',#39370);
#11675=VERTEX_POINT('',#39375);
#11676=VERTEX_POINT('',#39376);
#11677=VERTEX_POINT('',#39385);
#11678=VERTEX_POINT('',#39386);
#11679=VERTEX_POINT('',#39391);
#11680=VERTEX_POINT('',#39392);
#11681=VERTEX_POINT('',#39399);
#11682=VERTEX_POINT('',#39401);
#11683=VERTEX_POINT('',#39407);
#11684=VERTEX_POINT('',#39408);
#11685=VERTEX_POINT('',#39413);
#11686=VERTEX_POINT('',#39414);
#11687=VERTEX_POINT('',#39421);
#11688=VERTEX_POINT('',#39422);
#11689=VERTEX_POINT('',#39427);
#11690=VERTEX_POINT('',#39428);
#11691=VERTEX_POINT('',#39439);
#11692=VERTEX_POINT('',#39440);
#11693=VERTEX_POINT('',#39445);
#11694=VERTEX_POINT('',#39446);
#11695=VERTEX_POINT('',#39453);
#11696=VERTEX_POINT('',#39455);
#11697=VERTEX_POINT('',#39459);
#11698=VERTEX_POINT('',#39461);
#11699=VERTEX_POINT('',#39465);
#11700=VERTEX_POINT('',#39466);
#11701=VERTEX_POINT('',#39471);
#11702=VERTEX_POINT('',#39475);
#11703=VERTEX_POINT('',#39481);
#11704=VERTEX_POINT('',#39497);
#11705=VERTEX_POINT('',#39504);
#11706=VERTEX_POINT('',#39508);
#13635=EDGE_CURVE('',#11068,#11068,#9707,.T.);
#13636=EDGE_CURVE('',#11068,#11069,#5822,.T.);
#13637=EDGE_CURVE('',#11069,#11069,#9708,.T.);
#13638=EDGE_CURVE('',#11070,#11070,#9709,.T.);
#13639=EDGE_CURVE('',#11070,#11071,#5823,.T.);
#13640=EDGE_CURVE('',#11071,#11071,#9710,.T.);
#13641=EDGE_CURVE('',#11072,#11072,#9711,.T.);
#13642=EDGE_CURVE('',#11072,#11073,#5824,.T.);
#13643=EDGE_CURVE('',#11073,#11073,#9712,.T.);
#13644=EDGE_CURVE('',#11074,#11068,#5825,.T.);
#13645=EDGE_CURVE('',#11075,#11070,#5826,.T.);
#13646=EDGE_CURVE('',#11076,#11076,#9713,.T.);
#13647=EDGE_CURVE('',#11076,#11077,#5827,.T.);
#13648=EDGE_CURVE('',#11077,#11077,#9714,.T.);
#13649=EDGE_CURVE('',#11078,#11078,#9715,.T.);
#13650=EDGE_CURVE('',#11078,#11079,#5828,.T.);
#13651=EDGE_CURVE('',#11079,#11079,#9716,.T.);
#13652=EDGE_CURVE('',#11080,#11080,#9717,.T.);
#13653=EDGE_CURVE('',#11080,#11081,#5829,.T.);
#13654=EDGE_CURVE('',#11081,#11081,#9718,.T.);
#13655=EDGE_CURVE('',#11082,#11082,#9719,.T.);
#13656=EDGE_CURVE('',#11082,#11083,#5830,.T.);
#13657=EDGE_CURVE('',#11083,#11083,#9720,.T.);
#13658=EDGE_CURVE('',#11084,#11084,#9721,.T.);
#13659=EDGE_CURVE('',#11084,#11085,#5831,.T.);
#13660=EDGE_CURVE('',#11085,#11085,#9722,.T.);
#13661=EDGE_CURVE('',#11086,#11086,#9723,.T.);
#13662=EDGE_CURVE('',#11086,#11087,#5832,.T.);
#13663=EDGE_CURVE('',#11087,#11087,#9724,.T.);
#13664=EDGE_CURVE('',#11088,#11088,#9725,.T.);
#13665=EDGE_CURVE('',#11088,#11089,#5833,.T.);
#13666=EDGE_CURVE('',#11089,#11089,#9726,.T.);
#13667=EDGE_CURVE('',#11090,#11090,#9727,.T.);
#13668=EDGE_CURVE('',#11090,#11091,#5834,.T.);
#13669=EDGE_CURVE('',#11091,#11092,#9728,.T.);
#13670=EDGE_CURVE('',#11092,#11093,#5835,.T.);
#13671=EDGE_CURVE('',#11093,#11094,#9729,.T.);
#13672=EDGE_CURVE('',#11091,#11094,#5836,.T.);
#13673=EDGE_CURVE('',#11095,#11084,#5837,.T.);
#13674=EDGE_CURVE('',#11096,#11086,#5838,.T.);
#13675=EDGE_CURVE('',#11097,#11097,#9730,.T.);
#13676=EDGE_CURVE('',#11097,#11098,#5839,.T.);
#13677=EDGE_CURVE('',#11098,#11099,#5840,.T.);
#13678=EDGE_CURVE('',#11099,#11100,#9731,.T.);
#13679=EDGE_CURVE('',#11101,#11100,#5841,.T.);
#13680=EDGE_CURVE('',#11101,#11098,#9732,.T.);
#13681=EDGE_CURVE('',#11102,#11103,#109,.T.);
#13682=EDGE_CURVE('',#11104,#11102,#110,.T.);
#13683=EDGE_CURVE('',#11105,#11104,#111,.T.);
#13684=EDGE_CURVE('',#11105,#11106,#82,.T.);
#13685=EDGE_CURVE('',#11107,#11106,#9733,.T.);
#13686=EDGE_CURVE('',#11106,#11107,#9734,.T.);
#13687=EDGE_CURVE('',#11108,#11105,#112,.T.);
#13688=EDGE_CURVE('',#11109,#11108,#113,.T.);
#13689=EDGE_CURVE('',#11103,#11109,#114,.T.);
#13690=EDGE_CURVE('',#11110,#11110,#9735,.T.);
#13691=EDGE_CURVE('',#11110,#11107,#5842,.T.);
#13692=EDGE_CURVE('',#11111,#11111,#9736,.T.);
#13693=EDGE_CURVE('',#11111,#11112,#5843,.T.);
#13694=EDGE_CURVE('',#11112,#11112,#9737,.T.);
#13695=EDGE_CURVE('',#11113,#11114,#642,.T.);
#13696=EDGE_CURVE('',#11115,#11113,#5844,.T.);
#13697=EDGE_CURVE('',#11115,#11116,#5845,.T.);
#13698=EDGE_CURVE('',#11116,#11114,#5846,.T.);
#13699=EDGE_CURVE('',#11117,#11113,#643,.T.);
#13700=EDGE_CURVE('',#11117,#11118,#5847,.T.);
#13701=EDGE_CURVE('',#11119,#11118,#644,.T.);
#13702=EDGE_CURVE('',#11113,#11119,#5848,.T.);
#13703=EDGE_CURVE('',#11120,#11121,#645,.T.);
#13704=EDGE_CURVE('',#11120,#11122,#5849,.T.);
#13705=EDGE_CURVE('',#11123,#11122,#646,.T.);
#13706=EDGE_CURVE('',#11121,#11123,#5850,.T.);
#13707=EDGE_CURVE('',#11122,#11124,#647,.T.);
#13708=EDGE_CURVE('',#11122,#11125,#5851,.T.);
#13709=EDGE_CURVE('',#11126,#11125,#5852,.T.);
#13710=EDGE_CURVE('',#11124,#11126,#5853,.T.);
#13711=EDGE_CURVE('',#11127,#11128,#5854,.T.);
#13712=EDGE_CURVE('',#11127,#11129,#5855,.T.);
#13713=EDGE_CURVE('',#11129,#11130,#5856,.T.);
#13714=EDGE_CURVE('',#11130,#11128,#5857,.T.);
#13715=EDGE_CURVE('',#11131,#11132,#5858,.T.);
#13716=EDGE_CURVE('',#11131,#11133,#5859,.T.);
#13717=EDGE_CURVE('',#11133,#11134,#5860,.T.);
#13718=EDGE_CURVE('',#11134,#11132,#5861,.T.);
#13719=EDGE_CURVE('',#11135,#11136,#5862,.T.);
#13720=EDGE_CURVE('',#11135,#11137,#5863,.T.);
#13721=EDGE_CURVE('',#11137,#11138,#5864,.T.);
#13722=EDGE_CURVE('',#11138,#11136,#5865,.T.);
#13723=EDGE_CURVE('',#11139,#11140,#5866,.T.);
#13724=EDGE_CURVE('',#11139,#11141,#5867,.T.);
#13725=EDGE_CURVE('',#11141,#11142,#5868,.T.);
#13726=EDGE_CURVE('',#11142,#11140,#5869,.T.);
#13727=EDGE_CURVE('',#11143,#11144,#5870,.T.);
#13728=EDGE_CURVE('',#11143,#11145,#5871,.T.);
#13729=EDGE_CURVE('',#11145,#11146,#5872,.T.);
#13730=EDGE_CURVE('',#11146,#11144,#5873,.T.);
#13731=EDGE_CURVE('',#11147,#11148,#5874,.T.);
#13732=EDGE_CURVE('',#11147,#11149,#5875,.T.);
#13733=EDGE_CURVE('',#11149,#11150,#5876,.T.);
#13734=EDGE_CURVE('',#11150,#11148,#5877,.T.);
#13735=EDGE_CURVE('',#11151,#11152,#5878,.T.);
#13736=EDGE_CURVE('',#11151,#11153,#5879,.T.);
#13737=EDGE_CURVE('',#11153,#11154,#5880,.T.);
#13738=EDGE_CURVE('',#11154,#11152,#5881,.T.);
#13739=EDGE_CURVE('',#11155,#11156,#5882,.T.);
#13740=EDGE_CURVE('',#11155,#11157,#5883,.T.);
#13741=EDGE_CURVE('',#11157,#11158,#5884,.T.);
#13742=EDGE_CURVE('',#11158,#11156,#5885,.T.);
#13743=EDGE_CURVE('',#11159,#11160,#5886,.T.);
#13744=EDGE_CURVE('',#11161,#11159,#5887,.T.);
#13745=EDGE_CURVE('',#11161,#11162,#5888,.T.);
#13746=EDGE_CURVE('',#11162,#11160,#5889,.T.);
#13747=EDGE_CURVE('',#11163,#11159,#5890,.T.);
#13748=EDGE_CURVE('',#11164,#11163,#5891,.T.);
#13749=EDGE_CURVE('',#11164,#11161,#5892,.T.);
#13750=EDGE_CURVE('',#11165,#11166,#5893,.T.);
#13751=EDGE_CURVE('',#11167,#11165,#5894,.T.);
#13752=EDGE_CURVE('',#11167,#11168,#5895,.T.);
#13753=EDGE_CURVE('',#11168,#11166,#5896,.T.);
#13754=EDGE_CURVE('',#11169,#11165,#5897,.T.);
#13755=EDGE_CURVE('',#11169,#11170,#5898,.T.);
#13756=EDGE_CURVE('',#11170,#11167,#5899,.T.);
#13757=EDGE_CURVE('',#11171,#11172,#5900,.T.);
#13758=EDGE_CURVE('',#11171,#11173,#5901,.T.);
#13759=EDGE_CURVE('',#11173,#11174,#5902,.T.);
#13760=EDGE_CURVE('',#11174,#11172,#5903,.T.);
#13761=EDGE_CURVE('',#11175,#11176,#5904,.T.);
#13762=EDGE_CURVE('',#11175,#11177,#5905,.T.);
#13763=EDGE_CURVE('',#11177,#11178,#5906,.T.);
#13764=EDGE_CURVE('',#11178,#11176,#5907,.T.);
#13765=EDGE_CURVE('',#11179,#11180,#5908,.T.);
#13766=EDGE_CURVE('',#11179,#11181,#5909,.T.);
#13767=EDGE_CURVE('',#11181,#11182,#5910,.T.);
#13768=EDGE_CURVE('',#11182,#11180,#5911,.T.);
#13769=EDGE_CURVE('',#11183,#11184,#5912,.T.);
#13770=EDGE_CURVE('',#11185,#11183,#5913,.T.);
#13771=EDGE_CURVE('',#11185,#11186,#5914,.T.);
#13772=EDGE_CURVE('',#11186,#11184,#5915,.T.);
#13773=EDGE_CURVE('',#11140,#11183,#5916,.T.);
#13774=EDGE_CURVE('',#11142,#11185,#5917,.T.);
#13775=EDGE_CURVE('',#11187,#11188,#9738,.T.);
#13776=EDGE_CURVE('',#11187,#11189,#5918,.T.);
#13777=EDGE_CURVE('',#11189,#11190,#9739,.T.);
#13778=EDGE_CURVE('',#11190,#11188,#5919,.T.);
#13779=EDGE_CURVE('',#11191,#11192,#9740,.T.);
#13780=EDGE_CURVE('',#11191,#11193,#5920,.T.);
#13781=EDGE_CURVE('',#11193,#11194,#9741,.T.);
#13782=EDGE_CURVE('',#11194,#11192,#5921,.T.);
#13783=EDGE_CURVE('',#11195,#11196,#9742,.T.);
#13784=EDGE_CURVE('',#11195,#11197,#5922,.T.);
#13785=EDGE_CURVE('',#11197,#11198,#9743,.T.);
#13786=EDGE_CURVE('',#11198,#11196,#5923,.T.);
#13787=EDGE_CURVE('',#11199,#11200,#9744,.T.);
#13788=EDGE_CURVE('',#11199,#11201,#5924,.T.);
#13789=EDGE_CURVE('',#11201,#11202,#9745,.T.);
#13790=EDGE_CURVE('',#11202,#11200,#5925,.T.);
#13791=EDGE_CURVE('',#11172,#11169,#9746,.T.);
#13792=EDGE_CURVE('',#11170,#11174,#9747,.T.);
#13793=EDGE_CURVE('',#11160,#11155,#9748,.T.);
#13794=EDGE_CURVE('',#11157,#11162,#9749,.T.);
#13795=EDGE_CURVE('',#11180,#11175,#9750,.T.);
#13796=EDGE_CURVE('',#11177,#11182,#9751,.T.);
#13797=EDGE_CURVE('',#11132,#11179,#9752,.T.);
#13798=EDGE_CURVE('',#11181,#11134,#9753,.T.);
#13799=EDGE_CURVE('',#11196,#11131,#9754,.T.);
#13800=EDGE_CURVE('',#11133,#11198,#9755,.T.);
#13801=EDGE_CURVE('',#11184,#11195,#9756,.T.);
#13802=EDGE_CURVE('',#11197,#11186,#9757,.T.);
#13803=EDGE_CURVE('',#11176,#11199,#9758,.T.);
#13804=EDGE_CURVE('',#11201,#11178,#9759,.T.);
#13805=EDGE_CURVE('',#11200,#11127,#9760,.T.);
#13806=EDGE_CURVE('',#11129,#11202,#9761,.T.);
#13807=EDGE_CURVE('',#11128,#11171,#9762,.T.);
#13808=EDGE_CURVE('',#11173,#11130,#9763,.T.);
#13809=EDGE_CURVE('',#11156,#11151,#9764,.T.);
#13810=EDGE_CURVE('',#11153,#11158,#9765,.T.);
#13811=EDGE_CURVE('',#11152,#11191,#9766,.T.);
#13812=EDGE_CURVE('',#11193,#11154,#9767,.T.);
#13813=EDGE_CURVE('',#11192,#11135,#9768,.T.);
#13814=EDGE_CURVE('',#11137,#11194,#9769,.T.);
#13815=EDGE_CURVE('',#11136,#11147,#9770,.T.);
#13816=EDGE_CURVE('',#11149,#11138,#9771,.T.);
#13817=EDGE_CURVE('',#11148,#11143,#9772,.T.);
#13818=EDGE_CURVE('',#11145,#11150,#9773,.T.);
#13819=EDGE_CURVE('',#11144,#11187,#9774,.T.);
#13820=EDGE_CURVE('',#11189,#11146,#9775,.T.);
#13821=EDGE_CURVE('',#11188,#11139,#9776,.T.);
#13822=EDGE_CURVE('',#11141,#11190,#9777,.T.);
#13823=EDGE_CURVE('',#11203,#11204,#5926,.T.);
#13824=EDGE_CURVE('',#11205,#11204,#5927,.T.);
#13825=EDGE_CURVE('',#11206,#11205,#5928,.T.);
#13826=EDGE_CURVE('',#11203,#11206,#5929,.T.);
#13827=EDGE_CURVE('',#11164,#11207,#5930,.T.);
#13828=EDGE_CURVE('',#11207,#11208,#5931,.T.);
#13829=EDGE_CURVE('',#11208,#11203,#5932,.T.);
#13830=EDGE_CURVE('',#11206,#11209,#5933,.T.);
#13831=EDGE_CURVE('',#11209,#11210,#5934,.T.);
#13832=EDGE_CURVE('',#11210,#11168,#5935,.T.);
#13833=EDGE_CURVE('',#11208,#11211,#5936,.T.);
#13834=EDGE_CURVE('',#11204,#11211,#5937,.T.);
#13835=EDGE_CURVE('',#11207,#11212,#5938,.T.);
#13836=EDGE_CURVE('',#11211,#11212,#5939,.T.);
#13837=EDGE_CURVE('',#11212,#11163,#5940,.T.);
#13838=EDGE_CURVE('',#11210,#11213,#5941,.T.);
#13839=EDGE_CURVE('',#11166,#11213,#5942,.T.);
#13840=EDGE_CURVE('',#11209,#11214,#5943,.T.);
#13841=EDGE_CURVE('',#11213,#11214,#5944,.T.);
#13842=EDGE_CURVE('',#11214,#11205,#5945,.T.);
#13843=EDGE_CURVE('',#11215,#11103,#5946,.T.);
#13844=EDGE_CURVE('',#11216,#11109,#5947,.T.);
#13845=EDGE_CURVE('',#11215,#11216,#5948,.T.);
#13846=EDGE_CURVE('',#11217,#11215,#5949,.T.);
#13847=EDGE_CURVE('',#11217,#11102,#5950,.T.);
#13848=EDGE_CURVE('',#11218,#11104,#5951,.T.);
#13849=EDGE_CURVE('',#11218,#11217,#5952,.T.);
#13850=EDGE_CURVE('',#11219,#11105,#5953,.T.);
#13851=EDGE_CURVE('',#11219,#11218,#5954,.T.);
#13852=EDGE_CURVE('',#11220,#11108,#5955,.T.);
#13853=EDGE_CURVE('',#11220,#11219,#5956,.T.);
#13854=EDGE_CURVE('',#11216,#11220,#5957,.T.);
#13855=EDGE_CURVE('',#11221,#11222,#5958,.T.);
#13856=EDGE_CURVE('',#11223,#11221,#9778,.T.);
#13857=EDGE_CURVE('',#11224,#11223,#5959,.T.);
#13858=EDGE_CURVE('',#11225,#11224,#9779,.T.);
#13859=EDGE_CURVE('',#11226,#11225,#5960,.T.);
#13860=EDGE_CURVE('',#11227,#11226,#9780,.T.);
#13861=EDGE_CURVE('',#11228,#11227,#9781,.T.);
#13862=EDGE_CURVE('',#11229,#11228,#9782,.T.);
#13863=EDGE_CURVE('',#11230,#11229,#5961,.T.);
#13864=EDGE_CURVE('',#11231,#11230,#9783,.T.);
#13865=EDGE_CURVE('',#11232,#11231,#5962,.T.);
#13866=EDGE_CURVE('',#11233,#11232,#9784,.T.);
#13867=EDGE_CURVE('',#11234,#11233,#5963,.T.);
#13868=EDGE_CURVE('',#11235,#11234,#9785,.T.);
#13869=EDGE_CURVE('',#11236,#11235,#9786,.T.);
#13870=EDGE_CURVE('',#11237,#11236,#9787,.T.);
#13871=EDGE_CURVE('',#11238,#11237,#5964,.T.);
#13872=EDGE_CURVE('',#11239,#11238,#5965,.T.);
#13873=EDGE_CURVE('',#11240,#11239,#5966,.T.);
#13874=EDGE_CURVE('',#11241,#11240,#9788,.T.);
#13875=EDGE_CURVE('',#11242,#11241,#9789,.T.);
#13876=EDGE_CURVE('',#11243,#11242,#9790,.T.);
#13877=EDGE_CURVE('',#11244,#11243,#5967,.T.);
#13878=EDGE_CURVE('',#11245,#11244,#9791,.T.);
#13879=EDGE_CURVE('',#11246,#11245,#5968,.T.);
#13880=EDGE_CURVE('',#11247,#11246,#9792,.T.);
#13881=EDGE_CURVE('',#11248,#11247,#5969,.T.);
#13882=EDGE_CURVE('',#11249,#11248,#9793,.T.);
#13883=EDGE_CURVE('',#11250,#11249,#9794,.T.);
#13884=EDGE_CURVE('',#11251,#11250,#9795,.T.);
#13885=EDGE_CURVE('',#11252,#11251,#5970,.T.);
#13886=EDGE_CURVE('',#11253,#11252,#9796,.T.);
#13887=EDGE_CURVE('',#11254,#11253,#5971,.T.);
#13888=EDGE_CURVE('',#11255,#11254,#9797,.T.);
#13889=EDGE_CURVE('',#11256,#11255,#5972,.T.);
#13890=EDGE_CURVE('',#11257,#11256,#5973,.T.);
#13891=EDGE_CURVE('',#11258,#11257,#5974,.T.);
#13892=EDGE_CURVE('',#11259,#11258,#5975,.T.);
#13893=EDGE_CURVE('',#11260,#11259,#5976,.T.);
#13894=EDGE_CURVE('',#11261,#11260,#5977,.T.);
#13895=EDGE_CURVE('',#11262,#11261,#5978,.T.);
#13896=EDGE_CURVE('',#11263,#11262,#5979,.T.);
#13897=EDGE_CURVE('',#11264,#11263,#5980,.T.);
#13898=EDGE_CURVE('',#11222,#11264,#5981,.T.);
#13899=EDGE_CURVE('',#11265,#11266,#5982,.T.);
#13900=EDGE_CURVE('',#11221,#11265,#5983,.T.);
#13901=EDGE_CURVE('',#11222,#11266,#5984,.T.);
#13902=EDGE_CURVE('',#11267,#11265,#9798,.T.);
#13903=EDGE_CURVE('',#11223,#11267,#5985,.T.);
#13904=EDGE_CURVE('',#11268,#11267,#5986,.T.);
#13905=EDGE_CURVE('',#11224,#11268,#5987,.T.);
#13906=EDGE_CURVE('',#11269,#11268,#9799,.T.);
#13907=EDGE_CURVE('',#11225,#11269,#5988,.T.);
#13908=EDGE_CURVE('',#11270,#11269,#5989,.T.);
#13909=EDGE_CURVE('',#11226,#11270,#5990,.T.);
#13910=EDGE_CURVE('',#11271,#11270,#9800,.T.);
#13911=EDGE_CURVE('',#11227,#11271,#5991,.T.);
#13912=EDGE_CURVE('',#11272,#11271,#9801,.T.);
#13913=EDGE_CURVE('',#11228,#11272,#5992,.T.);
#13914=EDGE_CURVE('',#11273,#11272,#9802,.T.);
#13915=EDGE_CURVE('',#11229,#11273,#5993,.T.);
#13916=EDGE_CURVE('',#11274,#11273,#5994,.T.);
#13917=EDGE_CURVE('',#11230,#11274,#5995,.T.);
#13918=EDGE_CURVE('',#11275,#11274,#9803,.T.);
#13919=EDGE_CURVE('',#11231,#11275,#5996,.T.);
#13920=EDGE_CURVE('',#11276,#11275,#5997,.T.);
#13921=EDGE_CURVE('',#11232,#11276,#5998,.T.);
#13922=EDGE_CURVE('',#11277,#11276,#9804,.T.);
#13923=EDGE_CURVE('',#11233,#11277,#5999,.T.);
#13924=EDGE_CURVE('',#11278,#11277,#6000,.T.);
#13925=EDGE_CURVE('',#11234,#11278,#6001,.T.);
#13926=EDGE_CURVE('',#11279,#11278,#9805,.T.);
#13927=EDGE_CURVE('',#11235,#11279,#6002,.T.);
#13928=EDGE_CURVE('',#11280,#11279,#9806,.T.);
#13929=EDGE_CURVE('',#11236,#11280,#6003,.T.);
#13930=EDGE_CURVE('',#11281,#11280,#9807,.T.);
#13931=EDGE_CURVE('',#11237,#11281,#6004,.T.);
#13932=EDGE_CURVE('',#11282,#11281,#6005,.T.);
#13933=EDGE_CURVE('',#11238,#11282,#6006,.T.);
#13934=EDGE_CURVE('',#11283,#11282,#6007,.T.);
#13935=EDGE_CURVE('',#11239,#11283,#6008,.T.);
#13936=EDGE_CURVE('',#11284,#11283,#6009,.T.);
#13937=EDGE_CURVE('',#11240,#11284,#6010,.T.);
#13938=EDGE_CURVE('',#11285,#11284,#9808,.T.);
#13939=EDGE_CURVE('',#11241,#11285,#6011,.T.);
#13940=EDGE_CURVE('',#11286,#11285,#9809,.T.);
#13941=EDGE_CURVE('',#11242,#11286,#6012,.T.);
#13942=EDGE_CURVE('',#11287,#11286,#9810,.T.);
#13943=EDGE_CURVE('',#11243,#11287,#6013,.T.);
#13944=EDGE_CURVE('',#11288,#11287,#6014,.T.);
#13945=EDGE_CURVE('',#11244,#11288,#6015,.T.);
#13946=EDGE_CURVE('',#11289,#11288,#9811,.T.);
#13947=EDGE_CURVE('',#11245,#11289,#6016,.T.);
#13948=EDGE_CURVE('',#11290,#11289,#6017,.T.);
#13949=EDGE_CURVE('',#11246,#11290,#6018,.T.);
#13950=EDGE_CURVE('',#11291,#11290,#9812,.T.);
#13951=EDGE_CURVE('',#11247,#11291,#6019,.T.);
#13952=EDGE_CURVE('',#11292,#11291,#6020,.T.);
#13953=EDGE_CURVE('',#11248,#11292,#6021,.T.);
#13954=EDGE_CURVE('',#11293,#11292,#9813,.T.);
#13955=EDGE_CURVE('',#11249,#11293,#6022,.T.);
#13956=EDGE_CURVE('',#11294,#11293,#9814,.T.);
#13957=EDGE_CURVE('',#11250,#11294,#6023,.T.);
#13958=EDGE_CURVE('',#11295,#11294,#9815,.T.);
#13959=EDGE_CURVE('',#11251,#11295,#6024,.T.);
#13960=EDGE_CURVE('',#11296,#11295,#6025,.T.);
#13961=EDGE_CURVE('',#11252,#11296,#6026,.T.);
#13962=EDGE_CURVE('',#11297,#11296,#9816,.T.);
#13963=EDGE_CURVE('',#11253,#11297,#6027,.T.);
#13964=EDGE_CURVE('',#11298,#11297,#6028,.T.);
#13965=EDGE_CURVE('',#11254,#11298,#6029,.T.);
#13966=EDGE_CURVE('',#11299,#11298,#9817,.T.);
#13967=EDGE_CURVE('',#11255,#11299,#6030,.T.);
#13968=EDGE_CURVE('',#11300,#11299,#6031,.T.);
#13969=EDGE_CURVE('',#11256,#11300,#6032,.T.);
#13970=EDGE_CURVE('',#11301,#11300,#6033,.T.);
#13971=EDGE_CURVE('',#11257,#11301,#6034,.T.);
#13972=EDGE_CURVE('',#11302,#11301,#6035,.T.);
#13973=EDGE_CURVE('',#11258,#11302,#6036,.T.);
#13974=EDGE_CURVE('',#11303,#11302,#6037,.T.);
#13975=EDGE_CURVE('',#11259,#11303,#6038,.T.);
#13976=EDGE_CURVE('',#11304,#11303,#6039,.T.);
#13977=EDGE_CURVE('',#11260,#11304,#6040,.T.);
#13978=EDGE_CURVE('',#11305,#11304,#6041,.T.);
#13979=EDGE_CURVE('',#11261,#11305,#6042,.T.);
#13980=EDGE_CURVE('',#11306,#11305,#6043,.T.);
#13981=EDGE_CURVE('',#11262,#11306,#6044,.T.);
#13982=EDGE_CURVE('',#11307,#11306,#6045,.T.);
#13983=EDGE_CURVE('',#11263,#11307,#6046,.T.);
#13984=EDGE_CURVE('',#11308,#11307,#6047,.T.);
#13985=EDGE_CURVE('',#11264,#11308,#6048,.T.);
#13986=EDGE_CURVE('',#11266,#11308,#6049,.T.);
#13987=EDGE_CURVE('',#11101,#11309,#6050,.T.);
#13988=EDGE_CURVE('',#11309,#11310,#9818,.T.);
#13989=EDGE_CURVE('',#11310,#11098,#6051,.T.);
#13990=EDGE_CURVE('',#11311,#11312,#6052,.T.);
#13991=EDGE_CURVE('',#11313,#11311,#6053,.T.);
#13992=EDGE_CURVE('',#11314,#11313,#9819,.T.);
#13993=EDGE_CURVE('',#11315,#11314,#6054,.T.);
#13994=EDGE_CURVE('',#11316,#11315,#6055,.T.);
#13995=EDGE_CURVE('',#11317,#11316,#6056,.T.);
#13996=EDGE_CURVE('',#11318,#11317,#6057,.T.);
#13997=EDGE_CURVE('',#11319,#11318,#6058,.T.);
#13998=EDGE_CURVE('',#11319,#11320,#6059,.T.);
#13999=EDGE_CURVE('',#11320,#11321,#6060,.T.);
#14000=EDGE_CURVE('',#11321,#11322,#9820,.T.);
#14001=EDGE_CURVE('',#11322,#11323,#6061,.T.);
#14002=EDGE_CURVE('',#11323,#11324,#9821,.T.);
#14003=EDGE_CURVE('',#11324,#11325,#6062,.T.);
#14004=EDGE_CURVE('',#11325,#11326,#9822,.T.);
#14005=EDGE_CURVE('',#11326,#11327,#9823,.T.);
#14006=EDGE_CURVE('',#11327,#11328,#9824,.T.);
#14007=EDGE_CURVE('',#11328,#11329,#6063,.T.);
#14008=EDGE_CURVE('',#11329,#11330,#9825,.T.);
#14009=EDGE_CURVE('',#11330,#11331,#6064,.T.);
#14010=EDGE_CURVE('',#11331,#11332,#9826,.T.);
#14011=EDGE_CURVE('',#11332,#11333,#6065,.T.);
#14012=EDGE_CURVE('',#11333,#11334,#9827,.T.);
#14013=EDGE_CURVE('',#11334,#11335,#9828,.T.);
#14014=EDGE_CURVE('',#11335,#11336,#9829,.T.);
#14015=EDGE_CURVE('',#11336,#11337,#6066,.T.);
#14016=EDGE_CURVE('',#11337,#11338,#6067,.T.);
#14017=EDGE_CURVE('',#11338,#11339,#6068,.T.);
#14018=EDGE_CURVE('',#11339,#11340,#9830,.T.);
#14019=EDGE_CURVE('',#11340,#11341,#9831,.T.);
#14020=EDGE_CURVE('',#11341,#11342,#9832,.T.);
#14021=EDGE_CURVE('',#11342,#11343,#6069,.T.);
#14022=EDGE_CURVE('',#11343,#11344,#9833,.T.);
#14023=EDGE_CURVE('',#11344,#11345,#6070,.T.);
#14024=EDGE_CURVE('',#11345,#11346,#9834,.T.);
#14025=EDGE_CURVE('',#11346,#11347,#6071,.T.);
#14026=EDGE_CURVE('',#11347,#11348,#9835,.T.);
#14027=EDGE_CURVE('',#11348,#11349,#9836,.T.);
#14028=EDGE_CURVE('',#11349,#11350,#9837,.T.);
#14029=EDGE_CURVE('',#11350,#11351,#6072,.T.);
#14030=EDGE_CURVE('',#11351,#11352,#9838,.T.);
#14031=EDGE_CURVE('',#11352,#11353,#6073,.T.);
#14032=EDGE_CURVE('',#11353,#11354,#9839,.T.);
#14033=EDGE_CURVE('',#11354,#11355,#6074,.T.);
#14034=EDGE_CURVE('',#11355,#11356,#6075,.T.);
#14035=EDGE_CURVE('',#11357,#11356,#6076,.T.);
#14036=EDGE_CURVE('',#11358,#11357,#6077,.T.);
#14037=EDGE_CURVE('',#11312,#11358,#6078,.T.);
#14038=EDGE_CURVE('',#11359,#11099,#6079,.T.);
#14039=EDGE_CURVE('',#11310,#11359,#6080,.T.);
#14040=EDGE_CURVE('',#11100,#11360,#6081,.T.);
#14041=EDGE_CURVE('',#11309,#11360,#6082,.T.);
#14042=EDGE_CURVE('',#11360,#11359,#9840,.T.);
#14043=EDGE_CURVE('',#11091,#11361,#6083,.T.);
#14044=EDGE_CURVE('',#11361,#11362,#9841,.T.);
#14045=EDGE_CURVE('',#11362,#11092,#6084,.T.);
#14046=EDGE_CURVE('',#11363,#11364,#6085,.T.);
#14047=EDGE_CURVE('',#11364,#11356,#6086,.T.);
#14048=EDGE_CURVE('',#11363,#11355,#6087,.T.);
#14049=EDGE_CURVE('',#11364,#11365,#6088,.T.);
#14050=EDGE_CURVE('',#11365,#11357,#6089,.T.);
#14051=EDGE_CURVE('',#11365,#11366,#6090,.T.);
#14052=EDGE_CURVE('',#11366,#11358,#6091,.T.);
#14053=EDGE_CURVE('',#11366,#11367,#6092,.T.);
#14054=EDGE_CURVE('',#11367,#11312,#6093,.T.);
#14055=EDGE_CURVE('',#11368,#11369,#6094,.T.);
#14056=EDGE_CURVE('',#11368,#11311,#6095,.T.);
#14057=EDGE_CURVE('',#11367,#11370,#6096,.T.);
#14058=EDGE_CURVE('',#11370,#11316,#6097,.T.);
#14059=EDGE_CURVE('',#11369,#11315,#6098,.T.);
#14060=EDGE_CURVE('',#11370,#11371,#6099,.T.);
#14061=EDGE_CURVE('',#11371,#11317,#6100,.T.);
#14062=EDGE_CURVE('',#11371,#11372,#6101,.T.);
#14063=EDGE_CURVE('',#11372,#11318,#6102,.T.);
#14064=EDGE_CURVE('',#11372,#11373,#6103,.T.);
#14065=EDGE_CURVE('',#11373,#11319,#6104,.T.);
#14066=EDGE_CURVE('',#11373,#11374,#6105,.T.);
#14067=EDGE_CURVE('',#11374,#11320,#6106,.T.);
#14068=EDGE_CURVE('',#11374,#11375,#6107,.T.);
#14069=EDGE_CURVE('',#11375,#11321,#6108,.T.);
#14070=EDGE_CURVE('',#11375,#11376,#9842,.T.);
#14071=EDGE_CURVE('',#11322,#11376,#6109,.T.);
#14072=EDGE_CURVE('',#11376,#11377,#6110,.T.);
#14073=EDGE_CURVE('',#11377,#11323,#6111,.T.);
#14074=EDGE_CURVE('',#11377,#11378,#9843,.T.);
#14075=EDGE_CURVE('',#11324,#11378,#6112,.T.);
#14076=EDGE_CURVE('',#11378,#11379,#6113,.T.);
#14077=EDGE_CURVE('',#11379,#11325,#6114,.T.);
#14078=EDGE_CURVE('',#11379,#11380,#9844,.T.);
#14079=EDGE_CURVE('',#11326,#11380,#6115,.T.);
#14080=EDGE_CURVE('',#11380,#11381,#9845,.T.);
#14081=EDGE_CURVE('',#11381,#11327,#6116,.T.);
#14082=EDGE_CURVE('',#11381,#11382,#9846,.T.);
#14083=EDGE_CURVE('',#11328,#11382,#6117,.T.);
#14084=EDGE_CURVE('',#11382,#11383,#6118,.T.);
#14085=EDGE_CURVE('',#11383,#11329,#6119,.T.);
#14086=EDGE_CURVE('',#11383,#11384,#9847,.T.);
#14087=EDGE_CURVE('',#11330,#11384,#6120,.T.);
#14088=EDGE_CURVE('',#11384,#11385,#6121,.T.);
#14089=EDGE_CURVE('',#11385,#11331,#6122,.T.);
#14090=EDGE_CURVE('',#11385,#11386,#9848,.T.);
#14091=EDGE_CURVE('',#11332,#11386,#6123,.T.);
#14092=EDGE_CURVE('',#11386,#11387,#6124,.T.);
#14093=EDGE_CURVE('',#11387,#11333,#6125,.T.);
#14094=EDGE_CURVE('',#11387,#11388,#9849,.T.);
#14095=EDGE_CURVE('',#11334,#11388,#6126,.T.);
#14096=EDGE_CURVE('',#11388,#11389,#9850,.T.);
#14097=EDGE_CURVE('',#11389,#11335,#6127,.T.);
#14098=EDGE_CURVE('',#11389,#11390,#9851,.T.);
#14099=EDGE_CURVE('',#11336,#11390,#6128,.T.);
#14100=EDGE_CURVE('',#11390,#11391,#6129,.T.);
#14101=EDGE_CURVE('',#11391,#11337,#6130,.T.);
#14102=EDGE_CURVE('',#11391,#11392,#6131,.T.);
#14103=EDGE_CURVE('',#11392,#11338,#6132,.T.);
#14104=EDGE_CURVE('',#11392,#11393,#6133,.T.);
#14105=EDGE_CURVE('',#11393,#11339,#6134,.T.);
#14106=EDGE_CURVE('',#11393,#11394,#9852,.T.);
#14107=EDGE_CURVE('',#11340,#11394,#6135,.T.);
#14108=EDGE_CURVE('',#11394,#11395,#9853,.T.);
#14109=EDGE_CURVE('',#11395,#11341,#6136,.T.);
#14110=EDGE_CURVE('',#11395,#11396,#9854,.T.);
#14111=EDGE_CURVE('',#11342,#11396,#6137,.T.);
#14112=EDGE_CURVE('',#11396,#11397,#6138,.T.);
#14113=EDGE_CURVE('',#11397,#11343,#6139,.T.);
#14114=EDGE_CURVE('',#11397,#11398,#9855,.T.);
#14115=EDGE_CURVE('',#11344,#11398,#6140,.T.);
#14116=EDGE_CURVE('',#11398,#11399,#6141,.T.);
#14117=EDGE_CURVE('',#11399,#11345,#6142,.T.);
#14118=EDGE_CURVE('',#11399,#11400,#9856,.T.);
#14119=EDGE_CURVE('',#11346,#11400,#6143,.T.);
#14120=EDGE_CURVE('',#11400,#11401,#6144,.T.);
#14121=EDGE_CURVE('',#11401,#11347,#6145,.T.);
#14122=EDGE_CURVE('',#11401,#11402,#9857,.T.);
#14123=EDGE_CURVE('',#11348,#11402,#6146,.T.);
#14124=EDGE_CURVE('',#11402,#11403,#9858,.T.);
#14125=EDGE_CURVE('',#11403,#11349,#6147,.T.);
#14126=EDGE_CURVE('',#11403,#11404,#9859,.T.);
#14127=EDGE_CURVE('',#11350,#11404,#6148,.T.);
#14128=EDGE_CURVE('',#11404,#11405,#6149,.T.);
#14129=EDGE_CURVE('',#11405,#11351,#6150,.T.);
#14130=EDGE_CURVE('',#11405,#11406,#9860,.T.);
#14131=EDGE_CURVE('',#11352,#11406,#6151,.T.);
#14132=EDGE_CURVE('',#11406,#11407,#6152,.T.);
#14133=EDGE_CURVE('',#11407,#11353,#6153,.T.);
#14134=EDGE_CURVE('',#11407,#11408,#9861,.T.);
#14135=EDGE_CURVE('',#11354,#11408,#6154,.T.);
#14136=EDGE_CURVE('',#11408,#11363,#6155,.T.);
#14137=EDGE_CURVE('',#11409,#11410,#6156,.T.);
#14138=EDGE_CURVE('',#11410,#11411,#6157,.T.);
#14139=EDGE_CURVE('',#11411,#11412,#6158,.T.);
#14140=EDGE_CURVE('',#11412,#11409,#6159,.T.);
#14141=EDGE_CURVE('',#11413,#11414,#6160,.T.);
#14142=EDGE_CURVE('',#11414,#11415,#6161,.T.);
#14143=EDGE_CURVE('',#11415,#11416,#6162,.T.);
#14144=EDGE_CURVE('',#11413,#11416,#6163,.T.);
#14145=EDGE_CURVE('',#11417,#11093,#6164,.T.);
#14146=EDGE_CURVE('',#11362,#11417,#6165,.T.);
#14147=EDGE_CURVE('',#11094,#11418,#6166,.T.);
#14148=EDGE_CURVE('',#11361,#11418,#6167,.T.);
#14149=EDGE_CURVE('',#11418,#11417,#9862,.T.);
#14150=EDGE_CURVE('',#11410,#11419,#9863,.T.);
#14151=EDGE_CURVE('',#11420,#11409,#9864,.T.);
#14152=EDGE_CURVE('',#11419,#11420,#6168,.T.);
#14153=EDGE_CURVE('',#11421,#11419,#6169,.T.);
#14154=EDGE_CURVE('',#11421,#11422,#6170,.T.);
#14155=EDGE_CURVE('',#11422,#11423,#6171,.T.);
#14156=EDGE_CURVE('',#11411,#11423,#6172,.T.);
#14157=EDGE_CURVE('',#11421,#11424,#6173,.T.);
#14158=EDGE_CURVE('',#11424,#11425,#6174,.T.);
#14159=EDGE_CURVE('',#11422,#11425,#6175,.T.);
#14160=EDGE_CURVE('',#11426,#11427,#6176,.T.);
#14161=EDGE_CURVE('',#11427,#11428,#6177,.T.);
#14162=EDGE_CURVE('',#11428,#11429,#6178,.T.);
#14163=EDGE_CURVE('',#11426,#11429,#6179,.T.);
#14164=EDGE_CURVE('',#11430,#11429,#6180,.T.);
#14165=EDGE_CURVE('',#11430,#11415,#9865,.T.);
#14166=EDGE_CURVE('',#11431,#11414,#6181,.T.);
#14167=EDGE_CURVE('',#11431,#11426,#6182,.T.);
#14168=EDGE_CURVE('',#11432,#11430,#6183,.T.);
#14169=EDGE_CURVE('',#11432,#11416,#9866,.T.);
#14170=EDGE_CURVE('',#11433,#11434,#6184,.T.);
#14171=EDGE_CURVE('',#11434,#11435,#6185,.T.);
#14172=EDGE_CURVE('',#11435,#11436,#6186,.T.);
#14173=EDGE_CURVE('',#11436,#11437,#6187,.T.);
#14174=EDGE_CURVE('',#11437,#11438,#6188,.T.);
#14175=EDGE_CURVE('',#11438,#11439,#6189,.T.);
#14176=EDGE_CURVE('',#11439,#11440,#6190,.T.);
#14177=EDGE_CURVE('',#11440,#11441,#6191,.T.);
#14178=EDGE_CURVE('',#11441,#11442,#6192,.T.);
#14179=EDGE_CURVE('',#11442,#11443,#6193,.T.);
#14180=EDGE_CURVE('',#11443,#11444,#9867,.T.);
#14181=EDGE_CURVE('',#11444,#11445,#6194,.T.);
#14182=EDGE_CURVE('',#11445,#11446,#9868,.T.);
#14183=EDGE_CURVE('',#11446,#11447,#6195,.T.);
#14184=EDGE_CURVE('',#11447,#11448,#9869,.T.);
#14185=EDGE_CURVE('',#11448,#11449,#9870,.T.);
#14186=EDGE_CURVE('',#11449,#11450,#9871,.T.);
#14187=EDGE_CURVE('',#11450,#11451,#6196,.T.);
#14188=EDGE_CURVE('',#11451,#11452,#9872,.T.);
#14189=EDGE_CURVE('',#11452,#11453,#6197,.T.);
#14190=EDGE_CURVE('',#11453,#11454,#9873,.T.);
#14191=EDGE_CURVE('',#11454,#11455,#6198,.T.);
#14192=EDGE_CURVE('',#11455,#11456,#9874,.T.);
#14193=EDGE_CURVE('',#11456,#11457,#9875,.T.);
#14194=EDGE_CURVE('',#11457,#11458,#9876,.T.);
#14195=EDGE_CURVE('',#11458,#11459,#6199,.T.);
#14196=EDGE_CURVE('',#11459,#11460,#6200,.T.);
#14197=EDGE_CURVE('',#11460,#11461,#6201,.T.);
#14198=EDGE_CURVE('',#11461,#11462,#9877,.T.);
#14199=EDGE_CURVE('',#11462,#11463,#9878,.T.);
#14200=EDGE_CURVE('',#11463,#11464,#9879,.T.);
#14201=EDGE_CURVE('',#11464,#11465,#6202,.T.);
#14202=EDGE_CURVE('',#11465,#11466,#9880,.T.);
#14203=EDGE_CURVE('',#11466,#11467,#6203,.T.);
#14204=EDGE_CURVE('',#11467,#11468,#9881,.T.);
#14205=EDGE_CURVE('',#11468,#11469,#6204,.T.);
#14206=EDGE_CURVE('',#11469,#11470,#9882,.T.);
#14207=EDGE_CURVE('',#11470,#11471,#9883,.T.);
#14208=EDGE_CURVE('',#11471,#11472,#9884,.T.);
#14209=EDGE_CURVE('',#11472,#11473,#6205,.T.);
#14210=EDGE_CURVE('',#11473,#11474,#9885,.T.);
#14211=EDGE_CURVE('',#11474,#11475,#6206,.T.);
#14212=EDGE_CURVE('',#11475,#11476,#9886,.T.);
#14213=EDGE_CURVE('',#11476,#11433,#6207,.T.);
#14214=EDGE_CURVE('',#11431,#11477,#6208,.T.);
#14215=EDGE_CURVE('',#11477,#11413,#6209,.T.);
#14216=EDGE_CURVE('',#11478,#11423,#6210,.T.);
#14217=EDGE_CURVE('',#11478,#11412,#6211,.T.);
#14218=EDGE_CURVE('',#11479,#11480,#6212,.T.);
#14219=EDGE_CURVE('',#11420,#11480,#6213,.T.);
#14220=EDGE_CURVE('',#11478,#11479,#6214,.T.);
#14221=EDGE_CURVE('',#11479,#11481,#6215,.T.);
#14222=EDGE_CURVE('',#11481,#11482,#6216,.T.);
#14223=EDGE_CURVE('',#11482,#11480,#6217,.T.);
#14224=EDGE_CURVE('',#11483,#11477,#6218,.T.);
#14225=EDGE_CURVE('',#11432,#11484,#6219,.T.);
#14226=EDGE_CURVE('',#11484,#11483,#6220,.T.);
#14227=EDGE_CURVE('',#11484,#11485,#6221,.T.);
#14228=EDGE_CURVE('',#11485,#11486,#6222,.T.);
#14229=EDGE_CURVE('',#11483,#11486,#6223,.T.);
#14230=EDGE_CURVE('',#11121,#11482,#648,.T.);
#14231=EDGE_CURVE('',#11424,#11123,#649,.T.);
#14232=EDGE_CURVE('',#11487,#11427,#9887,.T.);
#14233=EDGE_CURVE('',#11488,#11431,#6224,.T.);
#14234=EDGE_CURVE('',#11488,#11489,#6225,.T.);
#14235=EDGE_CURVE('',#11487,#11489,#6226,.T.);
#14236=EDGE_CURVE('',#11490,#11491,#6227,.T.);
#14237=EDGE_CURVE('',#11491,#11487,#6228,.T.);
#14238=EDGE_CURVE('',#11489,#11490,#6229,.T.);
#14239=EDGE_CURVE('',#11124,#11492,#650,.T.);
#14240=EDGE_CURVE('',#11493,#11126,#6230,.T.);
#14241=EDGE_CURVE('',#11492,#11493,#6231,.T.);
#14242=EDGE_CURVE('',#11494,#11495,#6232,.T.);
#14243=EDGE_CURVE('',#11494,#11492,#6233,.T.);
#14244=EDGE_CURVE('',#11493,#11495,#6234,.T.);
#14245=EDGE_CURVE('',#11495,#11496,#6235,.T.);
#14246=EDGE_CURVE('',#11423,#11496,#6236,.T.);
#14247=EDGE_CURVE('',#11425,#11494,#9888,.T.);
#14248=EDGE_CURVE('',#11491,#11497,#651,.T.);
#14249=EDGE_CURVE('',#11498,#11490,#6237,.T.);
#14250=EDGE_CURVE('',#11497,#11498,#6238,.T.);
#14251=EDGE_CURVE('',#11485,#11117,#652,.T.);
#14252=EDGE_CURVE('',#11118,#11428,#653,.T.);
#14253=EDGE_CURVE('',#11499,#11500,#6239,.T.);
#14254=EDGE_CURVE('',#11434,#11500,#6240,.T.);
#14255=EDGE_CURVE('',#11433,#11499,#6241,.T.);
#14256=EDGE_CURVE('',#11500,#11501,#6242,.T.);
#14257=EDGE_CURVE('',#11435,#11501,#6243,.T.);
#14258=EDGE_CURVE('',#11501,#11502,#6244,.T.);
#14259=EDGE_CURVE('',#11436,#11502,#6245,.T.);
#14260=EDGE_CURVE('',#11502,#11503,#6246,.T.);
#14261=EDGE_CURVE('',#11437,#11503,#6247,.T.);
#14262=EDGE_CURVE('',#11503,#11504,#6248,.T.);
#14263=EDGE_CURVE('',#11438,#11504,#6249,.T.);
#14264=EDGE_CURVE('',#11504,#11505,#6250,.T.);
#14265=EDGE_CURVE('',#11439,#11505,#6251,.T.);
#14266=EDGE_CURVE('',#11505,#11506,#6252,.T.);
#14267=EDGE_CURVE('',#11440,#11506,#6253,.T.);
#14268=EDGE_CURVE('',#11506,#11507,#6254,.T.);
#14269=EDGE_CURVE('',#11441,#11507,#6255,.T.);
#14270=EDGE_CURVE('',#11507,#11508,#6256,.T.);
#14271=EDGE_CURVE('',#11442,#11508,#6257,.T.);
#14272=EDGE_CURVE('',#11508,#11509,#6258,.T.);
#14273=EDGE_CURVE('',#11443,#11509,#6259,.T.);
#14274=EDGE_CURVE('',#11509,#11510,#9889,.T.);
#14275=EDGE_CURVE('',#11444,#11510,#6260,.T.);
#14276=EDGE_CURVE('',#11510,#11511,#6261,.T.);
#14277=EDGE_CURVE('',#11445,#11511,#6262,.T.);
#14278=EDGE_CURVE('',#11511,#11512,#9890,.T.);
#14279=EDGE_CURVE('',#11446,#11512,#6263,.T.);
#14280=EDGE_CURVE('',#11512,#11513,#6264,.T.);
#14281=EDGE_CURVE('',#11447,#11513,#6265,.T.);
#14282=EDGE_CURVE('',#11513,#11514,#9891,.T.);
#14283=EDGE_CURVE('',#11448,#11514,#6266,.T.);
#14284=EDGE_CURVE('',#11514,#11515,#9892,.T.);
#14285=EDGE_CURVE('',#11449,#11515,#6267,.T.);
#14286=EDGE_CURVE('',#11515,#11516,#9893,.T.);
#14287=EDGE_CURVE('',#11450,#11516,#6268,.T.);
#14288=EDGE_CURVE('',#11516,#11517,#6269,.T.);
#14289=EDGE_CURVE('',#11451,#11517,#6270,.T.);
#14290=EDGE_CURVE('',#11517,#11518,#9894,.T.);
#14291=EDGE_CURVE('',#11452,#11518,#6271,.T.);
#14292=EDGE_CURVE('',#11518,#11519,#6272,.T.);
#14293=EDGE_CURVE('',#11453,#11519,#6273,.T.);
#14294=EDGE_CURVE('',#11519,#11520,#9895,.T.);
#14295=EDGE_CURVE('',#11454,#11520,#6274,.T.);
#14296=EDGE_CURVE('',#11520,#11521,#6275,.T.);
#14297=EDGE_CURVE('',#11455,#11521,#6276,.T.);
#14298=EDGE_CURVE('',#11521,#11522,#9896,.T.);
#14299=EDGE_CURVE('',#11456,#11522,#6277,.T.);
#14300=EDGE_CURVE('',#11522,#11523,#9897,.T.);
#14301=EDGE_CURVE('',#11457,#11523,#6278,.T.);
#14302=EDGE_CURVE('',#11523,#11524,#9898,.T.);
#14303=EDGE_CURVE('',#11458,#11524,#6279,.T.);
#14304=EDGE_CURVE('',#11524,#11525,#6280,.T.);
#14305=EDGE_CURVE('',#11459,#11525,#6281,.T.);
#14306=EDGE_CURVE('',#11525,#11526,#6282,.T.);
#14307=EDGE_CURVE('',#11460,#11526,#6283,.T.);
#14308=EDGE_CURVE('',#11526,#11527,#6284,.T.);
#14309=EDGE_CURVE('',#11461,#11527,#6285,.T.);
#14310=EDGE_CURVE('',#11527,#11528,#9899,.T.);
#14311=EDGE_CURVE('',#11462,#11528,#6286,.T.);
#14312=EDGE_CURVE('',#11528,#11529,#9900,.T.);
#14313=EDGE_CURVE('',#11463,#11529,#6287,.T.);
#14314=EDGE_CURVE('',#11529,#11530,#9901,.T.);
#14315=EDGE_CURVE('',#11464,#11530,#6288,.T.);
#14316=EDGE_CURVE('',#11530,#11531,#6289,.T.);
#14317=EDGE_CURVE('',#11465,#11531,#6290,.T.);
#14318=EDGE_CURVE('',#11531,#11532,#9902,.T.);
#14319=EDGE_CURVE('',#11466,#11532,#6291,.T.);
#14320=EDGE_CURVE('',#11532,#11533,#6292,.T.);
#14321=EDGE_CURVE('',#11467,#11533,#6293,.T.);
#14322=EDGE_CURVE('',#11533,#11534,#9903,.T.);
#14323=EDGE_CURVE('',#11468,#11534,#6294,.T.);
#14324=EDGE_CURVE('',#11534,#11535,#6295,.T.);
#14325=EDGE_CURVE('',#11469,#11535,#6296,.T.);
#14326=EDGE_CURVE('',#11535,#11536,#9904,.T.);
#14327=EDGE_CURVE('',#11470,#11536,#6297,.T.);
#14328=EDGE_CURVE('',#11536,#11537,#9905,.T.);
#14329=EDGE_CURVE('',#11471,#11537,#6298,.T.);
#14330=EDGE_CURVE('',#11537,#11538,#9906,.T.);
#14331=EDGE_CURVE('',#11472,#11538,#6299,.T.);
#14332=EDGE_CURVE('',#11538,#11539,#6300,.T.);
#14333=EDGE_CURVE('',#11473,#11539,#6301,.T.);
#14334=EDGE_CURVE('',#11539,#11540,#9907,.T.);
#14335=EDGE_CURVE('',#11474,#11540,#6302,.T.);
#14336=EDGE_CURVE('',#11540,#11541,#6303,.T.);
#14337=EDGE_CURVE('',#11475,#11541,#6304,.T.);
#14338=EDGE_CURVE('',#11541,#11542,#9908,.T.);
#14339=EDGE_CURVE('',#11476,#11542,#6305,.T.);
#14340=EDGE_CURVE('',#11542,#11499,#6306,.T.);
#14341=EDGE_CURVE('',#11543,#11544,#6307,.T.);
#14342=EDGE_CURVE('',#11544,#11545,#6308,.T.);
#14343=EDGE_CURVE('',#11545,#11546,#6309,.T.);
#14344=EDGE_CURVE('',#11546,#11543,#6310,.T.);
#14345=EDGE_CURVE('',#11547,#11544,#6311,.T.);
#14346=EDGE_CURVE('',#11547,#11548,#6312,.T.);
#14347=EDGE_CURVE('',#11545,#11548,#6313,.T.);
#14348=EDGE_CURVE('',#11549,#11547,#6314,.T.);
#14349=EDGE_CURVE('',#11550,#11549,#6315,.T.);
#14350=EDGE_CURVE('',#11548,#11550,#6316,.T.);
#14351=EDGE_CURVE('',#11551,#11549,#6317,.T.);
#14352=EDGE_CURVE('',#11552,#11551,#6318,.T.);
#14353=EDGE_CURVE('',#11550,#11552,#6319,.T.);
#14354=EDGE_CURVE('',#11553,#11551,#6320,.T.);
#14355=EDGE_CURVE('',#11554,#11553,#6321,.T.);
#14356=EDGE_CURVE('',#11552,#11554,#6322,.T.);
#14357=EDGE_CURVE('',#11555,#11556,#6323,.T.);
#14358=EDGE_CURVE('',#11557,#11555,#6324,.T.);
#14359=EDGE_CURVE('',#11558,#11557,#6325,.T.);
#14360=EDGE_CURVE('',#11558,#11556,#6326,.T.);
#14361=EDGE_CURVE('',#11559,#11555,#6327,.T.);
#14362=EDGE_CURVE('',#11560,#11559,#6328,.T.);
#14363=EDGE_CURVE('',#11557,#11560,#6329,.T.);
#14364=EDGE_CURVE('',#11561,#11559,#6330,.T.);
#14365=EDGE_CURVE('',#11562,#11561,#6331,.T.);
#14366=EDGE_CURVE('',#11560,#11562,#6332,.T.);
#14367=EDGE_CURVE('',#11562,#11546,#6333,.T.);
#14368=EDGE_CURVE('',#11543,#11561,#6334,.T.);
#14369=EDGE_CURVE('',#11488,#11563,#6335,.T.);
#14370=EDGE_CURVE('',#11477,#11564,#6336,.T.);
#14371=EDGE_CURVE('',#11564,#11565,#6337,.T.);
#14372=EDGE_CURVE('',#11565,#11563,#6338,.T.);
#14373=EDGE_CURVE('',#11565,#11566,#6339,.T.);
#14374=EDGE_CURVE('',#11566,#11567,#6340,.T.);
#14375=EDGE_CURVE('',#11563,#11567,#6341,.T.);
#14376=EDGE_CURVE('',#11568,#11569,#6342,.T.);
#14377=EDGE_CURVE('',#11567,#11569,#6343,.T.);
#14378=EDGE_CURVE('',#11566,#11568,#6344,.T.);
#14379=EDGE_CURVE('',#11570,#11571,#6345,.T.);
#14380=EDGE_CURVE('',#11571,#11569,#6346,.T.);
#14381=EDGE_CURVE('',#11570,#11568,#6347,.T.);
#14382=EDGE_CURVE('',#11572,#11573,#6348,.T.);
#14383=EDGE_CURVE('',#11573,#11571,#6349,.T.);
#14384=EDGE_CURVE('',#11572,#11570,#6350,.T.);
#14385=EDGE_CURVE('',#11574,#11575,#6351,.T.);
#14386=EDGE_CURVE('',#11575,#11573,#6352,.T.);
#14387=EDGE_CURVE('',#11574,#11572,#6353,.T.);
#14388=EDGE_CURVE('',#11574,#11576,#6354,.T.);
#14389=EDGE_CURVE('',#11576,#11577,#6355,.T.);
#14390=EDGE_CURVE('',#11575,#11577,#6356,.T.);
#14391=EDGE_CURVE('',#11578,#11579,#6357,.T.);
#14392=EDGE_CURVE('',#11579,#11577,#6358,.T.);
#14393=EDGE_CURVE('',#11578,#11576,#6359,.T.);
#14394=EDGE_CURVE('',#11580,#11581,#6360,.T.);
#14395=EDGE_CURVE('',#11581,#11579,#6361,.T.);
#14396=EDGE_CURVE('',#11580,#11578,#6362,.T.);
#14397=EDGE_CURVE('',#11582,#11583,#6363,.T.);
#14398=EDGE_CURVE('',#11583,#11581,#6364,.T.);
#14399=EDGE_CURVE('',#11582,#11580,#6365,.T.);
#14400=EDGE_CURVE('',#11582,#11584,#6366,.T.);
#14401=EDGE_CURVE('',#11584,#11585,#6367,.T.);
#14402=EDGE_CURVE('',#11583,#11585,#6368,.T.);
#14403=EDGE_CURVE('',#11584,#11586,#6369,.T.);
#14404=EDGE_CURVE('',#11586,#11587,#6370,.T.);
#14405=EDGE_CURVE('',#11585,#11587,#6371,.T.);
#14406=EDGE_CURVE('',#11586,#11588,#6372,.T.);
#14407=EDGE_CURVE('',#11588,#11589,#6373,.T.);
#14408=EDGE_CURVE('',#11587,#11589,#6374,.T.);
#14409=EDGE_CURVE('',#11588,#11590,#6375,.T.);
#14410=EDGE_CURVE('',#11590,#11591,#6376,.T.);
#14411=EDGE_CURVE('',#11589,#11591,#6377,.T.);
#14412=EDGE_CURVE('',#11590,#11592,#6378,.T.);
#14413=EDGE_CURVE('',#11592,#11478,#6379,.T.);
#14414=EDGE_CURVE('',#11591,#11496,#6380,.T.);
#14415=EDGE_CURVE('',#11593,#11481,#9909,.T.);
#14416=EDGE_CURVE('',#11592,#11594,#6381,.T.);
#14417=EDGE_CURVE('',#11593,#11594,#6382,.T.);
#14418=EDGE_CURVE('',#11595,#11596,#6383,.T.);
#14419=EDGE_CURVE('',#11596,#11593,#6384,.T.);
#14420=EDGE_CURVE('',#11594,#11595,#6385,.T.);
#14421=EDGE_CURVE('',#11596,#11597,#654,.T.);
#14422=EDGE_CURVE('',#11595,#11598,#6386,.T.);
#14423=EDGE_CURVE('',#11598,#11597,#6387,.T.);
#14424=EDGE_CURVE('',#11114,#11599,#655,.T.);
#14425=EDGE_CURVE('',#11116,#11600,#6388,.T.);
#14426=EDGE_CURVE('',#11599,#11600,#6389,.T.);
#14427=EDGE_CURVE('',#11601,#11602,#6390,.T.);
#14428=EDGE_CURVE('',#11601,#11599,#6391,.T.);
#14429=EDGE_CURVE('',#11600,#11602,#6392,.T.);
#14430=EDGE_CURVE('',#11602,#11564,#6393,.T.);
#14431=EDGE_CURVE('',#11486,#11601,#9910,.T.);
#14432=EDGE_CURVE('',#11597,#11120,#656,.T.);
#14433=EDGE_CURVE('',#11598,#11603,#6394,.T.);
#14434=EDGE_CURVE('',#11603,#11120,#6395,.T.);
#14435=EDGE_CURVE('',#11556,#11604,#6396,.T.);
#14436=EDGE_CURVE('',#11605,#11558,#6397,.T.);
#14437=EDGE_CURVE('',#11605,#11604,#6398,.T.);
#14438=EDGE_CURVE('',#11606,#11553,#6399,.T.);
#14439=EDGE_CURVE('',#11607,#11606,#6400,.T.);
#14440=EDGE_CURVE('',#11554,#11607,#6401,.T.);
#14441=EDGE_CURVE('',#11125,#11605,#6402,.T.);
#14442=EDGE_CURVE('',#11607,#11608,#6403,.T.);
#14443=EDGE_CURVE('',#11608,#11498,#6404,.T.);
#14444=EDGE_CURVE('',#11497,#11119,#657,.T.);
#14445=EDGE_CURVE('',#11119,#11608,#6405,.T.);
#14446=EDGE_CURVE('',#11604,#11609,#6406,.T.);
#14447=EDGE_CURVE('',#11609,#11610,#6407,.T.);
#14448=EDGE_CURVE('',#11610,#11611,#9911,.T.);
#14449=EDGE_CURVE('',#11611,#11612,#6408,.T.);
#14450=EDGE_CURVE('',#11612,#11613,#9912,.T.);
#14451=EDGE_CURVE('',#11613,#11614,#6409,.T.);
#14452=EDGE_CURVE('',#11614,#11615,#9913,.T.);
#14453=EDGE_CURVE('',#11615,#11616,#9914,.T.);
#14454=EDGE_CURVE('',#11616,#11617,#9915,.T.);
#14455=EDGE_CURVE('',#11617,#11618,#6410,.T.);
#14456=EDGE_CURVE('',#11618,#11619,#9916,.T.);
#14457=EDGE_CURVE('',#11619,#11620,#6411,.T.);
#14458=EDGE_CURVE('',#11620,#11621,#9917,.T.);
#14459=EDGE_CURVE('',#11621,#11622,#6412,.T.);
#14460=EDGE_CURVE('',#11622,#11623,#9918,.T.);
#14461=EDGE_CURVE('',#11623,#11624,#9919,.T.);
#14462=EDGE_CURVE('',#11624,#11625,#9920,.T.);
#14463=EDGE_CURVE('',#11625,#11626,#6413,.T.);
#14464=EDGE_CURVE('',#11626,#11627,#6414,.T.);
#14465=EDGE_CURVE('',#11627,#11628,#6415,.T.);
#14466=EDGE_CURVE('',#11628,#11629,#9921,.T.);
#14467=EDGE_CURVE('',#11629,#11630,#9922,.T.);
#14468=EDGE_CURVE('',#11630,#11631,#9923,.T.);
#14469=EDGE_CURVE('',#11631,#11632,#6416,.T.);
#14470=EDGE_CURVE('',#11632,#11633,#9924,.T.);
#14471=EDGE_CURVE('',#11633,#11634,#6417,.T.);
#14472=EDGE_CURVE('',#11634,#11635,#9925,.T.);
#14473=EDGE_CURVE('',#11635,#11636,#6418,.T.);
#14474=EDGE_CURVE('',#11636,#11637,#9926,.T.);
#14475=EDGE_CURVE('',#11637,#11638,#9927,.T.);
#14476=EDGE_CURVE('',#11638,#11639,#9928,.T.);
#14477=EDGE_CURVE('',#11639,#11640,#6419,.T.);
#14478=EDGE_CURVE('',#11640,#11641,#9929,.T.);
#14479=EDGE_CURVE('',#11641,#11642,#6420,.T.);
#14480=EDGE_CURVE('',#11642,#11643,#9930,.T.);
#14481=EDGE_CURVE('',#11643,#11644,#6421,.T.);
#14482=EDGE_CURVE('',#11644,#11606,#6422,.T.);
#14483=EDGE_CURVE('',#11645,#11115,#6423,.T.);
#14484=EDGE_CURVE('',#11646,#11645,#6424,.T.);
#14485=EDGE_CURVE('',#11647,#11646,#6425,.T.);
#14486=EDGE_CURVE('',#11648,#11647,#6426,.T.);
#14487=EDGE_CURVE('',#11649,#11648,#6427,.T.);
#14488=EDGE_CURVE('',#11649,#11650,#6428,.T.);
#14489=EDGE_CURVE('',#11651,#11650,#6429,.T.);
#14490=EDGE_CURVE('',#11651,#11652,#6430,.T.);
#14491=EDGE_CURVE('',#11653,#11652,#6431,.T.);
#14492=EDGE_CURVE('',#11654,#11653,#6432,.T.);
#14493=EDGE_CURVE('',#11655,#11654,#6433,.T.);
#14494=EDGE_CURVE('',#11656,#11655,#6434,.T.);
#14495=EDGE_CURVE('',#11603,#11656,#6435,.T.);
#14496=EDGE_CURVE('',#11657,#11658,#6436,.T.);
#14497=EDGE_CURVE('',#11657,#11652,#6437,.T.);
#14498=EDGE_CURVE('',#11658,#11651,#6438,.T.);
#14499=EDGE_CURVE('',#11659,#11660,#6439,.T.);
#14500=EDGE_CURVE('',#11660,#11648,#6440,.T.);
#14501=EDGE_CURVE('',#11659,#11647,#6441,.T.);
#14502=EDGE_CURVE('',#11661,#11659,#6442,.T.);
#14503=EDGE_CURVE('',#11661,#11646,#6443,.T.);
#14504=EDGE_CURVE('',#11662,#11661,#6444,.T.);
#14505=EDGE_CURVE('',#11662,#11645,#6445,.T.);
#14506=EDGE_CURVE('',#11660,#11663,#6446,.T.);
#14507=EDGE_CURVE('',#11649,#11663,#6447,.T.);
#14508=EDGE_CURVE('',#11664,#11642,#6448,.T.);
#14509=EDGE_CURVE('',#11664,#11665,#9931,.T.);
#14510=EDGE_CURVE('',#11643,#11665,#6449,.T.);
#14511=EDGE_CURVE('',#11666,#11640,#6450,.T.);
#14512=EDGE_CURVE('',#11666,#11667,#9932,.T.);
#14513=EDGE_CURVE('',#11641,#11667,#6451,.T.);
#14514=EDGE_CURVE('',#11667,#11664,#6452,.T.);
#14515=EDGE_CURVE('',#11665,#11668,#6453,.T.);
#14516=EDGE_CURVE('',#11668,#11644,#6454,.T.);
#14517=EDGE_CURVE('',#11668,#11662,#6455,.T.);
#14518=EDGE_CURVE('',#11669,#11670,#9933,.T.);
#14519=EDGE_CURVE('',#11639,#11670,#6456,.T.);
#14520=EDGE_CURVE('',#11669,#11638,#6457,.T.);
#14521=EDGE_CURVE('',#11671,#11672,#9934,.T.);
#14522=EDGE_CURVE('',#11637,#11672,#6458,.T.);
#14523=EDGE_CURVE('',#11671,#11636,#6459,.T.);
#14524=EDGE_CURVE('',#11672,#11669,#9935,.T.);
#14525=EDGE_CURVE('',#11673,#11674,#9936,.T.);
#14526=EDGE_CURVE('',#11635,#11674,#6460,.T.);
#14527=EDGE_CURVE('',#11673,#11634,#6461,.T.);
#14528=EDGE_CURVE('',#11675,#11676,#9937,.T.);
#14529=EDGE_CURVE('',#11633,#11676,#6462,.T.);
#14530=EDGE_CURVE('',#11675,#11632,#6463,.T.);
#14531=EDGE_CURVE('',#11676,#11673,#6464,.T.);
#14532=EDGE_CURVE('',#11674,#11671,#6465,.T.);
#14533=EDGE_CURVE('',#11677,#11678,#9938,.T.);
#14534=EDGE_CURVE('',#11631,#11678,#6466,.T.);
#14535=EDGE_CURVE('',#11677,#11630,#6467,.T.);
#14536=EDGE_CURVE('',#11679,#11680,#9939,.T.);
#14537=EDGE_CURVE('',#11629,#11680,#6468,.T.);
#14538=EDGE_CURVE('',#11679,#11628,#6469,.T.);
#14539=EDGE_CURVE('',#11680,#11677,#9940,.T.);
#14540=EDGE_CURVE('',#11681,#11626,#6470,.T.);
#14541=EDGE_CURVE('',#11681,#11682,#6471,.T.);
#14542=EDGE_CURVE('',#11682,#11627,#6472,.T.);
#14543=EDGE_CURVE('',#11682,#11679,#6473,.T.);
#14544=EDGE_CURVE('',#11683,#11684,#9941,.T.);
#14545=EDGE_CURVE('',#11625,#11684,#6474,.T.);
#14546=EDGE_CURVE('',#11683,#11624,#6475,.T.);
#14547=EDGE_CURVE('',#11685,#11686,#9942,.T.);
#14548=EDGE_CURVE('',#11623,#11686,#6476,.T.);
#14549=EDGE_CURVE('',#11685,#11622,#6477,.T.);
#14550=EDGE_CURVE('',#11686,#11683,#9943,.T.);
#14551=EDGE_CURVE('',#11687,#11688,#9944,.T.);
#14552=EDGE_CURVE('',#11621,#11688,#6478,.T.);
#14553=EDGE_CURVE('',#11687,#11620,#6479,.T.);
#14554=EDGE_CURVE('',#11689,#11690,#9945,.T.);
#14555=EDGE_CURVE('',#11619,#11690,#6480,.T.);
#14556=EDGE_CURVE('',#11689,#11618,#6481,.T.);
#14557=EDGE_CURVE('',#11690,#11687,#6482,.T.);
#14558=EDGE_CURVE('',#11688,#11685,#6483,.T.);
#14559=EDGE_CURVE('',#11684,#11681,#6484,.T.);
#14560=EDGE_CURVE('',#11691,#11692,#9946,.T.);
#14561=EDGE_CURVE('',#11617,#11692,#6485,.T.);
#14562=EDGE_CURVE('',#11691,#11616,#6486,.T.);
#14563=EDGE_CURVE('',#11693,#11694,#9947,.T.);
#14564=EDGE_CURVE('',#11615,#11694,#6487,.T.);
#14565=EDGE_CURVE('',#11693,#11614,#6488,.T.);
#14566=EDGE_CURVE('',#11694,#11691,#9948,.T.);
#14567=EDGE_CURVE('',#11695,#11612,#6489,.T.);
#14568=EDGE_CURVE('',#11695,#11696,#9949,.T.);
#14569=EDGE_CURVE('',#11613,#11696,#6490,.T.);
#14570=EDGE_CURVE('',#11697,#11610,#6491,.T.);
#14571=EDGE_CURVE('',#11697,#11698,#9950,.T.);
#14572=EDGE_CURVE('',#11611,#11698,#6492,.T.);
#14573=EDGE_CURVE('',#11699,#11700,#6493,.T.);
#14574=EDGE_CURVE('',#11700,#11656,#6494,.T.);
#14575=EDGE_CURVE('',#11699,#11655,#6495,.T.);
#14576=EDGE_CURVE('',#11701,#11699,#6496,.T.);
#14577=EDGE_CURVE('',#11701,#11654,#6497,.T.);
#14578=EDGE_CURVE('',#11702,#11701,#6498,.T.);
#14579=EDGE_CURVE('',#11702,#11653,#6499,.T.);
#14580=EDGE_CURVE('',#11657,#11702,#6500,.T.);
#14581=EDGE_CURVE('',#11700,#11703,#6501,.T.);
#14582=EDGE_CURVE('',#11703,#11609,#6502,.T.);
#14583=EDGE_CURVE('',#11703,#11697,#6503,.T.);
#14584=EDGE_CURVE('',#11698,#11695,#6504,.T.);
#14585=EDGE_CURVE('',#11696,#11693,#6505,.T.);
#14586=EDGE_CURVE('',#11692,#11689,#6506,.T.);
#14587=EDGE_CURVE('',#11678,#11675,#6507,.T.);
#14588=EDGE_CURVE('',#11670,#11666,#6508,.T.);
#14589=EDGE_CURVE('',#11704,#11663,#6509,.T.);
#14590=EDGE_CURVE('',#11650,#11704,#6510,.T.);
#14591=EDGE_CURVE('',#11704,#11658,#6511,.T.);
#14592=EDGE_CURVE('',#11705,#11368,#6512,.T.);
#14593=EDGE_CURVE('',#11705,#11313,#6513,.T.);
#14594=EDGE_CURVE('',#11706,#11705,#9951,.T.);
#14595=EDGE_CURVE('',#11706,#11314,#6514,.T.);
#14596=EDGE_CURVE('',#11369,#11706,#6515,.T.);
#17884=ORIENTED_EDGE('',*,*,#13635,.F.);
#17885=ORIENTED_EDGE('',*,*,#13636,.T.);
#17886=ORIENTED_EDGE('',*,*,#13637,.T.);
#17887=ORIENTED_EDGE('',*,*,#13636,.F.);
#17888=ORIENTED_EDGE('',*,*,#13638,.F.);
#17889=ORIENTED_EDGE('',*,*,#13639,.T.);
#17890=ORIENTED_EDGE('',*,*,#13640,.T.);
#17891=ORIENTED_EDGE('',*,*,#13639,.F.);
#17892=ORIENTED_EDGE('',*,*,#13641,.F.);
#17893=ORIENTED_EDGE('',*,*,#13642,.T.);
#17894=ORIENTED_EDGE('',*,*,#13643,.T.);
#17895=ORIENTED_EDGE('',*,*,#13642,.F.);
#17896=ORIENTED_EDGE('',*,*,#13644,.T.);
#17897=ORIENTED_EDGE('',*,*,#13635,.T.);
#17898=ORIENTED_EDGE('',*,*,#13644,.F.);
#17899=ORIENTED_EDGE('',*,*,#13645,.T.);
#17900=ORIENTED_EDGE('',*,*,#13638,.T.);
#17901=ORIENTED_EDGE('',*,*,#13645,.F.);
#17902=ORIENTED_EDGE('',*,*,#13646,.F.);
#17903=ORIENTED_EDGE('',*,*,#13647,.T.);
#17904=ORIENTED_EDGE('',*,*,#13648,.T.);
#17905=ORIENTED_EDGE('',*,*,#13647,.F.);
#17906=ORIENTED_EDGE('',*,*,#13649,.F.);
#17907=ORIENTED_EDGE('',*,*,#13650,.T.);
#17908=ORIENTED_EDGE('',*,*,#13651,.T.);
#17909=ORIENTED_EDGE('',*,*,#13650,.F.);
#17910=ORIENTED_EDGE('',*,*,#13652,.F.);
#17911=ORIENTED_EDGE('',*,*,#13653,.T.);
#17912=ORIENTED_EDGE('',*,*,#13654,.T.);
#17913=ORIENTED_EDGE('',*,*,#13653,.F.);
#17914=ORIENTED_EDGE('',*,*,#13655,.F.);
#17915=ORIENTED_EDGE('',*,*,#13656,.T.);
#17916=ORIENTED_EDGE('',*,*,#13657,.T.);
#17917=ORIENTED_EDGE('',*,*,#13656,.F.);
#17918=ORIENTED_EDGE('',*,*,#13658,.F.);
#17919=ORIENTED_EDGE('',*,*,#13659,.T.);
#17920=ORIENTED_EDGE('',*,*,#13660,.T.);
#17921=ORIENTED_EDGE('',*,*,#13659,.F.);
#17922=ORIENTED_EDGE('',*,*,#13661,.F.);
#17923=ORIENTED_EDGE('',*,*,#13662,.T.);
#17924=ORIENTED_EDGE('',*,*,#13663,.T.);
#17925=ORIENTED_EDGE('',*,*,#13662,.F.);
#17926=ORIENTED_EDGE('',*,*,#13664,.F.);
#17927=ORIENTED_EDGE('',*,*,#13665,.T.);
#17928=ORIENTED_EDGE('',*,*,#13666,.T.);
#17929=ORIENTED_EDGE('',*,*,#13665,.F.);
#17930=ORIENTED_EDGE('',*,*,#13667,.F.);
#17931=ORIENTED_EDGE('',*,*,#13668,.T.);
#17932=ORIENTED_EDGE('',*,*,#13669,.T.);
#17933=ORIENTED_EDGE('',*,*,#13670,.T.);
#17934=ORIENTED_EDGE('',*,*,#13671,.T.);
#17935=ORIENTED_EDGE('',*,*,#13672,.F.);
#17936=ORIENTED_EDGE('',*,*,#13668,.F.);
#17937=ORIENTED_EDGE('',*,*,#13673,.T.);
#17938=ORIENTED_EDGE('',*,*,#13658,.T.);
#17939=ORIENTED_EDGE('',*,*,#13673,.F.);
#17940=ORIENTED_EDGE('',*,*,#13674,.T.);
#17941=ORIENTED_EDGE('',*,*,#13661,.T.);
#17942=ORIENTED_EDGE('',*,*,#13674,.F.);
#17943=ORIENTED_EDGE('',*,*,#13675,.F.);
#17944=ORIENTED_EDGE('',*,*,#13676,.T.);
#17945=ORIENTED_EDGE('',*,*,#13677,.T.);
#17946=ORIENTED_EDGE('',*,*,#13678,.T.);
#17947=ORIENTED_EDGE('',*,*,#13679,.F.);
#17948=ORIENTED_EDGE('',*,*,#13680,.T.);
#17949=ORIENTED_EDGE('',*,*,#13676,.F.);
#17950=ORIENTED_EDGE('',*,*,#13681,.F.);
#17951=ORIENTED_EDGE('',*,*,#13682,.F.);
#17952=ORIENTED_EDGE('',*,*,#13683,.F.);
#17953=ORIENTED_EDGE('',*,*,#13684,.T.);
#17954=ORIENTED_EDGE('',*,*,#13685,.F.);
#17955=ORIENTED_EDGE('',*,*,#13686,.F.);
#17956=ORIENTED_EDGE('',*,*,#13684,.F.);
#17957=ORIENTED_EDGE('',*,*,#13687,.F.);
#17958=ORIENTED_EDGE('',*,*,#13688,.F.);
#17959=ORIENTED_EDGE('',*,*,#13689,.F.);
#17960=ORIENTED_EDGE('',*,*,#13690,.T.);
#17961=ORIENTED_EDGE('',*,*,#13691,.T.);
#17962=ORIENTED_EDGE('',*,*,#13685,.T.);
#17963=ORIENTED_EDGE('',*,*,#13686,.T.);
#17964=ORIENTED_EDGE('',*,*,#13691,.F.);
#17965=ORIENTED_EDGE('',*,*,#13692,.F.);
#17966=ORIENTED_EDGE('',*,*,#13693,.T.);
#17967=ORIENTED_EDGE('',*,*,#13694,.T.);
#17968=ORIENTED_EDGE('',*,*,#13693,.F.);
#17969=ORIENTED_EDGE('',*,*,#13695,.F.);
#17970=ORIENTED_EDGE('',*,*,#13696,.F.);
#17971=ORIENTED_EDGE('',*,*,#13697,.T.);
#17972=ORIENTED_EDGE('',*,*,#13698,.T.);
#17973=ORIENTED_EDGE('',*,*,#13699,.F.);
#17974=ORIENTED_EDGE('',*,*,#13700,.T.);
#17975=ORIENTED_EDGE('',*,*,#13701,.F.);
#17976=ORIENTED_EDGE('',*,*,#13702,.F.);
#17977=ORIENTED_EDGE('',*,*,#13703,.F.);
#17978=ORIENTED_EDGE('',*,*,#13704,.T.);
#17979=ORIENTED_EDGE('',*,*,#13705,.F.);
#17980=ORIENTED_EDGE('',*,*,#13706,.F.);
#17981=ORIENTED_EDGE('',*,*,#13707,.F.);
#17982=ORIENTED_EDGE('',*,*,#13708,.T.);
#17983=ORIENTED_EDGE('',*,*,#13709,.F.);
#17984=ORIENTED_EDGE('',*,*,#13710,.F.);
#17985=ORIENTED_EDGE('',*,*,#13711,.F.);
#17986=ORIENTED_EDGE('',*,*,#13712,.T.);
#17987=ORIENTED_EDGE('',*,*,#13713,.T.);
#17988=ORIENTED_EDGE('',*,*,#13714,.T.);
#17989=ORIENTED_EDGE('',*,*,#13715,.F.);
#17990=ORIENTED_EDGE('',*,*,#13716,.T.);
#17991=ORIENTED_EDGE('',*,*,#13717,.T.);
#17992=ORIENTED_EDGE('',*,*,#13718,.T.);
#17993=ORIENTED_EDGE('',*,*,#13719,.F.);
#17994=ORIENTED_EDGE('',*,*,#13720,.T.);
#17995=ORIENTED_EDGE('',*,*,#13721,.T.);
#17996=ORIENTED_EDGE('',*,*,#13722,.T.);
#17997=ORIENTED_EDGE('',*,*,#13723,.F.);
#17998=ORIENTED_EDGE('',*,*,#13724,.T.);
#17999=ORIENTED_EDGE('',*,*,#13725,.T.);
#18000=ORIENTED_EDGE('',*,*,#13726,.T.);
#18001=ORIENTED_EDGE('',*,*,#13727,.F.);
#18002=ORIENTED_EDGE('',*,*,#13728,.T.);
#18003=ORIENTED_EDGE('',*,*,#13729,.T.);
#18004=ORIENTED_EDGE('',*,*,#13730,.T.);
#18005=ORIENTED_EDGE('',*,*,#13731,.F.);
#18006=ORIENTED_EDGE('',*,*,#13732,.T.);
#18007=ORIENTED_EDGE('',*,*,#13733,.T.);
#18008=ORIENTED_EDGE('',*,*,#13734,.T.);
#18009=ORIENTED_EDGE('',*,*,#13735,.F.);
#18010=ORIENTED_EDGE('',*,*,#13736,.T.);
#18011=ORIENTED_EDGE('',*,*,#13737,.T.);
#18012=ORIENTED_EDGE('',*,*,#13738,.T.);
#18013=ORIENTED_EDGE('',*,*,#13739,.F.);
#18014=ORIENTED_EDGE('',*,*,#13740,.T.);
#18015=ORIENTED_EDGE('',*,*,#13741,.T.);
#18016=ORIENTED_EDGE('',*,*,#13742,.T.);
#18017=ORIENTED_EDGE('',*,*,#13743,.F.);
#18018=ORIENTED_EDGE('',*,*,#13744,.F.);
#18019=ORIENTED_EDGE('',*,*,#13745,.T.);
#18020=ORIENTED_EDGE('',*,*,#13746,.T.);
#18021=ORIENTED_EDGE('',*,*,#13747,.F.);
#18022=ORIENTED_EDGE('',*,*,#13748,.F.);
#18023=ORIENTED_EDGE('',*,*,#13749,.T.);
#18024=ORIENTED_EDGE('',*,*,#13744,.T.);
#18025=ORIENTED_EDGE('',*,*,#13750,.F.);
#18026=ORIENTED_EDGE('',*,*,#13751,.F.);
#18027=ORIENTED_EDGE('',*,*,#13752,.T.);
#18028=ORIENTED_EDGE('',*,*,#13753,.T.);
#18029=ORIENTED_EDGE('',*,*,#13754,.F.);
#18030=ORIENTED_EDGE('',*,*,#13755,.T.);
#18031=ORIENTED_EDGE('',*,*,#13756,.T.);
#18032=ORIENTED_EDGE('',*,*,#13751,.T.);
#18033=ORIENTED_EDGE('',*,*,#13757,.F.);
#18034=ORIENTED_EDGE('',*,*,#13758,.T.);
#18035=ORIENTED_EDGE('',*,*,#13759,.T.);
#18036=ORIENTED_EDGE('',*,*,#13760,.T.);
#18037=ORIENTED_EDGE('',*,*,#13761,.F.);
#18038=ORIENTED_EDGE('',*,*,#13762,.T.);
#18039=ORIENTED_EDGE('',*,*,#13763,.T.);
#18040=ORIENTED_EDGE('',*,*,#13764,.T.);
#18041=ORIENTED_EDGE('',*,*,#13765,.F.);
#18042=ORIENTED_EDGE('',*,*,#13766,.T.);
#18043=ORIENTED_EDGE('',*,*,#13767,.T.);
#18044=ORIENTED_EDGE('',*,*,#13768,.T.);
#18045=ORIENTED_EDGE('',*,*,#13769,.F.);
#18046=ORIENTED_EDGE('',*,*,#13770,.F.);
#18047=ORIENTED_EDGE('',*,*,#13771,.T.);
#18048=ORIENTED_EDGE('',*,*,#13772,.T.);
#18049=ORIENTED_EDGE('',*,*,#13773,.F.);
#18050=ORIENTED_EDGE('',*,*,#13726,.F.);
#18051=ORIENTED_EDGE('',*,*,#13774,.T.);
#18052=ORIENTED_EDGE('',*,*,#13770,.T.);
#18053=ORIENTED_EDGE('',*,*,#13775,.F.);
#18054=ORIENTED_EDGE('',*,*,#13776,.T.);
#18055=ORIENTED_EDGE('',*,*,#13777,.T.);
#18056=ORIENTED_EDGE('',*,*,#13778,.T.);
#18057=ORIENTED_EDGE('',*,*,#13779,.F.);
#18058=ORIENTED_EDGE('',*,*,#13780,.T.);
#18059=ORIENTED_EDGE('',*,*,#13781,.T.);
#18060=ORIENTED_EDGE('',*,*,#13782,.T.);
#18061=ORIENTED_EDGE('',*,*,#13783,.F.);
#18062=ORIENTED_EDGE('',*,*,#13784,.T.);
#18063=ORIENTED_EDGE('',*,*,#13785,.T.);
#18064=ORIENTED_EDGE('',*,*,#13786,.T.);
#18065=ORIENTED_EDGE('',*,*,#13787,.F.);
#18066=ORIENTED_EDGE('',*,*,#13788,.T.);
#18067=ORIENTED_EDGE('',*,*,#13789,.T.);
#18068=ORIENTED_EDGE('',*,*,#13790,.T.);
#18069=ORIENTED_EDGE('',*,*,#13791,.F.);
#18070=ORIENTED_EDGE('',*,*,#13760,.F.);
#18071=ORIENTED_EDGE('',*,*,#13792,.F.);
#18072=ORIENTED_EDGE('',*,*,#13755,.F.);
#18073=ORIENTED_EDGE('',*,*,#13793,.F.);
#18074=ORIENTED_EDGE('',*,*,#13746,.F.);
#18075=ORIENTED_EDGE('',*,*,#13794,.F.);
#18076=ORIENTED_EDGE('',*,*,#13740,.F.);
#18077=ORIENTED_EDGE('',*,*,#13762,.F.);
#18078=ORIENTED_EDGE('',*,*,#13795,.F.);
#18079=ORIENTED_EDGE('',*,*,#13768,.F.);
#18080=ORIENTED_EDGE('',*,*,#13796,.F.);
#18081=ORIENTED_EDGE('',*,*,#13766,.F.);
#18082=ORIENTED_EDGE('',*,*,#13797,.F.);
#18083=ORIENTED_EDGE('',*,*,#13718,.F.);
#18084=ORIENTED_EDGE('',*,*,#13798,.F.);
#18085=ORIENTED_EDGE('',*,*,#13716,.F.);
#18086=ORIENTED_EDGE('',*,*,#13799,.F.);
#18087=ORIENTED_EDGE('',*,*,#13786,.F.);
#18088=ORIENTED_EDGE('',*,*,#13800,.F.);
#18089=ORIENTED_EDGE('',*,*,#13784,.F.);
#18090=ORIENTED_EDGE('',*,*,#13801,.F.);
#18091=ORIENTED_EDGE('',*,*,#13772,.F.);
#18092=ORIENTED_EDGE('',*,*,#13802,.F.);
#18093=ORIENTED_EDGE('',*,*,#13788,.F.);
#18094=ORIENTED_EDGE('',*,*,#13803,.F.);
#18095=ORIENTED_EDGE('',*,*,#13764,.F.);
#18096=ORIENTED_EDGE('',*,*,#13804,.F.);
#18097=ORIENTED_EDGE('',*,*,#13712,.F.);
#18098=ORIENTED_EDGE('',*,*,#13805,.F.);
#18099=ORIENTED_EDGE('',*,*,#13790,.F.);
#18100=ORIENTED_EDGE('',*,*,#13806,.F.);
#18101=ORIENTED_EDGE('',*,*,#13807,.F.);
#18102=ORIENTED_EDGE('',*,*,#13714,.F.);
#18103=ORIENTED_EDGE('',*,*,#13808,.F.);
#18104=ORIENTED_EDGE('',*,*,#13758,.F.);
#18105=ORIENTED_EDGE('',*,*,#13809,.F.);
#18106=ORIENTED_EDGE('',*,*,#13742,.F.);
#18107=ORIENTED_EDGE('',*,*,#13810,.F.);
#18108=ORIENTED_EDGE('',*,*,#13736,.F.);
#18109=ORIENTED_EDGE('',*,*,#13780,.F.);
#18110=ORIENTED_EDGE('',*,*,#13811,.F.);
#18111=ORIENTED_EDGE('',*,*,#13738,.F.);
#18112=ORIENTED_EDGE('',*,*,#13812,.F.);
#18113=ORIENTED_EDGE('',*,*,#13720,.F.);
#18114=ORIENTED_EDGE('',*,*,#13813,.F.);
#18115=ORIENTED_EDGE('',*,*,#13782,.F.);
#18116=ORIENTED_EDGE('',*,*,#13814,.F.);
#18117=ORIENTED_EDGE('',*,*,#13732,.F.);
#18118=ORIENTED_EDGE('',*,*,#13815,.F.);
#18119=ORIENTED_EDGE('',*,*,#13722,.F.);
#18120=ORIENTED_EDGE('',*,*,#13816,.F.);
#18121=ORIENTED_EDGE('',*,*,#13728,.F.);
#18122=ORIENTED_EDGE('',*,*,#13817,.F.);
#18123=ORIENTED_EDGE('',*,*,#13734,.F.);
#18124=ORIENTED_EDGE('',*,*,#13818,.F.);
#18125=ORIENTED_EDGE('',*,*,#13776,.F.);
#18126=ORIENTED_EDGE('',*,*,#13819,.F.);
#18127=ORIENTED_EDGE('',*,*,#13730,.F.);
#18128=ORIENTED_EDGE('',*,*,#13820,.F.);
#18129=ORIENTED_EDGE('',*,*,#13724,.F.);
#18130=ORIENTED_EDGE('',*,*,#13821,.F.);
#18131=ORIENTED_EDGE('',*,*,#13778,.F.);
#18132=ORIENTED_EDGE('',*,*,#13822,.F.);
#18133=ORIENTED_EDGE('',*,*,#13692,.T.);
#18134=ORIENTED_EDGE('',*,*,#13690,.F.);
#18135=ORIENTED_EDGE('',*,*,#13823,.T.);
#18136=ORIENTED_EDGE('',*,*,#13824,.F.);
#18137=ORIENTED_EDGE('',*,*,#13825,.F.);
#18138=ORIENTED_EDGE('',*,*,#13826,.F.);
#18139=ORIENTED_EDGE('',*,*,#13827,.T.);
#18140=ORIENTED_EDGE('',*,*,#13828,.T.);
#18141=ORIENTED_EDGE('',*,*,#13829,.T.);
#18142=ORIENTED_EDGE('',*,*,#13826,.T.);
#18143=ORIENTED_EDGE('',*,*,#13830,.T.);
#18144=ORIENTED_EDGE('',*,*,#13831,.T.);
#18145=ORIENTED_EDGE('',*,*,#13832,.T.);
#18146=ORIENTED_EDGE('',*,*,#13752,.F.);
#18147=ORIENTED_EDGE('',*,*,#13756,.F.);
#18148=ORIENTED_EDGE('',*,*,#13792,.T.);
#18149=ORIENTED_EDGE('',*,*,#13759,.F.);
#18150=ORIENTED_EDGE('',*,*,#13808,.T.);
#18151=ORIENTED_EDGE('',*,*,#13713,.F.);
#18152=ORIENTED_EDGE('',*,*,#13806,.T.);
#18153=ORIENTED_EDGE('',*,*,#13789,.F.);
#18154=ORIENTED_EDGE('',*,*,#13804,.T.);
#18155=ORIENTED_EDGE('',*,*,#13763,.F.);
#18156=ORIENTED_EDGE('',*,*,#13796,.T.);
#18157=ORIENTED_EDGE('',*,*,#13767,.F.);
#18158=ORIENTED_EDGE('',*,*,#13798,.T.);
#18159=ORIENTED_EDGE('',*,*,#13717,.F.);
#18160=ORIENTED_EDGE('',*,*,#13800,.T.);
#18161=ORIENTED_EDGE('',*,*,#13785,.F.);
#18162=ORIENTED_EDGE('',*,*,#13802,.T.);
#18163=ORIENTED_EDGE('',*,*,#13771,.F.);
#18164=ORIENTED_EDGE('',*,*,#13774,.F.);
#18165=ORIENTED_EDGE('',*,*,#13725,.F.);
#18166=ORIENTED_EDGE('',*,*,#13822,.T.);
#18167=ORIENTED_EDGE('',*,*,#13777,.F.);
#18168=ORIENTED_EDGE('',*,*,#13820,.T.);
#18169=ORIENTED_EDGE('',*,*,#13729,.F.);
#18170=ORIENTED_EDGE('',*,*,#13818,.T.);
#18171=ORIENTED_EDGE('',*,*,#13733,.F.);
#18172=ORIENTED_EDGE('',*,*,#13816,.T.);
#18173=ORIENTED_EDGE('',*,*,#13721,.F.);
#18174=ORIENTED_EDGE('',*,*,#13814,.T.);
#18175=ORIENTED_EDGE('',*,*,#13781,.F.);
#18176=ORIENTED_EDGE('',*,*,#13812,.T.);
#18177=ORIENTED_EDGE('',*,*,#13737,.F.);
#18178=ORIENTED_EDGE('',*,*,#13810,.T.);
#18179=ORIENTED_EDGE('',*,*,#13741,.F.);
#18180=ORIENTED_EDGE('',*,*,#13794,.T.);
#18181=ORIENTED_EDGE('',*,*,#13745,.F.);
#18182=ORIENTED_EDGE('',*,*,#13749,.F.);
#18183=ORIENTED_EDGE('',*,*,#13694,.F.);
#18184=ORIENTED_EDGE('',*,*,#13833,.T.);
#18185=ORIENTED_EDGE('',*,*,#13834,.F.);
#18186=ORIENTED_EDGE('',*,*,#13823,.F.);
#18187=ORIENTED_EDGE('',*,*,#13829,.F.);
#18188=ORIENTED_EDGE('',*,*,#13835,.T.);
#18189=ORIENTED_EDGE('',*,*,#13836,.F.);
#18190=ORIENTED_EDGE('',*,*,#13833,.F.);
#18191=ORIENTED_EDGE('',*,*,#13828,.F.);
#18192=ORIENTED_EDGE('',*,*,#13748,.T.);
#18193=ORIENTED_EDGE('',*,*,#13837,.F.);
#18194=ORIENTED_EDGE('',*,*,#13835,.F.);
#18195=ORIENTED_EDGE('',*,*,#13827,.F.);
#18196=ORIENTED_EDGE('',*,*,#13838,.T.);
#18197=ORIENTED_EDGE('',*,*,#13839,.F.);
#18198=ORIENTED_EDGE('',*,*,#13753,.F.);
#18199=ORIENTED_EDGE('',*,*,#13832,.F.);
#18200=ORIENTED_EDGE('',*,*,#13840,.T.);
#18201=ORIENTED_EDGE('',*,*,#13841,.F.);
#18202=ORIENTED_EDGE('',*,*,#13838,.F.);
#18203=ORIENTED_EDGE('',*,*,#13831,.F.);
#18204=ORIENTED_EDGE('',*,*,#13825,.T.);
#18205=ORIENTED_EDGE('',*,*,#13842,.F.);
#18206=ORIENTED_EDGE('',*,*,#13840,.F.);
#18207=ORIENTED_EDGE('',*,*,#13830,.F.);
#18208=ORIENTED_EDGE('',*,*,#13843,.T.);
#18209=ORIENTED_EDGE('',*,*,#13689,.T.);
#18210=ORIENTED_EDGE('',*,*,#13844,.F.);
#18211=ORIENTED_EDGE('',*,*,#13845,.F.);
#18212=ORIENTED_EDGE('',*,*,#13681,.T.);
#18213=ORIENTED_EDGE('',*,*,#13843,.F.);
#18214=ORIENTED_EDGE('',*,*,#13846,.F.);
#18215=ORIENTED_EDGE('',*,*,#13847,.T.);
#18216=ORIENTED_EDGE('',*,*,#13848,.T.);
#18217=ORIENTED_EDGE('',*,*,#13682,.T.);
#18218=ORIENTED_EDGE('',*,*,#13847,.F.);
#18219=ORIENTED_EDGE('',*,*,#13849,.F.);
#18220=ORIENTED_EDGE('',*,*,#13850,.T.);
#18221=ORIENTED_EDGE('',*,*,#13683,.T.);
#18222=ORIENTED_EDGE('',*,*,#13848,.F.);
#18223=ORIENTED_EDGE('',*,*,#13851,.F.);
#18224=ORIENTED_EDGE('',*,*,#13852,.T.);
#18225=ORIENTED_EDGE('',*,*,#13687,.T.);
#18226=ORIENTED_EDGE('',*,*,#13850,.F.);
#18227=ORIENTED_EDGE('',*,*,#13853,.F.);
#18228=ORIENTED_EDGE('',*,*,#13844,.T.);
#18229=ORIENTED_EDGE('',*,*,#13688,.T.);
#18230=ORIENTED_EDGE('',*,*,#13852,.F.);
#18231=ORIENTED_EDGE('',*,*,#13854,.F.);
#18232=ORIENTED_EDGE('',*,*,#13845,.T.);
#18233=ORIENTED_EDGE('',*,*,#13854,.T.);
#18234=ORIENTED_EDGE('',*,*,#13853,.T.);
#18235=ORIENTED_EDGE('',*,*,#13851,.T.);
#18236=ORIENTED_EDGE('',*,*,#13849,.T.);
#18237=ORIENTED_EDGE('',*,*,#13846,.T.);
#18238=ORIENTED_EDGE('',*,*,#13754,.T.);
#18239=ORIENTED_EDGE('',*,*,#13750,.T.);
#18240=ORIENTED_EDGE('',*,*,#13839,.T.);
#18241=ORIENTED_EDGE('',*,*,#13841,.T.);
#18242=ORIENTED_EDGE('',*,*,#13842,.T.);
#18243=ORIENTED_EDGE('',*,*,#13824,.T.);
#18244=ORIENTED_EDGE('',*,*,#13834,.T.);
#18245=ORIENTED_EDGE('',*,*,#13836,.T.);
#18246=ORIENTED_EDGE('',*,*,#13837,.T.);
#18247=ORIENTED_EDGE('',*,*,#13747,.T.);
#18248=ORIENTED_EDGE('',*,*,#13743,.T.);
#18249=ORIENTED_EDGE('',*,*,#13793,.T.);
#18250=ORIENTED_EDGE('',*,*,#13739,.T.);
#18251=ORIENTED_EDGE('',*,*,#13809,.T.);
#18252=ORIENTED_EDGE('',*,*,#13735,.T.);
#18253=ORIENTED_EDGE('',*,*,#13811,.T.);
#18254=ORIENTED_EDGE('',*,*,#13779,.T.);
#18255=ORIENTED_EDGE('',*,*,#13813,.T.);
#18256=ORIENTED_EDGE('',*,*,#13719,.T.);
#18257=ORIENTED_EDGE('',*,*,#13815,.T.);
#18258=ORIENTED_EDGE('',*,*,#13731,.T.);
#18259=ORIENTED_EDGE('',*,*,#13817,.T.);
#18260=ORIENTED_EDGE('',*,*,#13727,.T.);
#18261=ORIENTED_EDGE('',*,*,#13819,.T.);
#18262=ORIENTED_EDGE('',*,*,#13775,.T.);
#18263=ORIENTED_EDGE('',*,*,#13821,.T.);
#18264=ORIENTED_EDGE('',*,*,#13723,.T.);
#18265=ORIENTED_EDGE('',*,*,#13773,.T.);
#18266=ORIENTED_EDGE('',*,*,#13769,.T.);
#18267=ORIENTED_EDGE('',*,*,#13801,.T.);
#18268=ORIENTED_EDGE('',*,*,#13783,.T.);
#18269=ORIENTED_EDGE('',*,*,#13799,.T.);
#18270=ORIENTED_EDGE('',*,*,#13715,.T.);
#18271=ORIENTED_EDGE('',*,*,#13797,.T.);
#18272=ORIENTED_EDGE('',*,*,#13765,.T.);
#18273=ORIENTED_EDGE('',*,*,#13795,.T.);
#18274=ORIENTED_EDGE('',*,*,#13761,.T.);
#18275=ORIENTED_EDGE('',*,*,#13803,.T.);
#18276=ORIENTED_EDGE('',*,*,#13787,.T.);
#18277=ORIENTED_EDGE('',*,*,#13805,.T.);
#18278=ORIENTED_EDGE('',*,*,#13711,.T.);
#18279=ORIENTED_EDGE('',*,*,#13807,.T.);
#18280=ORIENTED_EDGE('',*,*,#13757,.T.);
#18281=ORIENTED_EDGE('',*,*,#13791,.T.);
#18282=ORIENTED_EDGE('',*,*,#13855,.F.);
#18283=ORIENTED_EDGE('',*,*,#13856,.F.);
#18284=ORIENTED_EDGE('',*,*,#13857,.F.);
#18285=ORIENTED_EDGE('',*,*,#13858,.F.);
#18286=ORIENTED_EDGE('',*,*,#13859,.F.);
#18287=ORIENTED_EDGE('',*,*,#13860,.F.);
#18288=ORIENTED_EDGE('',*,*,#13861,.F.);
#18289=ORIENTED_EDGE('',*,*,#13862,.F.);
#18290=ORIENTED_EDGE('',*,*,#13863,.F.);
#18291=ORIENTED_EDGE('',*,*,#13864,.F.);
#18292=ORIENTED_EDGE('',*,*,#13865,.F.);
#18293=ORIENTED_EDGE('',*,*,#13866,.F.);
#18294=ORIENTED_EDGE('',*,*,#13867,.F.);
#18295=ORIENTED_EDGE('',*,*,#13868,.F.);
#18296=ORIENTED_EDGE('',*,*,#13869,.F.);
#18297=ORIENTED_EDGE('',*,*,#13870,.F.);
#18298=ORIENTED_EDGE('',*,*,#13871,.F.);
#18299=ORIENTED_EDGE('',*,*,#13872,.F.);
#18300=ORIENTED_EDGE('',*,*,#13873,.F.);
#18301=ORIENTED_EDGE('',*,*,#13874,.F.);
#18302=ORIENTED_EDGE('',*,*,#13875,.F.);
#18303=ORIENTED_EDGE('',*,*,#13876,.F.);
#18304=ORIENTED_EDGE('',*,*,#13877,.F.);
#18305=ORIENTED_EDGE('',*,*,#13878,.F.);
#18306=ORIENTED_EDGE('',*,*,#13879,.F.);
#18307=ORIENTED_EDGE('',*,*,#13880,.F.);
#18308=ORIENTED_EDGE('',*,*,#13881,.F.);
#18309=ORIENTED_EDGE('',*,*,#13882,.F.);
#18310=ORIENTED_EDGE('',*,*,#13883,.F.);
#18311=ORIENTED_EDGE('',*,*,#13884,.F.);
#18312=ORIENTED_EDGE('',*,*,#13885,.F.);
#18313=ORIENTED_EDGE('',*,*,#13886,.F.);
#18314=ORIENTED_EDGE('',*,*,#13887,.F.);
#18315=ORIENTED_EDGE('',*,*,#13888,.F.);
#18316=ORIENTED_EDGE('',*,*,#13889,.F.);
#18317=ORIENTED_EDGE('',*,*,#13890,.F.);
#18318=ORIENTED_EDGE('',*,*,#13891,.F.);
#18319=ORIENTED_EDGE('',*,*,#13892,.F.);
#18320=ORIENTED_EDGE('',*,*,#13893,.F.);
#18321=ORIENTED_EDGE('',*,*,#13894,.F.);
#18322=ORIENTED_EDGE('',*,*,#13895,.F.);
#18323=ORIENTED_EDGE('',*,*,#13896,.F.);
#18324=ORIENTED_EDGE('',*,*,#13897,.F.);
#18325=ORIENTED_EDGE('',*,*,#13898,.F.);
#18326=ORIENTED_EDGE('',*,*,#13899,.F.);
#18327=ORIENTED_EDGE('',*,*,#13900,.F.);
#18328=ORIENTED_EDGE('',*,*,#13855,.T.);
#18329=ORIENTED_EDGE('',*,*,#13901,.T.);
#18330=ORIENTED_EDGE('',*,*,#13902,.F.);
#18331=ORIENTED_EDGE('',*,*,#13903,.F.);
#18332=ORIENTED_EDGE('',*,*,#13856,.T.);
#18333=ORIENTED_EDGE('',*,*,#13900,.T.);
#18334=ORIENTED_EDGE('',*,*,#13904,.F.);
#18335=ORIENTED_EDGE('',*,*,#13905,.F.);
#18336=ORIENTED_EDGE('',*,*,#13857,.T.);
#18337=ORIENTED_EDGE('',*,*,#13903,.T.);
#18338=ORIENTED_EDGE('',*,*,#13906,.F.);
#18339=ORIENTED_EDGE('',*,*,#13907,.F.);
#18340=ORIENTED_EDGE('',*,*,#13858,.T.);
#18341=ORIENTED_EDGE('',*,*,#13905,.T.);
#18342=ORIENTED_EDGE('',*,*,#13908,.F.);
#18343=ORIENTED_EDGE('',*,*,#13909,.F.);
#18344=ORIENTED_EDGE('',*,*,#13859,.T.);
#18345=ORIENTED_EDGE('',*,*,#13907,.T.);
#18346=ORIENTED_EDGE('',*,*,#13910,.F.);
#18347=ORIENTED_EDGE('',*,*,#13911,.F.);
#18348=ORIENTED_EDGE('',*,*,#13860,.T.);
#18349=ORIENTED_EDGE('',*,*,#13909,.T.);
#18350=ORIENTED_EDGE('',*,*,#13912,.F.);
#18351=ORIENTED_EDGE('',*,*,#13913,.F.);
#18352=ORIENTED_EDGE('',*,*,#13861,.T.);
#18353=ORIENTED_EDGE('',*,*,#13911,.T.);
#18354=ORIENTED_EDGE('',*,*,#13914,.F.);
#18355=ORIENTED_EDGE('',*,*,#13915,.F.);
#18356=ORIENTED_EDGE('',*,*,#13862,.T.);
#18357=ORIENTED_EDGE('',*,*,#13913,.T.);
#18358=ORIENTED_EDGE('',*,*,#13916,.F.);
#18359=ORIENTED_EDGE('',*,*,#13917,.F.);
#18360=ORIENTED_EDGE('',*,*,#13863,.T.);
#18361=ORIENTED_EDGE('',*,*,#13915,.T.);
#18362=ORIENTED_EDGE('',*,*,#13918,.F.);
#18363=ORIENTED_EDGE('',*,*,#13919,.F.);
#18364=ORIENTED_EDGE('',*,*,#13864,.T.);
#18365=ORIENTED_EDGE('',*,*,#13917,.T.);
#18366=ORIENTED_EDGE('',*,*,#13920,.F.);
#18367=ORIENTED_EDGE('',*,*,#13921,.F.);
#18368=ORIENTED_EDGE('',*,*,#13865,.T.);
#18369=ORIENTED_EDGE('',*,*,#13919,.T.);
#18370=ORIENTED_EDGE('',*,*,#13922,.F.);
#18371=ORIENTED_EDGE('',*,*,#13923,.F.);
#18372=ORIENTED_EDGE('',*,*,#13866,.T.);
#18373=ORIENTED_EDGE('',*,*,#13921,.T.);
#18374=ORIENTED_EDGE('',*,*,#13924,.F.);
#18375=ORIENTED_EDGE('',*,*,#13925,.F.);
#18376=ORIENTED_EDGE('',*,*,#13867,.T.);
#18377=ORIENTED_EDGE('',*,*,#13923,.T.);
#18378=ORIENTED_EDGE('',*,*,#13926,.F.);
#18379=ORIENTED_EDGE('',*,*,#13927,.F.);
#18380=ORIENTED_EDGE('',*,*,#13868,.T.);
#18381=ORIENTED_EDGE('',*,*,#13925,.T.);
#18382=ORIENTED_EDGE('',*,*,#13928,.F.);
#18383=ORIENTED_EDGE('',*,*,#13929,.F.);
#18384=ORIENTED_EDGE('',*,*,#13869,.T.);
#18385=ORIENTED_EDGE('',*,*,#13927,.T.);
#18386=ORIENTED_EDGE('',*,*,#13930,.F.);
#18387=ORIENTED_EDGE('',*,*,#13931,.F.);
#18388=ORIENTED_EDGE('',*,*,#13870,.T.);
#18389=ORIENTED_EDGE('',*,*,#13929,.T.);
#18390=ORIENTED_EDGE('',*,*,#13932,.F.);
#18391=ORIENTED_EDGE('',*,*,#13933,.F.);
#18392=ORIENTED_EDGE('',*,*,#13871,.T.);
#18393=ORIENTED_EDGE('',*,*,#13931,.T.);
#18394=ORIENTED_EDGE('',*,*,#13934,.F.);
#18395=ORIENTED_EDGE('',*,*,#13935,.F.);
#18396=ORIENTED_EDGE('',*,*,#13872,.T.);
#18397=ORIENTED_EDGE('',*,*,#13933,.T.);
#18398=ORIENTED_EDGE('',*,*,#13936,.F.);
#18399=ORIENTED_EDGE('',*,*,#13937,.F.);
#18400=ORIENTED_EDGE('',*,*,#13873,.T.);
#18401=ORIENTED_EDGE('',*,*,#13935,.T.);
#18402=ORIENTED_EDGE('',*,*,#13938,.F.);
#18403=ORIENTED_EDGE('',*,*,#13939,.F.);
#18404=ORIENTED_EDGE('',*,*,#13874,.T.);
#18405=ORIENTED_EDGE('',*,*,#13937,.T.);
#18406=ORIENTED_EDGE('',*,*,#13940,.F.);
#18407=ORIENTED_EDGE('',*,*,#13941,.F.);
#18408=ORIENTED_EDGE('',*,*,#13875,.T.);
#18409=ORIENTED_EDGE('',*,*,#13939,.T.);
#18410=ORIENTED_EDGE('',*,*,#13942,.F.);
#18411=ORIENTED_EDGE('',*,*,#13943,.F.);
#18412=ORIENTED_EDGE('',*,*,#13876,.T.);
#18413=ORIENTED_EDGE('',*,*,#13941,.T.);
#18414=ORIENTED_EDGE('',*,*,#13944,.F.);
#18415=ORIENTED_EDGE('',*,*,#13945,.F.);
#18416=ORIENTED_EDGE('',*,*,#13877,.T.);
#18417=ORIENTED_EDGE('',*,*,#13943,.T.);
#18418=ORIENTED_EDGE('',*,*,#13946,.F.);
#18419=ORIENTED_EDGE('',*,*,#13947,.F.);
#18420=ORIENTED_EDGE('',*,*,#13878,.T.);
#18421=ORIENTED_EDGE('',*,*,#13945,.T.);
#18422=ORIENTED_EDGE('',*,*,#13948,.F.);
#18423=ORIENTED_EDGE('',*,*,#13949,.F.);
#18424=ORIENTED_EDGE('',*,*,#13879,.T.);
#18425=ORIENTED_EDGE('',*,*,#13947,.T.);
#18426=ORIENTED_EDGE('',*,*,#13950,.F.);
#18427=ORIENTED_EDGE('',*,*,#13951,.F.);
#18428=ORIENTED_EDGE('',*,*,#13880,.T.);
#18429=ORIENTED_EDGE('',*,*,#13949,.T.);
#18430=ORIENTED_EDGE('',*,*,#13952,.F.);
#18431=ORIENTED_EDGE('',*,*,#13953,.F.);
#18432=ORIENTED_EDGE('',*,*,#13881,.T.);
#18433=ORIENTED_EDGE('',*,*,#13951,.T.);
#18434=ORIENTED_EDGE('',*,*,#13954,.F.);
#18435=ORIENTED_EDGE('',*,*,#13955,.F.);
#18436=ORIENTED_EDGE('',*,*,#13882,.T.);
#18437=ORIENTED_EDGE('',*,*,#13953,.T.);
#18438=ORIENTED_EDGE('',*,*,#13956,.F.);
#18439=ORIENTED_EDGE('',*,*,#13957,.F.);
#18440=ORIENTED_EDGE('',*,*,#13883,.T.);
#18441=ORIENTED_EDGE('',*,*,#13955,.T.);
#18442=ORIENTED_EDGE('',*,*,#13958,.F.);
#18443=ORIENTED_EDGE('',*,*,#13959,.F.);
#18444=ORIENTED_EDGE('',*,*,#13884,.T.);
#18445=ORIENTED_EDGE('',*,*,#13957,.T.);
#18446=ORIENTED_EDGE('',*,*,#13960,.F.);
#18447=ORIENTED_EDGE('',*,*,#13961,.F.);
#18448=ORIENTED_EDGE('',*,*,#13885,.T.);
#18449=ORIENTED_EDGE('',*,*,#13959,.T.);
#18450=ORIENTED_EDGE('',*,*,#13962,.F.);
#18451=ORIENTED_EDGE('',*,*,#13963,.F.);
#18452=ORIENTED_EDGE('',*,*,#13886,.T.);
#18453=ORIENTED_EDGE('',*,*,#13961,.T.);
#18454=ORIENTED_EDGE('',*,*,#13964,.F.);
#18455=ORIENTED_EDGE('',*,*,#13965,.F.);
#18456=ORIENTED_EDGE('',*,*,#13887,.T.);
#18457=ORIENTED_EDGE('',*,*,#13963,.T.);
#18458=ORIENTED_EDGE('',*,*,#13966,.F.);
#18459=ORIENTED_EDGE('',*,*,#13967,.F.);
#18460=ORIENTED_EDGE('',*,*,#13888,.T.);
#18461=ORIENTED_EDGE('',*,*,#13965,.T.);
#18462=ORIENTED_EDGE('',*,*,#13968,.F.);
#18463=ORIENTED_EDGE('',*,*,#13969,.F.);
#18464=ORIENTED_EDGE('',*,*,#13889,.T.);
#18465=ORIENTED_EDGE('',*,*,#13967,.T.);
#18466=ORIENTED_EDGE('',*,*,#13970,.F.);
#18467=ORIENTED_EDGE('',*,*,#13971,.F.);
#18468=ORIENTED_EDGE('',*,*,#13890,.T.);
#18469=ORIENTED_EDGE('',*,*,#13969,.T.);
#18470=ORIENTED_EDGE('',*,*,#13972,.F.);
#18471=ORIENTED_EDGE('',*,*,#13973,.F.);
#18472=ORIENTED_EDGE('',*,*,#13891,.T.);
#18473=ORIENTED_EDGE('',*,*,#13971,.T.);
#18474=ORIENTED_EDGE('',*,*,#13974,.F.);
#18475=ORIENTED_EDGE('',*,*,#13975,.F.);
#18476=ORIENTED_EDGE('',*,*,#13892,.T.);
#18477=ORIENTED_EDGE('',*,*,#13973,.T.);
#18478=ORIENTED_EDGE('',*,*,#13976,.F.);
#18479=ORIENTED_EDGE('',*,*,#13977,.F.);
#18480=ORIENTED_EDGE('',*,*,#13893,.T.);
#18481=ORIENTED_EDGE('',*,*,#13975,.T.);
#18482=ORIENTED_EDGE('',*,*,#13978,.F.);
#18483=ORIENTED_EDGE('',*,*,#13979,.F.);
#18484=ORIENTED_EDGE('',*,*,#13894,.T.);
#18485=ORIENTED_EDGE('',*,*,#13977,.T.);
#18486=ORIENTED_EDGE('',*,*,#13980,.F.);
#18487=ORIENTED_EDGE('',*,*,#13981,.F.);
#18488=ORIENTED_EDGE('',*,*,#13895,.T.);
#18489=ORIENTED_EDGE('',*,*,#13979,.T.);
#18490=ORIENTED_EDGE('',*,*,#13982,.F.);
#18491=ORIENTED_EDGE('',*,*,#13983,.F.);
#18492=ORIENTED_EDGE('',*,*,#13896,.T.);
#18493=ORIENTED_EDGE('',*,*,#13981,.T.);
#18494=ORIENTED_EDGE('',*,*,#13984,.F.);
#18495=ORIENTED_EDGE('',*,*,#13985,.F.);
#18496=ORIENTED_EDGE('',*,*,#13897,.T.);
#18497=ORIENTED_EDGE('',*,*,#13983,.T.);
#18498=ORIENTED_EDGE('',*,*,#13986,.F.);
#18499=ORIENTED_EDGE('',*,*,#13901,.F.);
#18500=ORIENTED_EDGE('',*,*,#13898,.T.);
#18501=ORIENTED_EDGE('',*,*,#13985,.T.);
#18502=ORIENTED_EDGE('',*,*,#13675,.T.);
#18503=ORIENTED_EDGE('',*,*,#13680,.F.);
#18504=ORIENTED_EDGE('',*,*,#13987,.T.);
#18505=ORIENTED_EDGE('',*,*,#13988,.T.);
#18506=ORIENTED_EDGE('',*,*,#13989,.T.);
#18507=ORIENTED_EDGE('',*,*,#13990,.F.);
#18508=ORIENTED_EDGE('',*,*,#13991,.F.);
#18509=ORIENTED_EDGE('',*,*,#13992,.F.);
#18510=ORIENTED_EDGE('',*,*,#13993,.F.);
#18511=ORIENTED_EDGE('',*,*,#13994,.F.);
#18512=ORIENTED_EDGE('',*,*,#13995,.F.);
#18513=ORIENTED_EDGE('',*,*,#13996,.F.);
#18514=ORIENTED_EDGE('',*,*,#13997,.F.);
#18515=ORIENTED_EDGE('',*,*,#13998,.T.);
#18516=ORIENTED_EDGE('',*,*,#13999,.T.);
#18517=ORIENTED_EDGE('',*,*,#14000,.T.);
#18518=ORIENTED_EDGE('',*,*,#14001,.T.);
#18519=ORIENTED_EDGE('',*,*,#14002,.T.);
#18520=ORIENTED_EDGE('',*,*,#14003,.T.);
#18521=ORIENTED_EDGE('',*,*,#14004,.T.);
#18522=ORIENTED_EDGE('',*,*,#14005,.T.);
#18523=ORIENTED_EDGE('',*,*,#14006,.T.);
#18524=ORIENTED_EDGE('',*,*,#14007,.T.);
#18525=ORIENTED_EDGE('',*,*,#14008,.T.);
#18526=ORIENTED_EDGE('',*,*,#14009,.T.);
#18527=ORIENTED_EDGE('',*,*,#14010,.T.);
#18528=ORIENTED_EDGE('',*,*,#14011,.T.);
#18529=ORIENTED_EDGE('',*,*,#14012,.T.);
#18530=ORIENTED_EDGE('',*,*,#14013,.T.);
#18531=ORIENTED_EDGE('',*,*,#14014,.T.);
#18532=ORIENTED_EDGE('',*,*,#14015,.T.);
#18533=ORIENTED_EDGE('',*,*,#14016,.T.);
#18534=ORIENTED_EDGE('',*,*,#14017,.T.);
#18535=ORIENTED_EDGE('',*,*,#14018,.T.);
#18536=ORIENTED_EDGE('',*,*,#14019,.T.);
#18537=ORIENTED_EDGE('',*,*,#14020,.T.);
#18538=ORIENTED_EDGE('',*,*,#14021,.T.);
#18539=ORIENTED_EDGE('',*,*,#14022,.T.);
#18540=ORIENTED_EDGE('',*,*,#14023,.T.);
#18541=ORIENTED_EDGE('',*,*,#14024,.T.);
#18542=ORIENTED_EDGE('',*,*,#14025,.T.);
#18543=ORIENTED_EDGE('',*,*,#14026,.T.);
#18544=ORIENTED_EDGE('',*,*,#14027,.T.);
#18545=ORIENTED_EDGE('',*,*,#14028,.T.);
#18546=ORIENTED_EDGE('',*,*,#14029,.T.);
#18547=ORIENTED_EDGE('',*,*,#14030,.T.);
#18548=ORIENTED_EDGE('',*,*,#14031,.T.);
#18549=ORIENTED_EDGE('',*,*,#14032,.T.);
#18550=ORIENTED_EDGE('',*,*,#14033,.T.);
#18551=ORIENTED_EDGE('',*,*,#14034,.T.);
#18552=ORIENTED_EDGE('',*,*,#14035,.F.);
#18553=ORIENTED_EDGE('',*,*,#14036,.F.);
#18554=ORIENTED_EDGE('',*,*,#14037,.F.);
#18555=ORIENTED_EDGE('',*,*,#14038,.T.);
#18556=ORIENTED_EDGE('',*,*,#13677,.F.);
#18557=ORIENTED_EDGE('',*,*,#13989,.F.);
#18558=ORIENTED_EDGE('',*,*,#14039,.T.);
#18559=ORIENTED_EDGE('',*,*,#14040,.T.);
#18560=ORIENTED_EDGE('',*,*,#14041,.F.);
#18561=ORIENTED_EDGE('',*,*,#13987,.F.);
#18562=ORIENTED_EDGE('',*,*,#13679,.T.);
#18563=ORIENTED_EDGE('',*,*,#14042,.T.);
#18564=ORIENTED_EDGE('',*,*,#14039,.F.);
#18565=ORIENTED_EDGE('',*,*,#13988,.F.);
#18566=ORIENTED_EDGE('',*,*,#14041,.T.);
#18567=ORIENTED_EDGE('',*,*,#13667,.T.);
#18568=ORIENTED_EDGE('',*,*,#13669,.F.);
#18569=ORIENTED_EDGE('',*,*,#14043,.T.);
#18570=ORIENTED_EDGE('',*,*,#14044,.T.);
#18571=ORIENTED_EDGE('',*,*,#14045,.T.);
#18572=ORIENTED_EDGE('',*,*,#14046,.T.);
#18573=ORIENTED_EDGE('',*,*,#14047,.T.);
#18574=ORIENTED_EDGE('',*,*,#14034,.F.);
#18575=ORIENTED_EDGE('',*,*,#14048,.F.);
#18576=ORIENTED_EDGE('',*,*,#14047,.F.);
#18577=ORIENTED_EDGE('',*,*,#14049,.T.);
#18578=ORIENTED_EDGE('',*,*,#14050,.T.);
#18579=ORIENTED_EDGE('',*,*,#14035,.T.);
#18580=ORIENTED_EDGE('',*,*,#14050,.F.);
#18581=ORIENTED_EDGE('',*,*,#14051,.T.);
#18582=ORIENTED_EDGE('',*,*,#14052,.T.);
#18583=ORIENTED_EDGE('',*,*,#14036,.T.);
#18584=ORIENTED_EDGE('',*,*,#14052,.F.);
#18585=ORIENTED_EDGE('',*,*,#14053,.T.);
#18586=ORIENTED_EDGE('',*,*,#14054,.T.);
#18587=ORIENTED_EDGE('',*,*,#14037,.T.);
#18588=ORIENTED_EDGE('',*,*,#14055,.F.);
#18589=ORIENTED_EDGE('',*,*,#14056,.T.);
#18590=ORIENTED_EDGE('',*,*,#13990,.T.);
#18591=ORIENTED_EDGE('',*,*,#14054,.F.);
#18592=ORIENTED_EDGE('',*,*,#14057,.T.);
#18593=ORIENTED_EDGE('',*,*,#14058,.T.);
#18594=ORIENTED_EDGE('',*,*,#13994,.T.);
#18595=ORIENTED_EDGE('',*,*,#14059,.F.);
#18596=ORIENTED_EDGE('',*,*,#14058,.F.);
#18597=ORIENTED_EDGE('',*,*,#14060,.T.);
#18598=ORIENTED_EDGE('',*,*,#14061,.T.);
#18599=ORIENTED_EDGE('',*,*,#13995,.T.);
#18600=ORIENTED_EDGE('',*,*,#14061,.F.);
#18601=ORIENTED_EDGE('',*,*,#14062,.T.);
#18602=ORIENTED_EDGE('',*,*,#14063,.T.);
#18603=ORIENTED_EDGE('',*,*,#13996,.T.);
#18604=ORIENTED_EDGE('',*,*,#14063,.F.);
#18605=ORIENTED_EDGE('',*,*,#14064,.T.);
#18606=ORIENTED_EDGE('',*,*,#14065,.T.);
#18607=ORIENTED_EDGE('',*,*,#13997,.T.);
#18608=ORIENTED_EDGE('',*,*,#14066,.T.);
#18609=ORIENTED_EDGE('',*,*,#14067,.T.);
#18610=ORIENTED_EDGE('',*,*,#13998,.F.);
#18611=ORIENTED_EDGE('',*,*,#14065,.F.);
#18612=ORIENTED_EDGE('',*,*,#14068,.T.);
#18613=ORIENTED_EDGE('',*,*,#14069,.T.);
#18614=ORIENTED_EDGE('',*,*,#13999,.F.);
#18615=ORIENTED_EDGE('',*,*,#14067,.F.);
#18616=ORIENTED_EDGE('',*,*,#14070,.T.);
#18617=ORIENTED_EDGE('',*,*,#14071,.F.);
#18618=ORIENTED_EDGE('',*,*,#14000,.F.);
#18619=ORIENTED_EDGE('',*,*,#14069,.F.);
#18620=ORIENTED_EDGE('',*,*,#14072,.T.);
#18621=ORIENTED_EDGE('',*,*,#14073,.T.);
#18622=ORIENTED_EDGE('',*,*,#14001,.F.);
#18623=ORIENTED_EDGE('',*,*,#14071,.T.);
#18624=ORIENTED_EDGE('',*,*,#14074,.T.);
#18625=ORIENTED_EDGE('',*,*,#14075,.F.);
#18626=ORIENTED_EDGE('',*,*,#14002,.F.);
#18627=ORIENTED_EDGE('',*,*,#14073,.F.);
#18628=ORIENTED_EDGE('',*,*,#14076,.T.);
#18629=ORIENTED_EDGE('',*,*,#14077,.T.);
#18630=ORIENTED_EDGE('',*,*,#14003,.F.);
#18631=ORIENTED_EDGE('',*,*,#14075,.T.);
#18632=ORIENTED_EDGE('',*,*,#14077,.F.);
#18633=ORIENTED_EDGE('',*,*,#14078,.T.);
#18634=ORIENTED_EDGE('',*,*,#14079,.F.);
#18635=ORIENTED_EDGE('',*,*,#14004,.F.);
#18636=ORIENTED_EDGE('',*,*,#14080,.T.);
#18637=ORIENTED_EDGE('',*,*,#14081,.T.);
#18638=ORIENTED_EDGE('',*,*,#14005,.F.);
#18639=ORIENTED_EDGE('',*,*,#14079,.T.);
#18640=ORIENTED_EDGE('',*,*,#14081,.F.);
#18641=ORIENTED_EDGE('',*,*,#14082,.T.);
#18642=ORIENTED_EDGE('',*,*,#14083,.F.);
#18643=ORIENTED_EDGE('',*,*,#14006,.F.);
#18644=ORIENTED_EDGE('',*,*,#14084,.T.);
#18645=ORIENTED_EDGE('',*,*,#14085,.T.);
#18646=ORIENTED_EDGE('',*,*,#14007,.F.);
#18647=ORIENTED_EDGE('',*,*,#14083,.T.);
#18648=ORIENTED_EDGE('',*,*,#14085,.F.);
#18649=ORIENTED_EDGE('',*,*,#14086,.T.);
#18650=ORIENTED_EDGE('',*,*,#14087,.F.);
#18651=ORIENTED_EDGE('',*,*,#14008,.F.);
#18652=ORIENTED_EDGE('',*,*,#14088,.T.);
#18653=ORIENTED_EDGE('',*,*,#14089,.T.);
#18654=ORIENTED_EDGE('',*,*,#14009,.F.);
#18655=ORIENTED_EDGE('',*,*,#14087,.T.);
#18656=ORIENTED_EDGE('',*,*,#14089,.F.);
#18657=ORIENTED_EDGE('',*,*,#14090,.T.);
#18658=ORIENTED_EDGE('',*,*,#14091,.F.);
#18659=ORIENTED_EDGE('',*,*,#14010,.F.);
#18660=ORIENTED_EDGE('',*,*,#14092,.T.);
#18661=ORIENTED_EDGE('',*,*,#14093,.T.);
#18662=ORIENTED_EDGE('',*,*,#14011,.F.);
#18663=ORIENTED_EDGE('',*,*,#14091,.T.);
#18664=ORIENTED_EDGE('',*,*,#14093,.F.);
#18665=ORIENTED_EDGE('',*,*,#14094,.T.);
#18666=ORIENTED_EDGE('',*,*,#14095,.F.);
#18667=ORIENTED_EDGE('',*,*,#14012,.F.);
#18668=ORIENTED_EDGE('',*,*,#14096,.T.);
#18669=ORIENTED_EDGE('',*,*,#14097,.T.);
#18670=ORIENTED_EDGE('',*,*,#14013,.F.);
#18671=ORIENTED_EDGE('',*,*,#14095,.T.);
#18672=ORIENTED_EDGE('',*,*,#14097,.F.);
#18673=ORIENTED_EDGE('',*,*,#14098,.T.);
#18674=ORIENTED_EDGE('',*,*,#14099,.F.);
#18675=ORIENTED_EDGE('',*,*,#14014,.F.);
#18676=ORIENTED_EDGE('',*,*,#14100,.T.);
#18677=ORIENTED_EDGE('',*,*,#14101,.T.);
#18678=ORIENTED_EDGE('',*,*,#14015,.F.);
#18679=ORIENTED_EDGE('',*,*,#14099,.T.);
#18680=ORIENTED_EDGE('',*,*,#14102,.T.);
#18681=ORIENTED_EDGE('',*,*,#14103,.T.);
#18682=ORIENTED_EDGE('',*,*,#14016,.F.);
#18683=ORIENTED_EDGE('',*,*,#14101,.F.);
#18684=ORIENTED_EDGE('',*,*,#14104,.T.);
#18685=ORIENTED_EDGE('',*,*,#14105,.T.);
#18686=ORIENTED_EDGE('',*,*,#14017,.F.);
#18687=ORIENTED_EDGE('',*,*,#14103,.F.);
#18688=ORIENTED_EDGE('',*,*,#14105,.F.);
#18689=ORIENTED_EDGE('',*,*,#14106,.T.);
#18690=ORIENTED_EDGE('',*,*,#14107,.F.);
#18691=ORIENTED_EDGE('',*,*,#14018,.F.);
#18692=ORIENTED_EDGE('',*,*,#14108,.T.);
#18693=ORIENTED_EDGE('',*,*,#14109,.T.);
#18694=ORIENTED_EDGE('',*,*,#14019,.F.);
#18695=ORIENTED_EDGE('',*,*,#14107,.T.);
#18696=ORIENTED_EDGE('',*,*,#14109,.F.);
#18697=ORIENTED_EDGE('',*,*,#14110,.T.);
#18698=ORIENTED_EDGE('',*,*,#14111,.F.);
#18699=ORIENTED_EDGE('',*,*,#14020,.F.);
#18700=ORIENTED_EDGE('',*,*,#14112,.T.);
#18701=ORIENTED_EDGE('',*,*,#14113,.T.);
#18702=ORIENTED_EDGE('',*,*,#14021,.F.);
#18703=ORIENTED_EDGE('',*,*,#14111,.T.);
#18704=ORIENTED_EDGE('',*,*,#14113,.F.);
#18705=ORIENTED_EDGE('',*,*,#14114,.T.);
#18706=ORIENTED_EDGE('',*,*,#14115,.F.);
#18707=ORIENTED_EDGE('',*,*,#14022,.F.);
#18708=ORIENTED_EDGE('',*,*,#14116,.T.);
#18709=ORIENTED_EDGE('',*,*,#14117,.T.);
#18710=ORIENTED_EDGE('',*,*,#14023,.F.);
#18711=ORIENTED_EDGE('',*,*,#14115,.T.);
#18712=ORIENTED_EDGE('',*,*,#14117,.F.);
#18713=ORIENTED_EDGE('',*,*,#14118,.T.);
#18714=ORIENTED_EDGE('',*,*,#14119,.F.);
#18715=ORIENTED_EDGE('',*,*,#14024,.F.);
#18716=ORIENTED_EDGE('',*,*,#14120,.T.);
#18717=ORIENTED_EDGE('',*,*,#14121,.T.);
#18718=ORIENTED_EDGE('',*,*,#14025,.F.);
#18719=ORIENTED_EDGE('',*,*,#14119,.T.);
#18720=ORIENTED_EDGE('',*,*,#14121,.F.);
#18721=ORIENTED_EDGE('',*,*,#14122,.T.);
#18722=ORIENTED_EDGE('',*,*,#14123,.F.);
#18723=ORIENTED_EDGE('',*,*,#14026,.F.);
#18724=ORIENTED_EDGE('',*,*,#14124,.T.);
#18725=ORIENTED_EDGE('',*,*,#14125,.T.);
#18726=ORIENTED_EDGE('',*,*,#14027,.F.);
#18727=ORIENTED_EDGE('',*,*,#14123,.T.);
#18728=ORIENTED_EDGE('',*,*,#14125,.F.);
#18729=ORIENTED_EDGE('',*,*,#14126,.T.);
#18730=ORIENTED_EDGE('',*,*,#14127,.F.);
#18731=ORIENTED_EDGE('',*,*,#14028,.F.);
#18732=ORIENTED_EDGE('',*,*,#14128,.T.);
#18733=ORIENTED_EDGE('',*,*,#14129,.T.);
#18734=ORIENTED_EDGE('',*,*,#14029,.F.);
#18735=ORIENTED_EDGE('',*,*,#14127,.T.);
#18736=ORIENTED_EDGE('',*,*,#14130,.T.);
#18737=ORIENTED_EDGE('',*,*,#14131,.F.);
#18738=ORIENTED_EDGE('',*,*,#14030,.F.);
#18739=ORIENTED_EDGE('',*,*,#14129,.F.);
#18740=ORIENTED_EDGE('',*,*,#14132,.T.);
#18741=ORIENTED_EDGE('',*,*,#14133,.T.);
#18742=ORIENTED_EDGE('',*,*,#14031,.F.);
#18743=ORIENTED_EDGE('',*,*,#14131,.T.);
#18744=ORIENTED_EDGE('',*,*,#14134,.T.);
#18745=ORIENTED_EDGE('',*,*,#14135,.F.);
#18746=ORIENTED_EDGE('',*,*,#14032,.F.);
#18747=ORIENTED_EDGE('',*,*,#14133,.F.);
#18748=ORIENTED_EDGE('',*,*,#14136,.T.);
#18749=ORIENTED_EDGE('',*,*,#14048,.T.);
#18750=ORIENTED_EDGE('',*,*,#14033,.F.);
#18751=ORIENTED_EDGE('',*,*,#14135,.T.);
#18752=ORIENTED_EDGE('',*,*,#13664,.T.);
#18753=ORIENTED_EDGE('',*,*,#14042,.F.);
#18754=ORIENTED_EDGE('',*,*,#14040,.F.);
#18755=ORIENTED_EDGE('',*,*,#13678,.F.);
#18756=ORIENTED_EDGE('',*,*,#14038,.F.);
#18757=ORIENTED_EDGE('',*,*,#14137,.T.);
#18758=ORIENTED_EDGE('',*,*,#14138,.T.);
#18759=ORIENTED_EDGE('',*,*,#14139,.T.);
#18760=ORIENTED_EDGE('',*,*,#14140,.T.);
#18761=ORIENTED_EDGE('',*,*,#14141,.T.);
#18762=ORIENTED_EDGE('',*,*,#14142,.T.);
#18763=ORIENTED_EDGE('',*,*,#14143,.T.);
#18764=ORIENTED_EDGE('',*,*,#14144,.F.);
#18765=ORIENTED_EDGE('',*,*,#14145,.T.);
#18766=ORIENTED_EDGE('',*,*,#13670,.F.);
#18767=ORIENTED_EDGE('',*,*,#14045,.F.);
#18768=ORIENTED_EDGE('',*,*,#14146,.T.);
#18769=ORIENTED_EDGE('',*,*,#14147,.T.);
#18770=ORIENTED_EDGE('',*,*,#14148,.F.);
#18771=ORIENTED_EDGE('',*,*,#14043,.F.);
#18772=ORIENTED_EDGE('',*,*,#13672,.T.);
#18773=ORIENTED_EDGE('',*,*,#14149,.T.);
#18774=ORIENTED_EDGE('',*,*,#14146,.F.);
#18775=ORIENTED_EDGE('',*,*,#14044,.F.);
#18776=ORIENTED_EDGE('',*,*,#14148,.T.);
#18777=ORIENTED_EDGE('',*,*,#14150,.F.);
#18778=ORIENTED_EDGE('',*,*,#14137,.F.);
#18779=ORIENTED_EDGE('',*,*,#14151,.F.);
#18780=ORIENTED_EDGE('',*,*,#14152,.F.);
#18781=ORIENTED_EDGE('',*,*,#14150,.T.);
#18782=ORIENTED_EDGE('',*,*,#14153,.F.);
#18783=ORIENTED_EDGE('',*,*,#14154,.T.);
#18784=ORIENTED_EDGE('',*,*,#14155,.T.);
#18785=ORIENTED_EDGE('',*,*,#14156,.F.);
#18786=ORIENTED_EDGE('',*,*,#14138,.F.);
#18787=ORIENTED_EDGE('',*,*,#14157,.T.);
#18788=ORIENTED_EDGE('',*,*,#14158,.T.);
#18789=ORIENTED_EDGE('',*,*,#14159,.F.);
#18790=ORIENTED_EDGE('',*,*,#14154,.F.);
#18791=ORIENTED_EDGE('',*,*,#14160,.T.);
#18792=ORIENTED_EDGE('',*,*,#14161,.T.);
#18793=ORIENTED_EDGE('',*,*,#14162,.T.);
#18794=ORIENTED_EDGE('',*,*,#14163,.F.);
#18795=ORIENTED_EDGE('',*,*,#14163,.T.);
#18796=ORIENTED_EDGE('',*,*,#14164,.F.);
#18797=ORIENTED_EDGE('',*,*,#14165,.T.);
#18798=ORIENTED_EDGE('',*,*,#14142,.F.);
#18799=ORIENTED_EDGE('',*,*,#14166,.F.);
#18800=ORIENTED_EDGE('',*,*,#14167,.T.);
#18801=ORIENTED_EDGE('',*,*,#14165,.F.);
#18802=ORIENTED_EDGE('',*,*,#14168,.F.);
#18803=ORIENTED_EDGE('',*,*,#14169,.T.);
#18804=ORIENTED_EDGE('',*,*,#14143,.F.);
#18805=ORIENTED_EDGE('',*,*,#14136,.F.);
#18806=ORIENTED_EDGE('',*,*,#14134,.F.);
#18807=ORIENTED_EDGE('',*,*,#14132,.F.);
#18808=ORIENTED_EDGE('',*,*,#14130,.F.);
#18809=ORIENTED_EDGE('',*,*,#14128,.F.);
#18810=ORIENTED_EDGE('',*,*,#14126,.F.);
#18811=ORIENTED_EDGE('',*,*,#14124,.F.);
#18812=ORIENTED_EDGE('',*,*,#14122,.F.);
#18813=ORIENTED_EDGE('',*,*,#14120,.F.);
#18814=ORIENTED_EDGE('',*,*,#14118,.F.);
#18815=ORIENTED_EDGE('',*,*,#14116,.F.);
#18816=ORIENTED_EDGE('',*,*,#14114,.F.);
#18817=ORIENTED_EDGE('',*,*,#14112,.F.);
#18818=ORIENTED_EDGE('',*,*,#14110,.F.);
#18819=ORIENTED_EDGE('',*,*,#14108,.F.);
#18820=ORIENTED_EDGE('',*,*,#14106,.F.);
#18821=ORIENTED_EDGE('',*,*,#14104,.F.);
#18822=ORIENTED_EDGE('',*,*,#14102,.F.);
#18823=ORIENTED_EDGE('',*,*,#14100,.F.);
#18824=ORIENTED_EDGE('',*,*,#14098,.F.);
#18825=ORIENTED_EDGE('',*,*,#14096,.F.);
#18826=ORIENTED_EDGE('',*,*,#14094,.F.);
#18827=ORIENTED_EDGE('',*,*,#14092,.F.);
#18828=ORIENTED_EDGE('',*,*,#14090,.F.);
#18829=ORIENTED_EDGE('',*,*,#14088,.F.);
#18830=ORIENTED_EDGE('',*,*,#14086,.F.);
#18831=ORIENTED_EDGE('',*,*,#14084,.F.);
#18832=ORIENTED_EDGE('',*,*,#14082,.F.);
#18833=ORIENTED_EDGE('',*,*,#14080,.F.);
#18834=ORIENTED_EDGE('',*,*,#14078,.F.);
#18835=ORIENTED_EDGE('',*,*,#14076,.F.);
#18836=ORIENTED_EDGE('',*,*,#14074,.F.);
#18837=ORIENTED_EDGE('',*,*,#14072,.F.);
#18838=ORIENTED_EDGE('',*,*,#14070,.F.);
#18839=ORIENTED_EDGE('',*,*,#14068,.F.);
#18840=ORIENTED_EDGE('',*,*,#14066,.F.);
#18841=ORIENTED_EDGE('',*,*,#14064,.F.);
#18842=ORIENTED_EDGE('',*,*,#14062,.F.);
#18843=ORIENTED_EDGE('',*,*,#14060,.F.);
#18844=ORIENTED_EDGE('',*,*,#14057,.F.);
#18845=ORIENTED_EDGE('',*,*,#14053,.F.);
#18846=ORIENTED_EDGE('',*,*,#14051,.F.);
#18847=ORIENTED_EDGE('',*,*,#14049,.F.);
#18848=ORIENTED_EDGE('',*,*,#14046,.F.);
#18849=ORIENTED_EDGE('',*,*,#14170,.T.);
#18850=ORIENTED_EDGE('',*,*,#14171,.T.);
#18851=ORIENTED_EDGE('',*,*,#14172,.T.);
#18852=ORIENTED_EDGE('',*,*,#14173,.T.);
#18853=ORIENTED_EDGE('',*,*,#14174,.T.);
#18854=ORIENTED_EDGE('',*,*,#14175,.T.);
#18855=ORIENTED_EDGE('',*,*,#14176,.T.);
#18856=ORIENTED_EDGE('',*,*,#14177,.T.);
#18857=ORIENTED_EDGE('',*,*,#14178,.T.);
#18858=ORIENTED_EDGE('',*,*,#14179,.T.);
#18859=ORIENTED_EDGE('',*,*,#14180,.T.);
#18860=ORIENTED_EDGE('',*,*,#14181,.T.);
#18861=ORIENTED_EDGE('',*,*,#14182,.T.);
#18862=ORIENTED_EDGE('',*,*,#14183,.T.);
#18863=ORIENTED_EDGE('',*,*,#14184,.T.);
#18864=ORIENTED_EDGE('',*,*,#14185,.T.);
#18865=ORIENTED_EDGE('',*,*,#14186,.T.);
#18866=ORIENTED_EDGE('',*,*,#14187,.T.);
#18867=ORIENTED_EDGE('',*,*,#14188,.T.);
#18868=ORIENTED_EDGE('',*,*,#14189,.T.);
#18869=ORIENTED_EDGE('',*,*,#14190,.T.);
#18870=ORIENTED_EDGE('',*,*,#14191,.T.);
#18871=ORIENTED_EDGE('',*,*,#14192,.T.);
#18872=ORIENTED_EDGE('',*,*,#14193,.T.);
#18873=ORIENTED_EDGE('',*,*,#14194,.T.);
#18874=ORIENTED_EDGE('',*,*,#14195,.T.);
#18875=ORIENTED_EDGE('',*,*,#14196,.T.);
#18876=ORIENTED_EDGE('',*,*,#14197,.T.);
#18877=ORIENTED_EDGE('',*,*,#14198,.T.);
#18878=ORIENTED_EDGE('',*,*,#14199,.T.);
#18879=ORIENTED_EDGE('',*,*,#14200,.T.);
#18880=ORIENTED_EDGE('',*,*,#14201,.T.);
#18881=ORIENTED_EDGE('',*,*,#14202,.T.);
#18882=ORIENTED_EDGE('',*,*,#14203,.T.);
#18883=ORIENTED_EDGE('',*,*,#14204,.T.);
#18884=ORIENTED_EDGE('',*,*,#14205,.T.);
#18885=ORIENTED_EDGE('',*,*,#14206,.T.);
#18886=ORIENTED_EDGE('',*,*,#14207,.T.);
#18887=ORIENTED_EDGE('',*,*,#14208,.T.);
#18888=ORIENTED_EDGE('',*,*,#14209,.T.);
#18889=ORIENTED_EDGE('',*,*,#14210,.T.);
#18890=ORIENTED_EDGE('',*,*,#14211,.T.);
#18891=ORIENTED_EDGE('',*,*,#14212,.T.);
#18892=ORIENTED_EDGE('',*,*,#14213,.T.);
#18893=ORIENTED_EDGE('',*,*,#14214,.F.);
#18894=ORIENTED_EDGE('',*,*,#14166,.T.);
#18895=ORIENTED_EDGE('',*,*,#14141,.F.);
#18896=ORIENTED_EDGE('',*,*,#14215,.F.);
#18897=ORIENTED_EDGE('',*,*,#14139,.F.);
#18898=ORIENTED_EDGE('',*,*,#14156,.T.);
#18899=ORIENTED_EDGE('',*,*,#14216,.F.);
#18900=ORIENTED_EDGE('',*,*,#14217,.T.);
#18901=ORIENTED_EDGE('',*,*,#14218,.T.);
#18902=ORIENTED_EDGE('',*,*,#14219,.F.);
#18903=ORIENTED_EDGE('',*,*,#14151,.T.);
#18904=ORIENTED_EDGE('',*,*,#14140,.F.);
#18905=ORIENTED_EDGE('',*,*,#14217,.F.);
#18906=ORIENTED_EDGE('',*,*,#14220,.T.);
#18907=ORIENTED_EDGE('',*,*,#14221,.T.);
#18908=ORIENTED_EDGE('',*,*,#14222,.T.);
#18909=ORIENTED_EDGE('',*,*,#14223,.T.);
#18910=ORIENTED_EDGE('',*,*,#14218,.F.);
#18911=ORIENTED_EDGE('',*,*,#14224,.T.);
#18912=ORIENTED_EDGE('',*,*,#14215,.T.);
#18913=ORIENTED_EDGE('',*,*,#14144,.T.);
#18914=ORIENTED_EDGE('',*,*,#14169,.F.);
#18915=ORIENTED_EDGE('',*,*,#14225,.T.);
#18916=ORIENTED_EDGE('',*,*,#14226,.T.);
#18917=ORIENTED_EDGE('',*,*,#14227,.T.);
#18918=ORIENTED_EDGE('',*,*,#14228,.T.);
#18919=ORIENTED_EDGE('',*,*,#14229,.F.);
#18920=ORIENTED_EDGE('',*,*,#14226,.F.);
#18921=ORIENTED_EDGE('',*,*,#13641,.T.);
#18922=ORIENTED_EDGE('',*,*,#14149,.F.);
#18923=ORIENTED_EDGE('',*,*,#14147,.F.);
#18924=ORIENTED_EDGE('',*,*,#13671,.F.);
#18925=ORIENTED_EDGE('',*,*,#14145,.F.);
#18926=ORIENTED_EDGE('',*,*,#14230,.F.);
#18927=ORIENTED_EDGE('',*,*,#13706,.T.);
#18928=ORIENTED_EDGE('',*,*,#14231,.F.);
#18929=ORIENTED_EDGE('',*,*,#14157,.F.);
#18930=ORIENTED_EDGE('',*,*,#14153,.T.);
#18931=ORIENTED_EDGE('',*,*,#14152,.T.);
#18932=ORIENTED_EDGE('',*,*,#14219,.T.);
#18933=ORIENTED_EDGE('',*,*,#14223,.F.);
#18934=ORIENTED_EDGE('',*,*,#14232,.T.);
#18935=ORIENTED_EDGE('',*,*,#14160,.F.);
#18936=ORIENTED_EDGE('',*,*,#14167,.F.);
#18937=ORIENTED_EDGE('',*,*,#14233,.F.);
#18938=ORIENTED_EDGE('',*,*,#14234,.T.);
#18939=ORIENTED_EDGE('',*,*,#14235,.F.);
#18940=ORIENTED_EDGE('',*,*,#13649,.T.);
#18941=ORIENTED_EDGE('',*,*,#14236,.T.);
#18942=ORIENTED_EDGE('',*,*,#14237,.T.);
#18943=ORIENTED_EDGE('',*,*,#14235,.T.);
#18944=ORIENTED_EDGE('',*,*,#14238,.T.);
#18945=ORIENTED_EDGE('',*,*,#14239,.F.);
#18946=ORIENTED_EDGE('',*,*,#13710,.T.);
#18947=ORIENTED_EDGE('',*,*,#14240,.F.);
#18948=ORIENTED_EDGE('',*,*,#14241,.F.);
#18949=ORIENTED_EDGE('',*,*,#14242,.F.);
#18950=ORIENTED_EDGE('',*,*,#14243,.T.);
#18951=ORIENTED_EDGE('',*,*,#14241,.T.);
#18952=ORIENTED_EDGE('',*,*,#14244,.T.);
#18953=ORIENTED_EDGE('',*,*,#14245,.T.);
#18954=ORIENTED_EDGE('',*,*,#14246,.F.);
#18955=ORIENTED_EDGE('',*,*,#14155,.F.);
#18956=ORIENTED_EDGE('',*,*,#14159,.T.);
#18957=ORIENTED_EDGE('',*,*,#14247,.T.);
#18958=ORIENTED_EDGE('',*,*,#14242,.T.);
#18959=ORIENTED_EDGE('',*,*,#13655,.T.);
#18960=ORIENTED_EDGE('',*,*,#14248,.F.);
#18961=ORIENTED_EDGE('',*,*,#14236,.F.);
#18962=ORIENTED_EDGE('',*,*,#14249,.F.);
#18963=ORIENTED_EDGE('',*,*,#14250,.F.);
#18964=ORIENTED_EDGE('',*,*,#14251,.F.);
#18965=ORIENTED_EDGE('',*,*,#14227,.F.);
#18966=ORIENTED_EDGE('',*,*,#14225,.F.);
#18967=ORIENTED_EDGE('',*,*,#14168,.T.);
#18968=ORIENTED_EDGE('',*,*,#14164,.T.);
#18969=ORIENTED_EDGE('',*,*,#14162,.F.);
#18970=ORIENTED_EDGE('',*,*,#14252,.F.);
#18971=ORIENTED_EDGE('',*,*,#13700,.F.);
#18972=ORIENTED_EDGE('',*,*,#14253,.T.);
#18973=ORIENTED_EDGE('',*,*,#14254,.F.);
#18974=ORIENTED_EDGE('',*,*,#14170,.F.);
#18975=ORIENTED_EDGE('',*,*,#14255,.T.);
#18976=ORIENTED_EDGE('',*,*,#14256,.T.);
#18977=ORIENTED_EDGE('',*,*,#14257,.F.);
#18978=ORIENTED_EDGE('',*,*,#14171,.F.);
#18979=ORIENTED_EDGE('',*,*,#14254,.T.);
#18980=ORIENTED_EDGE('',*,*,#14258,.T.);
#18981=ORIENTED_EDGE('',*,*,#14259,.F.);
#18982=ORIENTED_EDGE('',*,*,#14172,.F.);
#18983=ORIENTED_EDGE('',*,*,#14257,.T.);
#18984=ORIENTED_EDGE('',*,*,#14260,.T.);
#18985=ORIENTED_EDGE('',*,*,#14261,.F.);
#18986=ORIENTED_EDGE('',*,*,#14173,.F.);
#18987=ORIENTED_EDGE('',*,*,#14259,.T.);
#18988=ORIENTED_EDGE('',*,*,#14262,.T.);
#18989=ORIENTED_EDGE('',*,*,#14263,.F.);
#18990=ORIENTED_EDGE('',*,*,#14174,.F.);
#18991=ORIENTED_EDGE('',*,*,#14261,.T.);
#18992=ORIENTED_EDGE('',*,*,#14264,.T.);
#18993=ORIENTED_EDGE('',*,*,#14265,.F.);
#18994=ORIENTED_EDGE('',*,*,#14175,.F.);
#18995=ORIENTED_EDGE('',*,*,#14263,.T.);
#18996=ORIENTED_EDGE('',*,*,#14266,.T.);
#18997=ORIENTED_EDGE('',*,*,#14267,.F.);
#18998=ORIENTED_EDGE('',*,*,#14176,.F.);
#18999=ORIENTED_EDGE('',*,*,#14265,.T.);
#19000=ORIENTED_EDGE('',*,*,#14268,.T.);
#19001=ORIENTED_EDGE('',*,*,#14269,.F.);
#19002=ORIENTED_EDGE('',*,*,#14177,.F.);
#19003=ORIENTED_EDGE('',*,*,#14267,.T.);
#19004=ORIENTED_EDGE('',*,*,#14270,.T.);
#19005=ORIENTED_EDGE('',*,*,#14271,.F.);
#19006=ORIENTED_EDGE('',*,*,#14178,.F.);
#19007=ORIENTED_EDGE('',*,*,#14269,.T.);
#19008=ORIENTED_EDGE('',*,*,#14272,.T.);
#19009=ORIENTED_EDGE('',*,*,#14273,.F.);
#19010=ORIENTED_EDGE('',*,*,#14179,.F.);
#19011=ORIENTED_EDGE('',*,*,#14271,.T.);
#19012=ORIENTED_EDGE('',*,*,#14274,.T.);
#19013=ORIENTED_EDGE('',*,*,#14275,.F.);
#19014=ORIENTED_EDGE('',*,*,#14180,.F.);
#19015=ORIENTED_EDGE('',*,*,#14273,.T.);
#19016=ORIENTED_EDGE('',*,*,#14276,.T.);
#19017=ORIENTED_EDGE('',*,*,#14277,.F.);
#19018=ORIENTED_EDGE('',*,*,#14181,.F.);
#19019=ORIENTED_EDGE('',*,*,#14275,.T.);
#19020=ORIENTED_EDGE('',*,*,#14278,.T.);
#19021=ORIENTED_EDGE('',*,*,#14279,.F.);
#19022=ORIENTED_EDGE('',*,*,#14182,.F.);
#19023=ORIENTED_EDGE('',*,*,#14277,.T.);
#19024=ORIENTED_EDGE('',*,*,#14280,.T.);
#19025=ORIENTED_EDGE('',*,*,#14281,.F.);
#19026=ORIENTED_EDGE('',*,*,#14183,.F.);
#19027=ORIENTED_EDGE('',*,*,#14279,.T.);
#19028=ORIENTED_EDGE('',*,*,#14282,.T.);
#19029=ORIENTED_EDGE('',*,*,#14283,.F.);
#19030=ORIENTED_EDGE('',*,*,#14184,.F.);
#19031=ORIENTED_EDGE('',*,*,#14281,.T.);
#19032=ORIENTED_EDGE('',*,*,#14284,.T.);
#19033=ORIENTED_EDGE('',*,*,#14285,.F.);
#19034=ORIENTED_EDGE('',*,*,#14185,.F.);
#19035=ORIENTED_EDGE('',*,*,#14283,.T.);
#19036=ORIENTED_EDGE('',*,*,#14286,.T.);
#19037=ORIENTED_EDGE('',*,*,#14287,.F.);
#19038=ORIENTED_EDGE('',*,*,#14186,.F.);
#19039=ORIENTED_EDGE('',*,*,#14285,.T.);
#19040=ORIENTED_EDGE('',*,*,#14288,.T.);
#19041=ORIENTED_EDGE('',*,*,#14289,.F.);
#19042=ORIENTED_EDGE('',*,*,#14187,.F.);
#19043=ORIENTED_EDGE('',*,*,#14287,.T.);
#19044=ORIENTED_EDGE('',*,*,#14290,.T.);
#19045=ORIENTED_EDGE('',*,*,#14291,.F.);
#19046=ORIENTED_EDGE('',*,*,#14188,.F.);
#19047=ORIENTED_EDGE('',*,*,#14289,.T.);
#19048=ORIENTED_EDGE('',*,*,#14292,.T.);
#19049=ORIENTED_EDGE('',*,*,#14293,.F.);
#19050=ORIENTED_EDGE('',*,*,#14189,.F.);
#19051=ORIENTED_EDGE('',*,*,#14291,.T.);
#19052=ORIENTED_EDGE('',*,*,#14294,.T.);
#19053=ORIENTED_EDGE('',*,*,#14295,.F.);
#19054=ORIENTED_EDGE('',*,*,#14190,.F.);
#19055=ORIENTED_EDGE('',*,*,#14293,.T.);
#19056=ORIENTED_EDGE('',*,*,#14296,.T.);
#19057=ORIENTED_EDGE('',*,*,#14297,.F.);
#19058=ORIENTED_EDGE('',*,*,#14191,.F.);
#19059=ORIENTED_EDGE('',*,*,#14295,.T.);
#19060=ORIENTED_EDGE('',*,*,#14298,.T.);
#19061=ORIENTED_EDGE('',*,*,#14299,.F.);
#19062=ORIENTED_EDGE('',*,*,#14192,.F.);
#19063=ORIENTED_EDGE('',*,*,#14297,.T.);
#19064=ORIENTED_EDGE('',*,*,#14300,.T.);
#19065=ORIENTED_EDGE('',*,*,#14301,.F.);
#19066=ORIENTED_EDGE('',*,*,#14193,.F.);
#19067=ORIENTED_EDGE('',*,*,#14299,.T.);
#19068=ORIENTED_EDGE('',*,*,#14302,.T.);
#19069=ORIENTED_EDGE('',*,*,#14303,.F.);
#19070=ORIENTED_EDGE('',*,*,#14194,.F.);
#19071=ORIENTED_EDGE('',*,*,#14301,.T.);
#19072=ORIENTED_EDGE('',*,*,#14304,.T.);
#19073=ORIENTED_EDGE('',*,*,#14305,.F.);
#19074=ORIENTED_EDGE('',*,*,#14195,.F.);
#19075=ORIENTED_EDGE('',*,*,#14303,.T.);
#19076=ORIENTED_EDGE('',*,*,#14306,.T.);
#19077=ORIENTED_EDGE('',*,*,#14307,.F.);
#19078=ORIENTED_EDGE('',*,*,#14196,.F.);
#19079=ORIENTED_EDGE('',*,*,#14305,.T.);
#19080=ORIENTED_EDGE('',*,*,#14308,.T.);
#19081=ORIENTED_EDGE('',*,*,#14309,.F.);
#19082=ORIENTED_EDGE('',*,*,#14197,.F.);
#19083=ORIENTED_EDGE('',*,*,#14307,.T.);
#19084=ORIENTED_EDGE('',*,*,#14310,.T.);
#19085=ORIENTED_EDGE('',*,*,#14311,.F.);
#19086=ORIENTED_EDGE('',*,*,#14198,.F.);
#19087=ORIENTED_EDGE('',*,*,#14309,.T.);
#19088=ORIENTED_EDGE('',*,*,#14312,.T.);
#19089=ORIENTED_EDGE('',*,*,#14313,.F.);
#19090=ORIENTED_EDGE('',*,*,#14199,.F.);
#19091=ORIENTED_EDGE('',*,*,#14311,.T.);
#19092=ORIENTED_EDGE('',*,*,#14314,.T.);
#19093=ORIENTED_EDGE('',*,*,#14315,.F.);
#19094=ORIENTED_EDGE('',*,*,#14200,.F.);
#19095=ORIENTED_EDGE('',*,*,#14313,.T.);
#19096=ORIENTED_EDGE('',*,*,#14316,.T.);
#19097=ORIENTED_EDGE('',*,*,#14317,.F.);
#19098=ORIENTED_EDGE('',*,*,#14201,.F.);
#19099=ORIENTED_EDGE('',*,*,#14315,.T.);
#19100=ORIENTED_EDGE('',*,*,#14318,.T.);
#19101=ORIENTED_EDGE('',*,*,#14319,.F.);
#19102=ORIENTED_EDGE('',*,*,#14202,.F.);
#19103=ORIENTED_EDGE('',*,*,#14317,.T.);
#19104=ORIENTED_EDGE('',*,*,#14320,.T.);
#19105=ORIENTED_EDGE('',*,*,#14321,.F.);
#19106=ORIENTED_EDGE('',*,*,#14203,.F.);
#19107=ORIENTED_EDGE('',*,*,#14319,.T.);
#19108=ORIENTED_EDGE('',*,*,#14322,.T.);
#19109=ORIENTED_EDGE('',*,*,#14323,.F.);
#19110=ORIENTED_EDGE('',*,*,#14204,.F.);
#19111=ORIENTED_EDGE('',*,*,#14321,.T.);
#19112=ORIENTED_EDGE('',*,*,#14324,.T.);
#19113=ORIENTED_EDGE('',*,*,#14325,.F.);
#19114=ORIENTED_EDGE('',*,*,#14205,.F.);
#19115=ORIENTED_EDGE('',*,*,#14323,.T.);
#19116=ORIENTED_EDGE('',*,*,#14326,.T.);
#19117=ORIENTED_EDGE('',*,*,#14327,.F.);
#19118=ORIENTED_EDGE('',*,*,#14206,.F.);
#19119=ORIENTED_EDGE('',*,*,#14325,.T.);
#19120=ORIENTED_EDGE('',*,*,#14328,.T.);
#19121=ORIENTED_EDGE('',*,*,#14329,.F.);
#19122=ORIENTED_EDGE('',*,*,#14207,.F.);
#19123=ORIENTED_EDGE('',*,*,#14327,.T.);
#19124=ORIENTED_EDGE('',*,*,#14330,.T.);
#19125=ORIENTED_EDGE('',*,*,#14331,.F.);
#19126=ORIENTED_EDGE('',*,*,#14208,.F.);
#19127=ORIENTED_EDGE('',*,*,#14329,.T.);
#19128=ORIENTED_EDGE('',*,*,#14332,.T.);
#19129=ORIENTED_EDGE('',*,*,#14333,.F.);
#19130=ORIENTED_EDGE('',*,*,#14209,.F.);
#19131=ORIENTED_EDGE('',*,*,#14331,.T.);
#19132=ORIENTED_EDGE('',*,*,#14334,.T.);
#19133=ORIENTED_EDGE('',*,*,#14335,.F.);
#19134=ORIENTED_EDGE('',*,*,#14210,.F.);
#19135=ORIENTED_EDGE('',*,*,#14333,.T.);
#19136=ORIENTED_EDGE('',*,*,#14336,.T.);
#19137=ORIENTED_EDGE('',*,*,#14337,.F.);
#19138=ORIENTED_EDGE('',*,*,#14211,.F.);
#19139=ORIENTED_EDGE('',*,*,#14335,.T.);
#19140=ORIENTED_EDGE('',*,*,#14338,.T.);
#19141=ORIENTED_EDGE('',*,*,#14339,.F.);
#19142=ORIENTED_EDGE('',*,*,#14212,.F.);
#19143=ORIENTED_EDGE('',*,*,#14337,.T.);
#19144=ORIENTED_EDGE('',*,*,#14340,.T.);
#19145=ORIENTED_EDGE('',*,*,#14255,.F.);
#19146=ORIENTED_EDGE('',*,*,#14213,.F.);
#19147=ORIENTED_EDGE('',*,*,#14339,.T.);
#19148=ORIENTED_EDGE('',*,*,#14341,.T.);
#19149=ORIENTED_EDGE('',*,*,#14342,.T.);
#19150=ORIENTED_EDGE('',*,*,#14343,.T.);
#19151=ORIENTED_EDGE('',*,*,#14344,.T.);
#19152=ORIENTED_EDGE('',*,*,#13666,.F.);
#19153=ORIENTED_EDGE('',*,*,#14345,.F.);
#19154=ORIENTED_EDGE('',*,*,#14346,.T.);
#19155=ORIENTED_EDGE('',*,*,#14347,.F.);
#19156=ORIENTED_EDGE('',*,*,#14342,.F.);
#19157=ORIENTED_EDGE('',*,*,#14348,.F.);
#19158=ORIENTED_EDGE('',*,*,#14349,.F.);
#19159=ORIENTED_EDGE('',*,*,#14350,.F.);
#19160=ORIENTED_EDGE('',*,*,#14346,.F.);
#19161=ORIENTED_EDGE('',*,*,#14351,.F.);
#19162=ORIENTED_EDGE('',*,*,#14352,.F.);
#19163=ORIENTED_EDGE('',*,*,#14353,.F.);
#19164=ORIENTED_EDGE('',*,*,#14349,.T.);
#19165=ORIENTED_EDGE('',*,*,#14354,.F.);
#19166=ORIENTED_EDGE('',*,*,#14355,.F.);
#19167=ORIENTED_EDGE('',*,*,#14356,.F.);
#19168=ORIENTED_EDGE('',*,*,#14352,.T.);
#19169=ORIENTED_EDGE('',*,*,#13663,.F.);
#19170=ORIENTED_EDGE('',*,*,#14357,.F.);
#19171=ORIENTED_EDGE('',*,*,#14358,.F.);
#19172=ORIENTED_EDGE('',*,*,#14359,.F.);
#19173=ORIENTED_EDGE('',*,*,#14360,.T.);
#19174=ORIENTED_EDGE('',*,*,#13660,.F.);
#19175=ORIENTED_EDGE('',*,*,#14361,.F.);
#19176=ORIENTED_EDGE('',*,*,#14362,.F.);
#19177=ORIENTED_EDGE('',*,*,#14363,.F.);
#19178=ORIENTED_EDGE('',*,*,#14358,.T.);
#19179=ORIENTED_EDGE('',*,*,#14364,.F.);
#19180=ORIENTED_EDGE('',*,*,#14365,.F.);
#19181=ORIENTED_EDGE('',*,*,#14366,.F.);
#19182=ORIENTED_EDGE('',*,*,#14362,.T.);
#19183=ORIENTED_EDGE('',*,*,#14367,.F.);
#19184=ORIENTED_EDGE('',*,*,#14365,.T.);
#19185=ORIENTED_EDGE('',*,*,#14368,.F.);
#19186=ORIENTED_EDGE('',*,*,#14344,.F.);
#19187=ORIENTED_EDGE('',*,*,#14369,.F.);
#19188=ORIENTED_EDGE('',*,*,#14233,.T.);
#19189=ORIENTED_EDGE('',*,*,#14214,.T.);
#19190=ORIENTED_EDGE('',*,*,#14370,.T.);
#19191=ORIENTED_EDGE('',*,*,#14371,.T.);
#19192=ORIENTED_EDGE('',*,*,#14372,.T.);
#19193=ORIENTED_EDGE('',*,*,#14372,.F.);
#19194=ORIENTED_EDGE('',*,*,#14373,.T.);
#19195=ORIENTED_EDGE('',*,*,#14374,.T.);
#19196=ORIENTED_EDGE('',*,*,#14375,.F.);
#19197=ORIENTED_EDGE('',*,*,#14376,.T.);
#19198=ORIENTED_EDGE('',*,*,#14377,.F.);
#19199=ORIENTED_EDGE('',*,*,#14374,.F.);
#19200=ORIENTED_EDGE('',*,*,#14378,.T.);
#19201=ORIENTED_EDGE('',*,*,#13648,.F.);
#19202=ORIENTED_EDGE('',*,*,#13651,.F.);
#19203=ORIENTED_EDGE('',*,*,#14379,.T.);
#19204=ORIENTED_EDGE('',*,*,#14380,.T.);
#19205=ORIENTED_EDGE('',*,*,#14376,.F.);
#19206=ORIENTED_EDGE('',*,*,#14381,.F.);
#19207=ORIENTED_EDGE('',*,*,#14382,.T.);
#19208=ORIENTED_EDGE('',*,*,#14383,.T.);
#19209=ORIENTED_EDGE('',*,*,#14379,.F.);
#19210=ORIENTED_EDGE('',*,*,#14384,.F.);
#19211=ORIENTED_EDGE('',*,*,#14385,.T.);
#19212=ORIENTED_EDGE('',*,*,#14386,.T.);
#19213=ORIENTED_EDGE('',*,*,#14382,.F.);
#19214=ORIENTED_EDGE('',*,*,#14387,.F.);
#19215=ORIENTED_EDGE('',*,*,#14385,.F.);
#19216=ORIENTED_EDGE('',*,*,#14388,.T.);
#19217=ORIENTED_EDGE('',*,*,#14389,.T.);
#19218=ORIENTED_EDGE('',*,*,#14390,.F.);
#19219=ORIENTED_EDGE('',*,*,#14391,.T.);
#19220=ORIENTED_EDGE('',*,*,#14392,.T.);
#19221=ORIENTED_EDGE('',*,*,#14389,.F.);
#19222=ORIENTED_EDGE('',*,*,#14393,.F.);
#19223=ORIENTED_EDGE('',*,*,#14394,.T.);
#19224=ORIENTED_EDGE('',*,*,#14395,.T.);
#19225=ORIENTED_EDGE('',*,*,#14391,.F.);
#19226=ORIENTED_EDGE('',*,*,#14396,.F.);
#19227=ORIENTED_EDGE('',*,*,#14397,.T.);
#19228=ORIENTED_EDGE('',*,*,#14398,.T.);
#19229=ORIENTED_EDGE('',*,*,#14394,.F.);
#19230=ORIENTED_EDGE('',*,*,#14399,.F.);
#19231=ORIENTED_EDGE('',*,*,#14397,.F.);
#19232=ORIENTED_EDGE('',*,*,#14400,.T.);
#19233=ORIENTED_EDGE('',*,*,#14401,.T.);
#19234=ORIENTED_EDGE('',*,*,#14402,.F.);
#19235=ORIENTED_EDGE('',*,*,#13654,.F.);
#19236=ORIENTED_EDGE('',*,*,#13657,.F.);
#19237=ORIENTED_EDGE('',*,*,#14401,.F.);
#19238=ORIENTED_EDGE('',*,*,#14403,.T.);
#19239=ORIENTED_EDGE('',*,*,#14404,.T.);
#19240=ORIENTED_EDGE('',*,*,#14405,.F.);
#19241=ORIENTED_EDGE('',*,*,#14404,.F.);
#19242=ORIENTED_EDGE('',*,*,#14406,.T.);
#19243=ORIENTED_EDGE('',*,*,#14407,.T.);
#19244=ORIENTED_EDGE('',*,*,#14408,.F.);
#19245=ORIENTED_EDGE('',*,*,#14407,.F.);
#19246=ORIENTED_EDGE('',*,*,#14409,.T.);
#19247=ORIENTED_EDGE('',*,*,#14410,.T.);
#19248=ORIENTED_EDGE('',*,*,#14411,.F.);
#19249=ORIENTED_EDGE('',*,*,#14412,.T.);
#19250=ORIENTED_EDGE('',*,*,#14413,.T.);
#19251=ORIENTED_EDGE('',*,*,#14216,.T.);
#19252=ORIENTED_EDGE('',*,*,#14246,.T.);
#19253=ORIENTED_EDGE('',*,*,#14414,.F.);
#19254=ORIENTED_EDGE('',*,*,#14410,.F.);
#19255=ORIENTED_EDGE('',*,*,#14415,.T.);
#19256=ORIENTED_EDGE('',*,*,#14221,.F.);
#19257=ORIENTED_EDGE('',*,*,#14220,.F.);
#19258=ORIENTED_EDGE('',*,*,#14413,.F.);
#19259=ORIENTED_EDGE('',*,*,#14416,.T.);
#19260=ORIENTED_EDGE('',*,*,#14417,.F.);
#19261=ORIENTED_EDGE('',*,*,#13652,.T.);
#19262=ORIENTED_EDGE('',*,*,#14418,.T.);
#19263=ORIENTED_EDGE('',*,*,#14419,.T.);
#19264=ORIENTED_EDGE('',*,*,#14417,.T.);
#19265=ORIENTED_EDGE('',*,*,#14420,.T.);
#19266=ORIENTED_EDGE('',*,*,#14421,.F.);
#19267=ORIENTED_EDGE('',*,*,#14418,.F.);
#19268=ORIENTED_EDGE('',*,*,#14422,.T.);
#19269=ORIENTED_EDGE('',*,*,#14423,.T.);
#19270=ORIENTED_EDGE('',*,*,#14424,.F.);
#19271=ORIENTED_EDGE('',*,*,#13698,.F.);
#19272=ORIENTED_EDGE('',*,*,#14425,.T.);
#19273=ORIENTED_EDGE('',*,*,#14426,.F.);
#19274=ORIENTED_EDGE('',*,*,#14427,.F.);
#19275=ORIENTED_EDGE('',*,*,#14428,.T.);
#19276=ORIENTED_EDGE('',*,*,#14426,.T.);
#19277=ORIENTED_EDGE('',*,*,#14429,.T.);
#19278=ORIENTED_EDGE('',*,*,#14430,.T.);
#19279=ORIENTED_EDGE('',*,*,#14370,.F.);
#19280=ORIENTED_EDGE('',*,*,#14224,.F.);
#19281=ORIENTED_EDGE('',*,*,#14229,.T.);
#19282=ORIENTED_EDGE('',*,*,#14431,.T.);
#19283=ORIENTED_EDGE('',*,*,#14427,.T.);
#19284=ORIENTED_EDGE('',*,*,#13646,.T.);
#19285=ORIENTED_EDGE('',*,*,#14432,.F.);
#19286=ORIENTED_EDGE('',*,*,#14423,.F.);
#19287=ORIENTED_EDGE('',*,*,#14433,.T.);
#19288=ORIENTED_EDGE('',*,*,#14434,.T.);
#19289=ORIENTED_EDGE('',*,*,#14435,.F.);
#19290=ORIENTED_EDGE('',*,*,#14360,.F.);
#19291=ORIENTED_EDGE('',*,*,#14436,.F.);
#19292=ORIENTED_EDGE('',*,*,#14437,.T.);
#19293=ORIENTED_EDGE('',*,*,#14438,.F.);
#19294=ORIENTED_EDGE('',*,*,#14439,.F.);
#19295=ORIENTED_EDGE('',*,*,#14440,.F.);
#19296=ORIENTED_EDGE('',*,*,#14355,.T.);
#19297=ORIENTED_EDGE('',*,*,#14245,.F.);
#19298=ORIENTED_EDGE('',*,*,#14244,.F.);
#19299=ORIENTED_EDGE('',*,*,#14240,.T.);
#19300=ORIENTED_EDGE('',*,*,#13709,.T.);
#19301=ORIENTED_EDGE('',*,*,#14441,.T.);
#19302=ORIENTED_EDGE('',*,*,#14436,.T.);
#19303=ORIENTED_EDGE('',*,*,#14359,.T.);
#19304=ORIENTED_EDGE('',*,*,#14363,.T.);
#19305=ORIENTED_EDGE('',*,*,#14366,.T.);
#19306=ORIENTED_EDGE('',*,*,#14367,.T.);
#19307=ORIENTED_EDGE('',*,*,#14343,.F.);
#19308=ORIENTED_EDGE('',*,*,#14347,.T.);
#19309=ORIENTED_EDGE('',*,*,#14350,.T.);
#19310=ORIENTED_EDGE('',*,*,#14353,.T.);
#19311=ORIENTED_EDGE('',*,*,#14356,.T.);
#19312=ORIENTED_EDGE('',*,*,#14440,.T.);
#19313=ORIENTED_EDGE('',*,*,#14442,.T.);
#19314=ORIENTED_EDGE('',*,*,#14443,.T.);
#19315=ORIENTED_EDGE('',*,*,#14249,.T.);
#19316=ORIENTED_EDGE('',*,*,#14238,.F.);
#19317=ORIENTED_EDGE('',*,*,#14234,.F.);
#19318=ORIENTED_EDGE('',*,*,#14369,.T.);
#19319=ORIENTED_EDGE('',*,*,#14375,.T.);
#19320=ORIENTED_EDGE('',*,*,#14377,.T.);
#19321=ORIENTED_EDGE('',*,*,#14380,.F.);
#19322=ORIENTED_EDGE('',*,*,#14383,.F.);
#19323=ORIENTED_EDGE('',*,*,#14386,.F.);
#19324=ORIENTED_EDGE('',*,*,#14390,.T.);
#19325=ORIENTED_EDGE('',*,*,#14392,.F.);
#19326=ORIENTED_EDGE('',*,*,#14395,.F.);
#19327=ORIENTED_EDGE('',*,*,#14398,.F.);
#19328=ORIENTED_EDGE('',*,*,#14402,.T.);
#19329=ORIENTED_EDGE('',*,*,#14405,.T.);
#19330=ORIENTED_EDGE('',*,*,#14408,.T.);
#19331=ORIENTED_EDGE('',*,*,#14411,.T.);
#19332=ORIENTED_EDGE('',*,*,#14414,.T.);
#19333=ORIENTED_EDGE('',*,*,#14444,.F.);
#19334=ORIENTED_EDGE('',*,*,#14250,.T.);
#19335=ORIENTED_EDGE('',*,*,#14443,.F.);
#19336=ORIENTED_EDGE('',*,*,#14445,.F.);
#19337=ORIENTED_EDGE('',*,*,#14368,.T.);
#19338=ORIENTED_EDGE('',*,*,#14364,.T.);
#19339=ORIENTED_EDGE('',*,*,#14361,.T.);
#19340=ORIENTED_EDGE('',*,*,#14357,.T.);
#19341=ORIENTED_EDGE('',*,*,#14435,.T.);
#19342=ORIENTED_EDGE('',*,*,#14446,.T.);
#19343=ORIENTED_EDGE('',*,*,#14447,.T.);
#19344=ORIENTED_EDGE('',*,*,#14448,.T.);
#19345=ORIENTED_EDGE('',*,*,#14449,.T.);
#19346=ORIENTED_EDGE('',*,*,#14450,.T.);
#19347=ORIENTED_EDGE('',*,*,#14451,.T.);
#19348=ORIENTED_EDGE('',*,*,#14452,.T.);
#19349=ORIENTED_EDGE('',*,*,#14453,.T.);
#19350=ORIENTED_EDGE('',*,*,#14454,.T.);
#19351=ORIENTED_EDGE('',*,*,#14455,.T.);
#19352=ORIENTED_EDGE('',*,*,#14456,.T.);
#19353=ORIENTED_EDGE('',*,*,#14457,.T.);
#19354=ORIENTED_EDGE('',*,*,#14458,.T.);
#19355=ORIENTED_EDGE('',*,*,#14459,.T.);
#19356=ORIENTED_EDGE('',*,*,#14460,.T.);
#19357=ORIENTED_EDGE('',*,*,#14461,.T.);
#19358=ORIENTED_EDGE('',*,*,#14462,.T.);
#19359=ORIENTED_EDGE('',*,*,#14463,.T.);
#19360=ORIENTED_EDGE('',*,*,#14464,.T.);
#19361=ORIENTED_EDGE('',*,*,#14465,.T.);
#19362=ORIENTED_EDGE('',*,*,#14466,.T.);
#19363=ORIENTED_EDGE('',*,*,#14467,.T.);
#19364=ORIENTED_EDGE('',*,*,#14468,.T.);
#19365=ORIENTED_EDGE('',*,*,#14469,.T.);
#19366=ORIENTED_EDGE('',*,*,#14470,.T.);
#19367=ORIENTED_EDGE('',*,*,#14471,.T.);
#19368=ORIENTED_EDGE('',*,*,#14472,.T.);
#19369=ORIENTED_EDGE('',*,*,#14473,.T.);
#19370=ORIENTED_EDGE('',*,*,#14474,.T.);
#19371=ORIENTED_EDGE('',*,*,#14475,.T.);
#19372=ORIENTED_EDGE('',*,*,#14476,.T.);
#19373=ORIENTED_EDGE('',*,*,#14477,.T.);
#19374=ORIENTED_EDGE('',*,*,#14478,.T.);
#19375=ORIENTED_EDGE('',*,*,#14479,.T.);
#19376=ORIENTED_EDGE('',*,*,#14480,.T.);
#19377=ORIENTED_EDGE('',*,*,#14481,.T.);
#19378=ORIENTED_EDGE('',*,*,#14482,.T.);
#19379=ORIENTED_EDGE('',*,*,#14438,.T.);
#19380=ORIENTED_EDGE('',*,*,#14354,.T.);
#19381=ORIENTED_EDGE('',*,*,#14351,.T.);
#19382=ORIENTED_EDGE('',*,*,#14348,.T.);
#19383=ORIENTED_EDGE('',*,*,#14345,.T.);
#19384=ORIENTED_EDGE('',*,*,#14341,.F.);
#19385=ORIENTED_EDGE('',*,*,#14340,.F.);
#19386=ORIENTED_EDGE('',*,*,#14338,.F.);
#19387=ORIENTED_EDGE('',*,*,#14336,.F.);
#19388=ORIENTED_EDGE('',*,*,#14334,.F.);
#19389=ORIENTED_EDGE('',*,*,#14332,.F.);
#19390=ORIENTED_EDGE('',*,*,#14330,.F.);
#19391=ORIENTED_EDGE('',*,*,#14328,.F.);
#19392=ORIENTED_EDGE('',*,*,#14326,.F.);
#19393=ORIENTED_EDGE('',*,*,#14324,.F.);
#19394=ORIENTED_EDGE('',*,*,#14322,.F.);
#19395=ORIENTED_EDGE('',*,*,#14320,.F.);
#19396=ORIENTED_EDGE('',*,*,#14318,.F.);
#19397=ORIENTED_EDGE('',*,*,#14316,.F.);
#19398=ORIENTED_EDGE('',*,*,#14314,.F.);
#19399=ORIENTED_EDGE('',*,*,#14312,.F.);
#19400=ORIENTED_EDGE('',*,*,#14310,.F.);
#19401=ORIENTED_EDGE('',*,*,#14308,.F.);
#19402=ORIENTED_EDGE('',*,*,#14306,.F.);
#19403=ORIENTED_EDGE('',*,*,#14304,.F.);
#19404=ORIENTED_EDGE('',*,*,#14302,.F.);
#19405=ORIENTED_EDGE('',*,*,#14300,.F.);
#19406=ORIENTED_EDGE('',*,*,#14298,.F.);
#19407=ORIENTED_EDGE('',*,*,#14296,.F.);
#19408=ORIENTED_EDGE('',*,*,#14294,.F.);
#19409=ORIENTED_EDGE('',*,*,#14292,.F.);
#19410=ORIENTED_EDGE('',*,*,#14290,.F.);
#19411=ORIENTED_EDGE('',*,*,#14288,.F.);
#19412=ORIENTED_EDGE('',*,*,#14286,.F.);
#19413=ORIENTED_EDGE('',*,*,#14284,.F.);
#19414=ORIENTED_EDGE('',*,*,#14282,.F.);
#19415=ORIENTED_EDGE('',*,*,#14280,.F.);
#19416=ORIENTED_EDGE('',*,*,#14278,.F.);
#19417=ORIENTED_EDGE('',*,*,#14276,.F.);
#19418=ORIENTED_EDGE('',*,*,#14274,.F.);
#19419=ORIENTED_EDGE('',*,*,#14272,.F.);
#19420=ORIENTED_EDGE('',*,*,#14270,.F.);
#19421=ORIENTED_EDGE('',*,*,#14268,.F.);
#19422=ORIENTED_EDGE('',*,*,#14266,.F.);
#19423=ORIENTED_EDGE('',*,*,#14264,.F.);
#19424=ORIENTED_EDGE('',*,*,#14262,.F.);
#19425=ORIENTED_EDGE('',*,*,#14260,.F.);
#19426=ORIENTED_EDGE('',*,*,#14258,.F.);
#19427=ORIENTED_EDGE('',*,*,#14256,.F.);
#19428=ORIENTED_EDGE('',*,*,#14253,.F.);
#19429=ORIENTED_EDGE('',*,*,#14430,.F.);
#19430=ORIENTED_EDGE('',*,*,#14429,.F.);
#19431=ORIENTED_EDGE('',*,*,#14425,.F.);
#19432=ORIENTED_EDGE('',*,*,#13697,.F.);
#19433=ORIENTED_EDGE('',*,*,#14483,.F.);
#19434=ORIENTED_EDGE('',*,*,#14484,.F.);
#19435=ORIENTED_EDGE('',*,*,#14485,.F.);
#19436=ORIENTED_EDGE('',*,*,#14486,.F.);
#19437=ORIENTED_EDGE('',*,*,#14487,.F.);
#19438=ORIENTED_EDGE('',*,*,#14488,.T.);
#19439=ORIENTED_EDGE('',*,*,#14489,.F.);
#19440=ORIENTED_EDGE('',*,*,#14490,.T.);
#19441=ORIENTED_EDGE('',*,*,#14491,.F.);
#19442=ORIENTED_EDGE('',*,*,#14492,.F.);
#19443=ORIENTED_EDGE('',*,*,#14493,.F.);
#19444=ORIENTED_EDGE('',*,*,#14494,.F.);
#19445=ORIENTED_EDGE('',*,*,#14495,.F.);
#19446=ORIENTED_EDGE('',*,*,#14433,.F.);
#19447=ORIENTED_EDGE('',*,*,#14422,.F.);
#19448=ORIENTED_EDGE('',*,*,#14420,.F.);
#19449=ORIENTED_EDGE('',*,*,#14416,.F.);
#19450=ORIENTED_EDGE('',*,*,#14412,.F.);
#19451=ORIENTED_EDGE('',*,*,#14409,.F.);
#19452=ORIENTED_EDGE('',*,*,#14406,.F.);
#19453=ORIENTED_EDGE('',*,*,#14403,.F.);
#19454=ORIENTED_EDGE('',*,*,#14400,.F.);
#19455=ORIENTED_EDGE('',*,*,#14399,.T.);
#19456=ORIENTED_EDGE('',*,*,#14396,.T.);
#19457=ORIENTED_EDGE('',*,*,#14393,.T.);
#19458=ORIENTED_EDGE('',*,*,#14388,.F.);
#19459=ORIENTED_EDGE('',*,*,#14387,.T.);
#19460=ORIENTED_EDGE('',*,*,#14384,.T.);
#19461=ORIENTED_EDGE('',*,*,#14381,.T.);
#19462=ORIENTED_EDGE('',*,*,#14378,.F.);
#19463=ORIENTED_EDGE('',*,*,#14373,.F.);
#19464=ORIENTED_EDGE('',*,*,#14371,.F.);
#19465=ORIENTED_EDGE('',*,*,#14496,.F.);
#19466=ORIENTED_EDGE('',*,*,#14497,.T.);
#19467=ORIENTED_EDGE('',*,*,#14490,.F.);
#19468=ORIENTED_EDGE('',*,*,#14498,.F.);
#19469=ORIENTED_EDGE('',*,*,#14499,.T.);
#19470=ORIENTED_EDGE('',*,*,#14500,.T.);
#19471=ORIENTED_EDGE('',*,*,#14486,.T.);
#19472=ORIENTED_EDGE('',*,*,#14501,.F.);
#19473=ORIENTED_EDGE('',*,*,#14502,.T.);
#19474=ORIENTED_EDGE('',*,*,#14501,.T.);
#19475=ORIENTED_EDGE('',*,*,#14485,.T.);
#19476=ORIENTED_EDGE('',*,*,#14503,.F.);
#19477=ORIENTED_EDGE('',*,*,#13637,.F.);
#19478=ORIENTED_EDGE('',*,*,#14504,.T.);
#19479=ORIENTED_EDGE('',*,*,#14503,.T.);
#19480=ORIENTED_EDGE('',*,*,#14484,.T.);
#19481=ORIENTED_EDGE('',*,*,#14505,.F.);
#19482=ORIENTED_EDGE('',*,*,#14506,.T.);
#19483=ORIENTED_EDGE('',*,*,#14507,.F.);
#19484=ORIENTED_EDGE('',*,*,#14487,.T.);
#19485=ORIENTED_EDGE('',*,*,#14500,.F.);
#19486=ORIENTED_EDGE('',*,*,#14508,.F.);
#19487=ORIENTED_EDGE('',*,*,#14509,.T.);
#19488=ORIENTED_EDGE('',*,*,#14510,.F.);
#19489=ORIENTED_EDGE('',*,*,#14480,.F.);
#19490=ORIENTED_EDGE('',*,*,#14511,.F.);
#19491=ORIENTED_EDGE('',*,*,#14512,.T.);
#19492=ORIENTED_EDGE('',*,*,#14513,.F.);
#19493=ORIENTED_EDGE('',*,*,#14478,.F.);
#19494=ORIENTED_EDGE('',*,*,#14513,.T.);
#19495=ORIENTED_EDGE('',*,*,#14514,.T.);
#19496=ORIENTED_EDGE('',*,*,#14508,.T.);
#19497=ORIENTED_EDGE('',*,*,#14479,.F.);
#19498=ORIENTED_EDGE('',*,*,#14510,.T.);
#19499=ORIENTED_EDGE('',*,*,#14515,.T.);
#19500=ORIENTED_EDGE('',*,*,#14516,.T.);
#19501=ORIENTED_EDGE('',*,*,#14481,.F.);
#19502=ORIENTED_EDGE('',*,*,#14516,.F.);
#19503=ORIENTED_EDGE('',*,*,#14517,.T.);
#19504=ORIENTED_EDGE('',*,*,#14505,.T.);
#19505=ORIENTED_EDGE('',*,*,#14483,.T.);
#19506=ORIENTED_EDGE('',*,*,#13696,.T.);
#19507=ORIENTED_EDGE('',*,*,#13702,.T.);
#19508=ORIENTED_EDGE('',*,*,#14445,.T.);
#19509=ORIENTED_EDGE('',*,*,#14442,.F.);
#19510=ORIENTED_EDGE('',*,*,#14439,.T.);
#19511=ORIENTED_EDGE('',*,*,#14482,.F.);
#19512=ORIENTED_EDGE('',*,*,#14518,.T.);
#19513=ORIENTED_EDGE('',*,*,#14519,.F.);
#19514=ORIENTED_EDGE('',*,*,#14476,.F.);
#19515=ORIENTED_EDGE('',*,*,#14520,.F.);
#19516=ORIENTED_EDGE('',*,*,#14521,.T.);
#19517=ORIENTED_EDGE('',*,*,#14522,.F.);
#19518=ORIENTED_EDGE('',*,*,#14474,.F.);
#19519=ORIENTED_EDGE('',*,*,#14523,.F.);
#19520=ORIENTED_EDGE('',*,*,#14522,.T.);
#19521=ORIENTED_EDGE('',*,*,#14524,.T.);
#19522=ORIENTED_EDGE('',*,*,#14520,.T.);
#19523=ORIENTED_EDGE('',*,*,#14475,.F.);
#19524=ORIENTED_EDGE('',*,*,#14525,.T.);
#19525=ORIENTED_EDGE('',*,*,#14526,.F.);
#19526=ORIENTED_EDGE('',*,*,#14472,.F.);
#19527=ORIENTED_EDGE('',*,*,#14527,.F.);
#19528=ORIENTED_EDGE('',*,*,#14528,.T.);
#19529=ORIENTED_EDGE('',*,*,#14529,.F.);
#19530=ORIENTED_EDGE('',*,*,#14470,.F.);
#19531=ORIENTED_EDGE('',*,*,#14530,.F.);
#19532=ORIENTED_EDGE('',*,*,#14529,.T.);
#19533=ORIENTED_EDGE('',*,*,#14531,.T.);
#19534=ORIENTED_EDGE('',*,*,#14527,.T.);
#19535=ORIENTED_EDGE('',*,*,#14471,.F.);
#19536=ORIENTED_EDGE('',*,*,#14526,.T.);
#19537=ORIENTED_EDGE('',*,*,#14532,.T.);
#19538=ORIENTED_EDGE('',*,*,#14523,.T.);
#19539=ORIENTED_EDGE('',*,*,#14473,.F.);
#19540=ORIENTED_EDGE('',*,*,#14533,.T.);
#19541=ORIENTED_EDGE('',*,*,#14534,.F.);
#19542=ORIENTED_EDGE('',*,*,#14468,.F.);
#19543=ORIENTED_EDGE('',*,*,#14535,.F.);
#19544=ORIENTED_EDGE('',*,*,#14536,.T.);
#19545=ORIENTED_EDGE('',*,*,#14537,.F.);
#19546=ORIENTED_EDGE('',*,*,#14466,.F.);
#19547=ORIENTED_EDGE('',*,*,#14538,.F.);
#19548=ORIENTED_EDGE('',*,*,#14537,.T.);
#19549=ORIENTED_EDGE('',*,*,#14539,.T.);
#19550=ORIENTED_EDGE('',*,*,#14535,.T.);
#19551=ORIENTED_EDGE('',*,*,#14467,.F.);
#19552=ORIENTED_EDGE('',*,*,#14540,.F.);
#19553=ORIENTED_EDGE('',*,*,#14541,.T.);
#19554=ORIENTED_EDGE('',*,*,#14542,.T.);
#19555=ORIENTED_EDGE('',*,*,#14464,.F.);
#19556=ORIENTED_EDGE('',*,*,#14542,.F.);
#19557=ORIENTED_EDGE('',*,*,#14543,.T.);
#19558=ORIENTED_EDGE('',*,*,#14538,.T.);
#19559=ORIENTED_EDGE('',*,*,#14465,.F.);
#19560=ORIENTED_EDGE('',*,*,#14544,.T.);
#19561=ORIENTED_EDGE('',*,*,#14545,.F.);
#19562=ORIENTED_EDGE('',*,*,#14462,.F.);
#19563=ORIENTED_EDGE('',*,*,#14546,.F.);
#19564=ORIENTED_EDGE('',*,*,#14547,.T.);
#19565=ORIENTED_EDGE('',*,*,#14548,.F.);
#19566=ORIENTED_EDGE('',*,*,#14460,.F.);
#19567=ORIENTED_EDGE('',*,*,#14549,.F.);
#19568=ORIENTED_EDGE('',*,*,#14548,.T.);
#19569=ORIENTED_EDGE('',*,*,#14550,.T.);
#19570=ORIENTED_EDGE('',*,*,#14546,.T.);
#19571=ORIENTED_EDGE('',*,*,#14461,.F.);
#19572=ORIENTED_EDGE('',*,*,#14551,.T.);
#19573=ORIENTED_EDGE('',*,*,#14552,.F.);
#19574=ORIENTED_EDGE('',*,*,#14458,.F.);
#19575=ORIENTED_EDGE('',*,*,#14553,.F.);
#19576=ORIENTED_EDGE('',*,*,#14554,.T.);
#19577=ORIENTED_EDGE('',*,*,#14555,.F.);
#19578=ORIENTED_EDGE('',*,*,#14456,.F.);
#19579=ORIENTED_EDGE('',*,*,#14556,.F.);
#19580=ORIENTED_EDGE('',*,*,#14555,.T.);
#19581=ORIENTED_EDGE('',*,*,#14557,.T.);
#19582=ORIENTED_EDGE('',*,*,#14553,.T.);
#19583=ORIENTED_EDGE('',*,*,#14457,.F.);
#19584=ORIENTED_EDGE('',*,*,#14552,.T.);
#19585=ORIENTED_EDGE('',*,*,#14558,.T.);
#19586=ORIENTED_EDGE('',*,*,#14549,.T.);
#19587=ORIENTED_EDGE('',*,*,#14459,.F.);
#19588=ORIENTED_EDGE('',*,*,#14545,.T.);
#19589=ORIENTED_EDGE('',*,*,#14559,.T.);
#19590=ORIENTED_EDGE('',*,*,#14540,.T.);
#19591=ORIENTED_EDGE('',*,*,#14463,.F.);
#19592=ORIENTED_EDGE('',*,*,#14560,.T.);
#19593=ORIENTED_EDGE('',*,*,#14561,.F.);
#19594=ORIENTED_EDGE('',*,*,#14454,.F.);
#19595=ORIENTED_EDGE('',*,*,#14562,.F.);
#19596=ORIENTED_EDGE('',*,*,#14563,.T.);
#19597=ORIENTED_EDGE('',*,*,#14564,.F.);
#19598=ORIENTED_EDGE('',*,*,#14452,.F.);
#19599=ORIENTED_EDGE('',*,*,#14565,.F.);
#19600=ORIENTED_EDGE('',*,*,#14564,.T.);
#19601=ORIENTED_EDGE('',*,*,#14566,.T.);
#19602=ORIENTED_EDGE('',*,*,#14562,.T.);
#19603=ORIENTED_EDGE('',*,*,#14453,.F.);
#19604=ORIENTED_EDGE('',*,*,#14567,.F.);
#19605=ORIENTED_EDGE('',*,*,#14568,.T.);
#19606=ORIENTED_EDGE('',*,*,#14569,.F.);
#19607=ORIENTED_EDGE('',*,*,#14450,.F.);
#19608=ORIENTED_EDGE('',*,*,#14570,.F.);
#19609=ORIENTED_EDGE('',*,*,#14571,.T.);
#19610=ORIENTED_EDGE('',*,*,#14572,.F.);
#19611=ORIENTED_EDGE('',*,*,#14448,.F.);
#19612=ORIENTED_EDGE('',*,*,#14573,.T.);
#19613=ORIENTED_EDGE('',*,*,#14574,.T.);
#19614=ORIENTED_EDGE('',*,*,#14494,.T.);
#19615=ORIENTED_EDGE('',*,*,#14575,.F.);
#19616=ORIENTED_EDGE('',*,*,#14576,.T.);
#19617=ORIENTED_EDGE('',*,*,#14575,.T.);
#19618=ORIENTED_EDGE('',*,*,#14493,.T.);
#19619=ORIENTED_EDGE('',*,*,#14577,.F.);
#19620=ORIENTED_EDGE('',*,*,#13640,.F.);
#19621=ORIENTED_EDGE('',*,*,#14578,.T.);
#19622=ORIENTED_EDGE('',*,*,#14577,.T.);
#19623=ORIENTED_EDGE('',*,*,#14492,.T.);
#19624=ORIENTED_EDGE('',*,*,#14579,.F.);
#19625=ORIENTED_EDGE('',*,*,#14580,.T.);
#19626=ORIENTED_EDGE('',*,*,#14579,.T.);
#19627=ORIENTED_EDGE('',*,*,#14491,.T.);
#19628=ORIENTED_EDGE('',*,*,#14497,.F.);
#19629=ORIENTED_EDGE('',*,*,#14574,.F.);
#19630=ORIENTED_EDGE('',*,*,#14581,.T.);
#19631=ORIENTED_EDGE('',*,*,#14582,.T.);
#19632=ORIENTED_EDGE('',*,*,#14446,.F.);
#19633=ORIENTED_EDGE('',*,*,#14437,.F.);
#19634=ORIENTED_EDGE('',*,*,#14441,.F.);
#19635=ORIENTED_EDGE('',*,*,#13708,.F.);
#19636=ORIENTED_EDGE('',*,*,#13704,.F.);
#19637=ORIENTED_EDGE('',*,*,#14434,.F.);
#19638=ORIENTED_EDGE('',*,*,#14495,.T.);
#19639=ORIENTED_EDGE('',*,*,#14582,.F.);
#19640=ORIENTED_EDGE('',*,*,#14583,.T.);
#19641=ORIENTED_EDGE('',*,*,#14570,.T.);
#19642=ORIENTED_EDGE('',*,*,#14447,.F.);
#19643=ORIENTED_EDGE('',*,*,#14572,.T.);
#19644=ORIENTED_EDGE('',*,*,#14584,.T.);
#19645=ORIENTED_EDGE('',*,*,#14567,.T.);
#19646=ORIENTED_EDGE('',*,*,#14449,.F.);
#19647=ORIENTED_EDGE('',*,*,#14569,.T.);
#19648=ORIENTED_EDGE('',*,*,#14585,.T.);
#19649=ORIENTED_EDGE('',*,*,#14565,.T.);
#19650=ORIENTED_EDGE('',*,*,#14451,.F.);
#19651=ORIENTED_EDGE('',*,*,#14561,.T.);
#19652=ORIENTED_EDGE('',*,*,#14586,.T.);
#19653=ORIENTED_EDGE('',*,*,#14556,.T.);
#19654=ORIENTED_EDGE('',*,*,#14455,.F.);
#19655=ORIENTED_EDGE('',*,*,#14534,.T.);
#19656=ORIENTED_EDGE('',*,*,#14587,.T.);
#19657=ORIENTED_EDGE('',*,*,#14530,.T.);
#19658=ORIENTED_EDGE('',*,*,#14469,.F.);
#19659=ORIENTED_EDGE('',*,*,#14519,.T.);
#19660=ORIENTED_EDGE('',*,*,#14588,.T.);
#19661=ORIENTED_EDGE('',*,*,#14511,.T.);
#19662=ORIENTED_EDGE('',*,*,#14477,.F.);
#19663=ORIENTED_EDGE('',*,*,#14488,.F.);
#19664=ORIENTED_EDGE('',*,*,#14507,.T.);
#19665=ORIENTED_EDGE('',*,*,#14589,.F.);
#19666=ORIENTED_EDGE('',*,*,#14590,.F.);
#19667=ORIENTED_EDGE('',*,*,#14489,.T.);
#19668=ORIENTED_EDGE('',*,*,#14590,.T.);
#19669=ORIENTED_EDGE('',*,*,#14591,.T.);
#19670=ORIENTED_EDGE('',*,*,#14498,.T.);
#19671=ORIENTED_EDGE('',*,*,#13643,.F.);
#19672=ORIENTED_EDGE('',*,*,#14591,.F.);
#19673=ORIENTED_EDGE('',*,*,#14589,.T.);
#19674=ORIENTED_EDGE('',*,*,#14506,.F.);
#19675=ORIENTED_EDGE('',*,*,#14499,.F.);
#19676=ORIENTED_EDGE('',*,*,#14502,.F.);
#19677=ORIENTED_EDGE('',*,*,#14504,.F.);
#19678=ORIENTED_EDGE('',*,*,#14517,.F.);
#19679=ORIENTED_EDGE('',*,*,#14515,.F.);
#19680=ORIENTED_EDGE('',*,*,#14509,.F.);
#19681=ORIENTED_EDGE('',*,*,#14514,.F.);
#19682=ORIENTED_EDGE('',*,*,#14512,.F.);
#19683=ORIENTED_EDGE('',*,*,#14588,.F.);
#19684=ORIENTED_EDGE('',*,*,#14518,.F.);
#19685=ORIENTED_EDGE('',*,*,#14524,.F.);
#19686=ORIENTED_EDGE('',*,*,#14521,.F.);
#19687=ORIENTED_EDGE('',*,*,#14532,.F.);
#19688=ORIENTED_EDGE('',*,*,#14525,.F.);
#19689=ORIENTED_EDGE('',*,*,#14531,.F.);
#19690=ORIENTED_EDGE('',*,*,#14528,.F.);
#19691=ORIENTED_EDGE('',*,*,#14587,.F.);
#19692=ORIENTED_EDGE('',*,*,#14533,.F.);
#19693=ORIENTED_EDGE('',*,*,#14539,.F.);
#19694=ORIENTED_EDGE('',*,*,#14536,.F.);
#19695=ORIENTED_EDGE('',*,*,#14543,.F.);
#19696=ORIENTED_EDGE('',*,*,#14541,.F.);
#19697=ORIENTED_EDGE('',*,*,#14559,.F.);
#19698=ORIENTED_EDGE('',*,*,#14544,.F.);
#19699=ORIENTED_EDGE('',*,*,#14550,.F.);
#19700=ORIENTED_EDGE('',*,*,#14547,.F.);
#19701=ORIENTED_EDGE('',*,*,#14558,.F.);
#19702=ORIENTED_EDGE('',*,*,#14551,.F.);
#19703=ORIENTED_EDGE('',*,*,#14557,.F.);
#19704=ORIENTED_EDGE('',*,*,#14554,.F.);
#19705=ORIENTED_EDGE('',*,*,#14586,.F.);
#19706=ORIENTED_EDGE('',*,*,#14560,.F.);
#19707=ORIENTED_EDGE('',*,*,#14566,.F.);
#19708=ORIENTED_EDGE('',*,*,#14563,.F.);
#19709=ORIENTED_EDGE('',*,*,#14585,.F.);
#19710=ORIENTED_EDGE('',*,*,#14568,.F.);
#19711=ORIENTED_EDGE('',*,*,#14584,.F.);
#19712=ORIENTED_EDGE('',*,*,#14571,.F.);
#19713=ORIENTED_EDGE('',*,*,#14583,.F.);
#19714=ORIENTED_EDGE('',*,*,#14581,.F.);
#19715=ORIENTED_EDGE('',*,*,#14573,.F.);
#19716=ORIENTED_EDGE('',*,*,#14576,.F.);
#19717=ORIENTED_EDGE('',*,*,#14578,.F.);
#19718=ORIENTED_EDGE('',*,*,#14580,.F.);
#19719=ORIENTED_EDGE('',*,*,#14496,.T.);
#19720=ORIENTED_EDGE('',*,*,#13986,.T.);
#19721=ORIENTED_EDGE('',*,*,#13984,.T.);
#19722=ORIENTED_EDGE('',*,*,#13982,.T.);
#19723=ORIENTED_EDGE('',*,*,#13980,.T.);
#19724=ORIENTED_EDGE('',*,*,#13978,.T.);
#19725=ORIENTED_EDGE('',*,*,#13976,.T.);
#19726=ORIENTED_EDGE('',*,*,#13974,.T.);
#19727=ORIENTED_EDGE('',*,*,#13972,.T.);
#19728=ORIENTED_EDGE('',*,*,#13970,.T.);
#19729=ORIENTED_EDGE('',*,*,#13968,.T.);
#19730=ORIENTED_EDGE('',*,*,#13966,.T.);
#19731=ORIENTED_EDGE('',*,*,#13964,.T.);
#19732=ORIENTED_EDGE('',*,*,#13962,.T.);
#19733=ORIENTED_EDGE('',*,*,#13960,.T.);
#19734=ORIENTED_EDGE('',*,*,#13958,.T.);
#19735=ORIENTED_EDGE('',*,*,#13956,.T.);
#19736=ORIENTED_EDGE('',*,*,#13954,.T.);
#19737=ORIENTED_EDGE('',*,*,#13952,.T.);
#19738=ORIENTED_EDGE('',*,*,#13950,.T.);
#19739=ORIENTED_EDGE('',*,*,#13948,.T.);
#19740=ORIENTED_EDGE('',*,*,#13946,.T.);
#19741=ORIENTED_EDGE('',*,*,#13944,.T.);
#19742=ORIENTED_EDGE('',*,*,#13942,.T.);
#19743=ORIENTED_EDGE('',*,*,#13940,.T.);
#19744=ORIENTED_EDGE('',*,*,#13938,.T.);
#19745=ORIENTED_EDGE('',*,*,#13936,.T.);
#19746=ORIENTED_EDGE('',*,*,#13934,.T.);
#19747=ORIENTED_EDGE('',*,*,#13932,.T.);
#19748=ORIENTED_EDGE('',*,*,#13930,.T.);
#19749=ORIENTED_EDGE('',*,*,#13928,.T.);
#19750=ORIENTED_EDGE('',*,*,#13926,.T.);
#19751=ORIENTED_EDGE('',*,*,#13924,.T.);
#19752=ORIENTED_EDGE('',*,*,#13922,.T.);
#19753=ORIENTED_EDGE('',*,*,#13920,.T.);
#19754=ORIENTED_EDGE('',*,*,#13918,.T.);
#19755=ORIENTED_EDGE('',*,*,#13916,.T.);
#19756=ORIENTED_EDGE('',*,*,#13914,.T.);
#19757=ORIENTED_EDGE('',*,*,#13912,.T.);
#19758=ORIENTED_EDGE('',*,*,#13910,.T.);
#19759=ORIENTED_EDGE('',*,*,#13908,.T.);
#19760=ORIENTED_EDGE('',*,*,#13906,.T.);
#19761=ORIENTED_EDGE('',*,*,#13904,.T.);
#19762=ORIENTED_EDGE('',*,*,#13902,.T.);
#19763=ORIENTED_EDGE('',*,*,#13899,.T.);
#19764=ORIENTED_EDGE('',*,*,#13991,.T.);
#19765=ORIENTED_EDGE('',*,*,#14056,.F.);
#19766=ORIENTED_EDGE('',*,*,#14592,.F.);
#19767=ORIENTED_EDGE('',*,*,#14593,.T.);
#19768=ORIENTED_EDGE('',*,*,#13992,.T.);
#19769=ORIENTED_EDGE('',*,*,#14593,.F.);
#19770=ORIENTED_EDGE('',*,*,#14594,.F.);
#19771=ORIENTED_EDGE('',*,*,#14595,.T.);
#19772=ORIENTED_EDGE('',*,*,#13993,.T.);
#19773=ORIENTED_EDGE('',*,*,#14595,.F.);
#19774=ORIENTED_EDGE('',*,*,#14596,.F.);
#19775=ORIENTED_EDGE('',*,*,#14059,.T.);
#19776=ORIENTED_EDGE('',*,*,#14055,.T.);
#19777=ORIENTED_EDGE('',*,*,#14596,.T.);
#19778=ORIENTED_EDGE('',*,*,#14594,.T.);
#19779=ORIENTED_EDGE('',*,*,#14592,.T.);
#19780=ORIENTED_EDGE('',*,*,#14247,.F.);
#19781=ORIENTED_EDGE('',*,*,#14158,.F.);
#19782=ORIENTED_EDGE('',*,*,#14231,.T.);
#19783=ORIENTED_EDGE('',*,*,#13705,.T.);
#19784=ORIENTED_EDGE('',*,*,#13707,.T.);
#19785=ORIENTED_EDGE('',*,*,#14239,.T.);
#19786=ORIENTED_EDGE('',*,*,#14243,.F.);
#19787=ORIENTED_EDGE('',*,*,#14415,.F.);
#19788=ORIENTED_EDGE('',*,*,#14419,.F.);
#19789=ORIENTED_EDGE('',*,*,#14421,.T.);
#19790=ORIENTED_EDGE('',*,*,#14432,.T.);
#19791=ORIENTED_EDGE('',*,*,#13703,.T.);
#19792=ORIENTED_EDGE('',*,*,#14230,.T.);
#19793=ORIENTED_EDGE('',*,*,#14222,.F.);
#19794=ORIENTED_EDGE('',*,*,#14232,.F.);
#19795=ORIENTED_EDGE('',*,*,#14237,.F.);
#19796=ORIENTED_EDGE('',*,*,#14248,.T.);
#19797=ORIENTED_EDGE('',*,*,#14444,.T.);
#19798=ORIENTED_EDGE('',*,*,#13701,.T.);
#19799=ORIENTED_EDGE('',*,*,#14252,.T.);
#19800=ORIENTED_EDGE('',*,*,#14161,.F.);
#19801=ORIENTED_EDGE('',*,*,#14251,.T.);
#19802=ORIENTED_EDGE('',*,*,#13699,.T.);
#19803=ORIENTED_EDGE('',*,*,#13695,.T.);
#19804=ORIENTED_EDGE('',*,*,#14424,.T.);
#19805=ORIENTED_EDGE('',*,*,#14428,.F.);
#19806=ORIENTED_EDGE('',*,*,#14431,.F.);
#19807=ORIENTED_EDGE('',*,*,#14228,.F.);
#23895=CYLINDRICAL_SURFACE('',#26593,2.5);
#23896=CYLINDRICAL_SURFACE('',#26596,2.5);
#23897=CYLINDRICAL_SURFACE('',#26599,3.65);
#23898=CYLINDRICAL_SURFACE('',#26604,3.32349999999999);
#23899=CYLINDRICAL_SURFACE('',#26607,3.3235);
#23900=CYLINDRICAL_SURFACE('',#26610,3.32349999999999);
#23901=CYLINDRICAL_SURFACE('',#26613,3.3235);
#23902=CYLINDRICAL_SURFACE('',#26616,2.5);
#23903=CYLINDRICAL_SURFACE('',#26619,2.5);
#23904=CYLINDRICAL_SURFACE('',#26622,3.65);
#23905=CYLINDRICAL_SURFACE('',#26625,0.500000000000006);
#23906=CYLINDRICAL_SURFACE('',#26631,0.5);
#23907=CYLINDRICAL_SURFACE('',#26637,4.);
#23908=CYLINDRICAL_SURFACE('',#26639,4.99995);
#23909=CYLINDRICAL_SURFACE('',#26669,2.3);
#23910=CYLINDRICAL_SURFACE('',#26672,2.3);
#23911=CYLINDRICAL_SURFACE('',#26675,2.3);
#23912=CYLINDRICAL_SURFACE('',#26678,2.3);
#23913=CYLINDRICAL_SURFACE('',#26681,0.5);
#23914=CYLINDRICAL_SURFACE('',#26684,0.5);
#23915=CYLINDRICAL_SURFACE('',#26687,0.5);
#23916=CYLINDRICAL_SURFACE('',#26690,0.5);
#23917=CYLINDRICAL_SURFACE('',#26693,0.5);
#23918=CYLINDRICAL_SURFACE('',#26696,0.5);
#23919=CYLINDRICAL_SURFACE('',#26699,0.5);
#23920=CYLINDRICAL_SURFACE('',#26702,0.5);
#23921=CYLINDRICAL_SURFACE('',#26705,0.5);
#23922=CYLINDRICAL_SURFACE('',#26708,0.5);
#23923=CYLINDRICAL_SURFACE('',#26711,0.5);
#23924=CYLINDRICAL_SURFACE('',#26714,0.5);
#23925=CYLINDRICAL_SURFACE('',#26717,0.5);
#23926=CYLINDRICAL_SURFACE('',#26720,0.5);
#23927=CYLINDRICAL_SURFACE('',#26723,0.5);
#23928=CYLINDRICAL_SURFACE('',#26726,0.5);
#23929=CYLINDRICAL_SURFACE('',#26767,0.450000000000001);
#23930=CYLINDRICAL_SURFACE('',#26770,0.450000000000001);
#23931=CYLINDRICAL_SURFACE('',#26773,0.55);
#23932=CYLINDRICAL_SURFACE('',#26775,2.25);
#23933=CYLINDRICAL_SURFACE('',#26777,0.549999999999998);
#23934=CYLINDRICAL_SURFACE('',#26780,0.55);
#23935=CYLINDRICAL_SURFACE('',#26783,0.55);
#23936=CYLINDRICAL_SURFACE('',#26786,0.55);
#23937=CYLINDRICAL_SURFACE('',#26788,2.25);
#23938=CYLINDRICAL_SURFACE('',#26790,0.55);
#23939=CYLINDRICAL_SURFACE('',#26795,0.550000000000001);
#23940=CYLINDRICAL_SURFACE('',#26797,2.25);
#23941=CYLINDRICAL_SURFACE('',#26799,0.550000000000002);
#23942=CYLINDRICAL_SURFACE('',#26802,0.55);
#23943=CYLINDRICAL_SURFACE('',#26805,0.55);
#23944=CYLINDRICAL_SURFACE('',#26808,0.55);
#23945=CYLINDRICAL_SURFACE('',#26810,2.25);
#23946=CYLINDRICAL_SURFACE('',#26812,0.55);
#23947=CYLINDRICAL_SURFACE('',#26815,0.450000000000001);
#23948=CYLINDRICAL_SURFACE('',#26818,0.450000000000001);
#23949=CYLINDRICAL_SURFACE('',#26857,0.5);
#23950=CYLINDRICAL_SURFACE('',#26872,0.5);
#23951=CYLINDRICAL_SURFACE('',#26875,0.5);
#23952=CYLINDRICAL_SURFACE('',#26878,0.5);
#23953=CYLINDRICAL_SURFACE('',#26880,2.3);
#23954=CYLINDRICAL_SURFACE('',#26882,0.5);
#23955=CYLINDRICAL_SURFACE('',#26885,0.5);
#23956=CYLINDRICAL_SURFACE('',#26888,0.5);
#23957=CYLINDRICAL_SURFACE('',#26891,0.5);
#23958=CYLINDRICAL_SURFACE('',#26893,2.3);
#23959=CYLINDRICAL_SURFACE('',#26895,0.5);
#23960=CYLINDRICAL_SURFACE('',#26900,0.5);
#23961=CYLINDRICAL_SURFACE('',#26902,2.3);
#23962=CYLINDRICAL_SURFACE('',#26904,0.5);
#23963=CYLINDRICAL_SURFACE('',#26907,0.5);
#23964=CYLINDRICAL_SURFACE('',#26910,0.5);
#23965=CYLINDRICAL_SURFACE('',#26913,0.5);
#23966=CYLINDRICAL_SURFACE('',#26915,2.3);
#23967=CYLINDRICAL_SURFACE('',#26917,0.5);
#23968=CYLINDRICAL_SURFACE('',#26920,0.5);
#23969=CYLINDRICAL_SURFACE('',#26923,0.5);
#23970=CYLINDRICAL_SURFACE('',#26931,0.500000000000006);
#23971=CYLINDRICAL_SURFACE('',#26933,2.);
#23972=CYLINDRICAL_SURFACE('',#26941,2.);
#23973=CYLINDRICAL_SURFACE('',#26997,0.450000000000001);
#23974=CYLINDRICAL_SURFACE('',#27000,0.450000000000001);
#23975=CYLINDRICAL_SURFACE('',#27003,0.55);
#23976=CYLINDRICAL_SURFACE('',#27005,2.25);
#23977=CYLINDRICAL_SURFACE('',#27007,0.55);
#23978=CYLINDRICAL_SURFACE('',#27010,0.55);
#23979=CYLINDRICAL_SURFACE('',#27013,0.55);
#23980=CYLINDRICAL_SURFACE('',#27016,0.550000000000002);
#23981=CYLINDRICAL_SURFACE('',#27018,2.25);
#23982=CYLINDRICAL_SURFACE('',#27020,0.55);
#23983=CYLINDRICAL_SURFACE('',#27025,0.55);
#23984=CYLINDRICAL_SURFACE('',#27027,2.25);
#23985=CYLINDRICAL_SURFACE('',#27029,0.55);
#23986=CYLINDRICAL_SURFACE('',#27032,0.55);
#23987=CYLINDRICAL_SURFACE('',#27035,0.55);
#23988=CYLINDRICAL_SURFACE('',#27038,0.549999999999998);
#23989=CYLINDRICAL_SURFACE('',#27040,2.25);
#23990=CYLINDRICAL_SURFACE('',#27042,0.550000000000001);
#23991=CYLINDRICAL_SURFACE('',#27045,0.450000000000001);
#23992=CYLINDRICAL_SURFACE('',#27048,0.450000000000001);
#23993=CYLINDRICAL_SURFACE('',#27119,0.5);
#23994=CYLINDRICAL_SURFACE('',#27121,0.5);
#23995=CYLINDRICAL_SURFACE('',#27126,0.5);
#23996=CYLINDRICAL_SURFACE('',#27128,0.5);
#23997=CYLINDRICAL_SURFACE('',#27130,2.3);
#23998=CYLINDRICAL_SURFACE('',#27132,0.5);
#23999=CYLINDRICAL_SURFACE('',#27134,0.5);
#24000=CYLINDRICAL_SURFACE('',#27138,0.5);
#24001=CYLINDRICAL_SURFACE('',#27140,0.5);
#24002=CYLINDRICAL_SURFACE('',#27142,2.3);
#24003=CYLINDRICAL_SURFACE('',#27146,0.5);
#24004=CYLINDRICAL_SURFACE('',#27148,0.5);
#24005=CYLINDRICAL_SURFACE('',#27150,2.3);
#24006=CYLINDRICAL_SURFACE('',#27152,0.5);
#24007=CYLINDRICAL_SURFACE('',#27154,0.5);
#24008=CYLINDRICAL_SURFACE('',#27159,0.5);
#24009=CYLINDRICAL_SURFACE('',#27161,0.5);
#24010=CYLINDRICAL_SURFACE('',#27163,2.3);
#24011=CYLINDRICAL_SURFACE('',#27165,0.5);
#24012=CYLINDRICAL_SURFACE('',#27167,0.5);
#24013=CYLINDRICAL_SURFACE('',#27184,4.99995);
#24014=CYLINDRICAL_SURFACE('',#27188,5.5);
#24015=CYLINDRICAL_SURFACE('',#27189,5.50000000000001);
#24016=CYLINDRICAL_SURFACE('',#27190,5.5);
#24017=CYLINDRICAL_SURFACE('',#27191,5.49999999999999);
#24454=ADVANCED_FACE('',(#2501),#23895,.F.);
#24455=ADVANCED_FACE('',(#2502),#23896,.F.);
#24456=ADVANCED_FACE('',(#2503),#23897,.F.);
#24457=ADVANCED_FACE('',(#2504),#524,.F.);
#24458=ADVANCED_FACE('',(#2505),#525,.F.);
#24459=ADVANCED_FACE('',(#2506),#23898,.F.);
#24460=ADVANCED_FACE('',(#2507),#23899,.F.);
#24461=ADVANCED_FACE('',(#2508),#23900,.F.);
#24462=ADVANCED_FACE('',(#2509),#23901,.F.);
#24463=ADVANCED_FACE('',(#2510),#23902,.F.);
#24464=ADVANCED_FACE('',(#2511),#23903,.F.);
#24465=ADVANCED_FACE('',(#2512),#23904,.F.);
#24466=ADVANCED_FACE('',(#2513),#23905,.F.);
#24467=ADVANCED_FACE('',(#2514),#526,.F.);
#24468=ADVANCED_FACE('',(#2515),#527,.F.);
#24469=ADVANCED_FACE('',(#2516),#23906,.F.);
#24470=ADVANCED_FACE('',(#2517),#402,.F.);
#24471=ADVANCED_FACE('',(#2518),#23907,.T.);
#24472=ADVANCED_FACE('',(#2519),#23908,.F.);
#24473=ADVANCED_FACE('',(#2520),#1637,.T.);
#24474=ADVANCED_FACE('',(#2521),#1638,.T.);
#24475=ADVANCED_FACE('',(#2522),#1639,.T.);
#24476=ADVANCED_FACE('',(#2523),#1640,.T.);
#24477=ADVANCED_FACE('',(#2524),#1641,.T.);
#24478=ADVANCED_FACE('',(#2525),#1642,.T.);
#24479=ADVANCED_FACE('',(#2526),#1643,.T.);
#24480=ADVANCED_FACE('',(#2527),#1644,.T.);
#24481=ADVANCED_FACE('',(#2528),#1645,.T.);
#24482=ADVANCED_FACE('',(#2529),#1646,.T.);
#24483=ADVANCED_FACE('',(#2530),#1647,.T.);
#24484=ADVANCED_FACE('',(#2531),#1648,.T.);
#24485=ADVANCED_FACE('',(#2532),#1649,.T.);
#24486=ADVANCED_FACE('',(#2533),#1650,.T.);
#24487=ADVANCED_FACE('',(#2534),#1651,.T.);
#24488=ADVANCED_FACE('',(#2535),#1652,.T.);
#24489=ADVANCED_FACE('',(#2536),#1653,.T.);
#24490=ADVANCED_FACE('',(#2537),#1654,.T.);
#24491=ADVANCED_FACE('',(#2538),#1655,.T.);
#24492=ADVANCED_FACE('',(#2539),#1656,.T.);
#24493=ADVANCED_FACE('',(#2540),#1657,.T.);
#24494=ADVANCED_FACE('',(#2541),#23909,.T.);
#24495=ADVANCED_FACE('',(#2542),#23910,.T.);
#24496=ADVANCED_FACE('',(#2543),#23911,.T.);
#24497=ADVANCED_FACE('',(#2544),#23912,.T.);
#24498=ADVANCED_FACE('',(#2545),#23913,.T.);
#24499=ADVANCED_FACE('',(#2546),#23914,.T.);
#24500=ADVANCED_FACE('',(#2547),#23915,.F.);
#24501=ADVANCED_FACE('',(#2548),#23916,.F.);
#24502=ADVANCED_FACE('',(#2549),#23917,.F.);
#24503=ADVANCED_FACE('',(#2550),#23918,.F.);
#24504=ADVANCED_FACE('',(#2551),#23919,.F.);
#24505=ADVANCED_FACE('',(#2552),#23920,.F.);
#24506=ADVANCED_FACE('',(#2553),#23921,.T.);
#24507=ADVANCED_FACE('',(#2554),#23922,.T.);
#24508=ADVANCED_FACE('',(#2555),#23923,.F.);
#24509=ADVANCED_FACE('',(#2556),#23924,.F.);
#24510=ADVANCED_FACE('',(#2557),#23925,.F.);
#24511=ADVANCED_FACE('',(#2558),#23926,.F.);
#24512=ADVANCED_FACE('',(#2559),#23927,.F.);
#24513=ADVANCED_FACE('',(#2560),#23928,.F.);
#24514=ADVANCED_FACE('',(#2561,#1277),#1658,.T.);
#24515=ADVANCED_FACE('',(#2562),#1659,.F.);
#24516=ADVANCED_FACE('',(#2563,#1278),#1660,.T.);
#24517=ADVANCED_FACE('',(#2564),#1661,.F.);
#24518=ADVANCED_FACE('',(#2565),#1662,.F.);
#24519=ADVANCED_FACE('',(#2566),#1663,.F.);
#24520=ADVANCED_FACE('',(#2567),#1664,.F.);
#24521=ADVANCED_FACE('',(#2568),#1665,.F.);
#24522=ADVANCED_FACE('',(#2569),#1666,.F.);
#24523=ADVANCED_FACE('',(#2570),#1667,.F.);
#24524=ADVANCED_FACE('',(#2571),#1668,.F.);
#24525=ADVANCED_FACE('',(#2572),#1669,.F.);
#24526=ADVANCED_FACE('',(#2573),#1670,.F.);
#24527=ADVANCED_FACE('',(#2574),#1671,.F.);
#24528=ADVANCED_FACE('',(#2575),#1672,.F.);
#24529=ADVANCED_FACE('',(#2576),#1673,.T.);
#24530=ADVANCED_FACE('',(#2577,#1279),#1674,.F.);
#24531=ADVANCED_FACE('',(#2578),#1675,.T.);
#24532=ADVANCED_FACE('',(#2579),#23929,.T.);
#24533=ADVANCED_FACE('',(#2580),#1676,.T.);
#24534=ADVANCED_FACE('',(#2581),#23930,.T.);
#24535=ADVANCED_FACE('',(#2582),#1677,.T.);
#24536=ADVANCED_FACE('',(#2583),#23931,.F.);
#24537=ADVANCED_FACE('',(#2584),#23932,.T.);
#24538=ADVANCED_FACE('',(#2585),#23933,.F.);
#24539=ADVANCED_FACE('',(#2586),#1678,.T.);
#24540=ADVANCED_FACE('',(#2587),#23934,.F.);
#24541=ADVANCED_FACE('',(#2588),#1679,.T.);
#24542=ADVANCED_FACE('',(#2589),#23935,.F.);
#24543=ADVANCED_FACE('',(#2590),#1680,.T.);
#24544=ADVANCED_FACE('',(#2591),#23936,.F.);
#24545=ADVANCED_FACE('',(#2592),#23937,.T.);
#24546=ADVANCED_FACE('',(#2593),#23938,.F.);
#24547=ADVANCED_FACE('',(#2594),#1681,.T.);
#24548=ADVANCED_FACE('',(#2595),#1682,.T.);
#24549=ADVANCED_FACE('',(#2596),#1683,.T.);
#24550=ADVANCED_FACE('',(#2597),#23939,.F.);
#24551=ADVANCED_FACE('',(#2598),#23940,.T.);
#24552=ADVANCED_FACE('',(#2599),#23941,.F.);
#24553=ADVANCED_FACE('',(#2600),#1684,.T.);
#24554=ADVANCED_FACE('',(#2601),#23942,.F.);
#24555=ADVANCED_FACE('',(#2602),#1685,.T.);
#24556=ADVANCED_FACE('',(#2603),#23943,.F.);
#24557=ADVANCED_FACE('',(#2604),#1686,.T.);
#24558=ADVANCED_FACE('',(#2605),#23944,.F.);
#24559=ADVANCED_FACE('',(#2606),#23945,.T.);
#24560=ADVANCED_FACE('',(#2607),#23946,.F.);
#24561=ADVANCED_FACE('',(#2608),#1687,.T.);
#24562=ADVANCED_FACE('',(#2609),#23947,.T.);
#24563=ADVANCED_FACE('',(#2610),#1688,.T.);
#24564=ADVANCED_FACE('',(#2611),#23948,.T.);
#24565=ADVANCED_FACE('',(#2612),#1689,.T.);
#24566=ADVANCED_FACE('',(#2613),#1690,.T.);
#24567=ADVANCED_FACE('',(#2614),#1691,.T.);
#24568=ADVANCED_FACE('',(#2615),#1692,.T.);
#24569=ADVANCED_FACE('',(#2616),#1693,.T.);
#24570=ADVANCED_FACE('',(#2617),#1694,.T.);
#24571=ADVANCED_FACE('',(#2618),#1695,.T.);
#24572=ADVANCED_FACE('',(#2619),#1696,.T.);
#24573=ADVANCED_FACE('',(#2620),#1697,.T.);
#24574=ADVANCED_FACE('',(#2621),#1698,.T.);
#24575=ADVANCED_FACE('',(#2622),#1699,.T.);
#24576=ADVANCED_FACE('',(#2623),#1700,.T.);
#24577=ADVANCED_FACE('',(#2624),#1701,.F.);
#24578=ADVANCED_FACE('',(#2625),#1702,.F.);
#24579=ADVANCED_FACE('',(#2626),#1703,.F.);
#24580=ADVANCED_FACE('',(#2627),#23949,.F.);
#24581=ADVANCED_FACE('',(#2628),#1704,.T.);
#24582=ADVANCED_FACE('',(#2629),#1705,.T.);
#24583=ADVANCED_FACE('',(#2630),#1706,.T.);
#24584=ADVANCED_FACE('',(#2631),#1707,.F.);
#24585=ADVANCED_FACE('',(#2632),#1708,.F.);
#24586=ADVANCED_FACE('',(#2633),#1709,.F.);
#24587=ADVANCED_FACE('',(#2634),#1710,.F.);
#24588=ADVANCED_FACE('',(#2635),#1711,.F.);
#24589=ADVANCED_FACE('',(#2636),#1712,.F.);
#24590=ADVANCED_FACE('',(#2637),#1713,.F.);
#24591=ADVANCED_FACE('',(#2638),#1714,.T.);
#24592=ADVANCED_FACE('',(#2639),#1715,.T.);
#24593=ADVANCED_FACE('',(#2640),#23950,.T.);
#24594=ADVANCED_FACE('',(#2641),#1716,.T.);
#24595=ADVANCED_FACE('',(#2642),#23951,.T.);
#24596=ADVANCED_FACE('',(#2643),#1717,.T.);
#24597=ADVANCED_FACE('',(#2644),#23952,.F.);
#24598=ADVANCED_FACE('',(#2645),#23953,.T.);
#24599=ADVANCED_FACE('',(#2646),#23954,.F.);
#24600=ADVANCED_FACE('',(#2647),#1718,.T.);
#24601=ADVANCED_FACE('',(#2648),#23955,.F.);
#24602=ADVANCED_FACE('',(#2649),#1719,.T.);
#24603=ADVANCED_FACE('',(#2650),#23956,.F.);
#24604=ADVANCED_FACE('',(#2651),#1720,.T.);
#24605=ADVANCED_FACE('',(#2652),#23957,.F.);
#24606=ADVANCED_FACE('',(#2653),#23958,.T.);
#24607=ADVANCED_FACE('',(#2654),#23959,.F.);
#24608=ADVANCED_FACE('',(#2655),#1721,.T.);
#24609=ADVANCED_FACE('',(#2656),#1722,.T.);
#24610=ADVANCED_FACE('',(#2657),#1723,.T.);
#24611=ADVANCED_FACE('',(#2658),#23960,.F.);
#24612=ADVANCED_FACE('',(#2659),#23961,.T.);
#24613=ADVANCED_FACE('',(#2660),#23962,.F.);
#24614=ADVANCED_FACE('',(#2661),#1724,.T.);
#24615=ADVANCED_FACE('',(#2662),#23963,.F.);
#24616=ADVANCED_FACE('',(#2663),#1725,.T.);
#24617=ADVANCED_FACE('',(#2664),#23964,.F.);
#24618=ADVANCED_FACE('',(#2665),#1726,.T.);
#24619=ADVANCED_FACE('',(#2666),#23965,.F.);
#24620=ADVANCED_FACE('',(#2667),#23966,.T.);
#24621=ADVANCED_FACE('',(#2668),#23967,.F.);
#24622=ADVANCED_FACE('',(#2669),#1727,.T.);
#24623=ADVANCED_FACE('',(#2670),#23968,.T.);
#24624=ADVANCED_FACE('',(#2671),#1728,.T.);
#24625=ADVANCED_FACE('',(#2672),#23969,.T.);
#24626=ADVANCED_FACE('',(#2673),#1729,.T.);
#24627=ADVANCED_FACE('',(#2674,#1280),#1730,.T.);
#24628=ADVANCED_FACE('',(#2675),#1731,.T.);
#24629=ADVANCED_FACE('',(#2676),#1732,.T.);
#24630=ADVANCED_FACE('',(#2677),#1733,.F.);
#24631=ADVANCED_FACE('',(#2678),#1734,.F.);
#24632=ADVANCED_FACE('',(#2679),#23970,.F.);
#24633=ADVANCED_FACE('',(#2680),#23971,.F.);
#24634=ADVANCED_FACE('',(#2681),#1735,.T.);
#24635=ADVANCED_FACE('',(#2682),#1736,.F.);
#24636=ADVANCED_FACE('',(#2683),#1737,.F.);
#24637=ADVANCED_FACE('',(#2684),#1738,.T.);
#24638=ADVANCED_FACE('',(#2685),#23972,.F.);
#24639=ADVANCED_FACE('',(#2686,#1281),#1739,.F.);
#24640=ADVANCED_FACE('',(#2687),#1740,.F.);
#24641=ADVANCED_FACE('',(#2688),#1741,.F.);
#24642=ADVANCED_FACE('',(#2689),#1742,.T.);
#24643=ADVANCED_FACE('',(#2690),#1743,.F.);
#24644=ADVANCED_FACE('',(#2691),#1744,.F.);
#24645=ADVANCED_FACE('',(#2692),#1745,.F.);
#24646=ADVANCED_FACE('',(#2693,#1282),#1746,.T.);
#24647=ADVANCED_FACE('',(#2694),#1747,.T.);
#24648=ADVANCED_FACE('',(#2695,#1283),#1748,.F.);
#24649=ADVANCED_FACE('',(#2696),#1749,.F.);
#24650=ADVANCED_FACE('',(#2697),#1750,.T.);
#24651=ADVANCED_FACE('',(#2698),#1751,.F.);
#24652=ADVANCED_FACE('',(#2699,#1284),#1752,.F.);
#24653=ADVANCED_FACE('',(#2700),#1753,.T.);
#24654=ADVANCED_FACE('',(#2701),#1754,.T.);
#24655=ADVANCED_FACE('',(#2702),#1755,.F.);
#24656=ADVANCED_FACE('',(#2703),#1756,.F.);
#24657=ADVANCED_FACE('',(#2704),#1757,.F.);
#24658=ADVANCED_FACE('',(#2705),#1758,.F.);
#24659=ADVANCED_FACE('',(#2706),#1759,.F.);
#24660=ADVANCED_FACE('',(#2707),#1760,.F.);
#24661=ADVANCED_FACE('',(#2708),#1761,.F.);
#24662=ADVANCED_FACE('',(#2709),#1762,.F.);
#24663=ADVANCED_FACE('',(#2710),#1763,.F.);
#24664=ADVANCED_FACE('',(#2711),#1764,.F.);
#24665=ADVANCED_FACE('',(#2712),#23973,.T.);
#24666=ADVANCED_FACE('',(#2713),#1765,.F.);
#24667=ADVANCED_FACE('',(#2714),#23974,.T.);
#24668=ADVANCED_FACE('',(#2715),#1766,.F.);
#24669=ADVANCED_FACE('',(#2716),#23975,.F.);
#24670=ADVANCED_FACE('',(#2717),#23976,.T.);
#24671=ADVANCED_FACE('',(#2718),#23977,.F.);
#24672=ADVANCED_FACE('',(#2719),#1767,.F.);
#24673=ADVANCED_FACE('',(#2720),#23978,.F.);
#24674=ADVANCED_FACE('',(#2721),#1768,.F.);
#24675=ADVANCED_FACE('',(#2722),#23979,.F.);
#24676=ADVANCED_FACE('',(#2723),#1769,.F.);
#24677=ADVANCED_FACE('',(#2724),#23980,.F.);
#24678=ADVANCED_FACE('',(#2725),#23981,.T.);
#24679=ADVANCED_FACE('',(#2726),#23982,.F.);
#24680=ADVANCED_FACE('',(#2727),#1770,.F.);
#24681=ADVANCED_FACE('',(#2728),#1771,.F.);
#24682=ADVANCED_FACE('',(#2729),#1772,.F.);
#24683=ADVANCED_FACE('',(#2730),#23983,.F.);
#24684=ADVANCED_FACE('',(#2731),#23984,.T.);
#24685=ADVANCED_FACE('',(#2732),#23985,.F.);
#24686=ADVANCED_FACE('',(#2733),#1773,.F.);
#24687=ADVANCED_FACE('',(#2734),#23986,.F.);
#24688=ADVANCED_FACE('',(#2735),#1774,.F.);
#24689=ADVANCED_FACE('',(#2736),#23987,.F.);
#24690=ADVANCED_FACE('',(#2737),#1775,.F.);
#24691=ADVANCED_FACE('',(#2738),#23988,.F.);
#24692=ADVANCED_FACE('',(#2739),#23989,.T.);
#24693=ADVANCED_FACE('',(#2740),#23990,.F.);
#24694=ADVANCED_FACE('',(#2741),#1776,.F.);
#24695=ADVANCED_FACE('',(#2742),#23991,.T.);
#24696=ADVANCED_FACE('',(#2743),#1777,.F.);
#24697=ADVANCED_FACE('',(#2744),#23992,.T.);
#24698=ADVANCED_FACE('',(#2745),#1778,.F.);
#24699=ADVANCED_FACE('',(#2746,#1285),#1779,.T.);
#24700=ADVANCED_FACE('',(#2747),#1780,.T.);
#24701=ADVANCED_FACE('',(#2748),#1781,.F.);
#24702=ADVANCED_FACE('',(#2749),#1782,.F.);
#24703=ADVANCED_FACE('',(#2750,#1286),#1783,.F.);
#24704=ADVANCED_FACE('',(#2751,#1287),#1784,.F.);
#24705=ADVANCED_FACE('',(#2752),#1785,.F.);
#24706=ADVANCED_FACE('',(#2753),#1786,.F.);
#24707=ADVANCED_FACE('',(#2754),#1787,.T.);
#24708=ADVANCED_FACE('',(#2755),#1788,.T.);
#24709=ADVANCED_FACE('',(#2756),#1789,.T.);
#24710=ADVANCED_FACE('',(#2757,#1288,#1289),#1790,.T.);
#24711=ADVANCED_FACE('',(#2758),#1791,.F.);
#24712=ADVANCED_FACE('',(#2759),#1792,.F.);
#24713=ADVANCED_FACE('',(#2760),#1793,.F.);
#24714=ADVANCED_FACE('',(#2761),#1794,.T.);
#24715=ADVANCED_FACE('',(#2762),#1795,.F.);
#24716=ADVANCED_FACE('',(#2763),#1796,.F.);
#24717=ADVANCED_FACE('',(#2764),#1797,.F.);
#24718=ADVANCED_FACE('',(#2765,#1290,#1291),#1798,.T.);
#24719=ADVANCED_FACE('',(#2766),#1799,.T.);
#24720=ADVANCED_FACE('',(#2767),#1800,.T.);
#24721=ADVANCED_FACE('',(#2768),#1801,.T.);
#24722=ADVANCED_FACE('',(#2769),#1802,.T.);
#24723=ADVANCED_FACE('',(#2770,#1292),#1803,.F.);
#24724=ADVANCED_FACE('',(#2771),#1804,.F.);
#24725=ADVANCED_FACE('',(#2772),#1805,.T.);
#24726=ADVANCED_FACE('',(#2773),#1806,.T.);
#24727=ADVANCED_FACE('',(#2774),#1807,.F.);
#24728=ADVANCED_FACE('',(#2775,#1293),#1808,.F.);
#24729=ADVANCED_FACE('',(#2776),#1809,.T.);
#24730=ADVANCED_FACE('',(#2777),#1810,.F.);
#24731=ADVANCED_FACE('',(#2778),#1811,.F.);
#24732=ADVANCED_FACE('',(#2779),#1812,.T.);
#24733=ADVANCED_FACE('',(#2780),#1813,.T.);
#24734=ADVANCED_FACE('',(#2781,#1294),#1814,.F.);
#24735=ADVANCED_FACE('',(#2782),#1815,.T.);
#24736=ADVANCED_FACE('',(#2783),#1816,.T.);
#24737=ADVANCED_FACE('',(#2784),#1817,.F.);
#24738=ADVANCED_FACE('',(#2785,#1295),#1818,.F.);
#24739=ADVANCED_FACE('',(#2786),#1819,.F.);
#24740=ADVANCED_FACE('',(#2787),#1820,.F.);
#24741=ADVANCED_FACE('',(#2788),#23993,.T.);
#24742=ADVANCED_FACE('',(#2789),#23994,.T.);
#24743=ADVANCED_FACE('',(#2790),#1821,.T.);
#24744=ADVANCED_FACE('',(#2791),#1822,.T.);
#24745=ADVANCED_FACE('',(#2792),#1823,.T.);
#24746=ADVANCED_FACE('',(#2793),#23995,.F.);
#24747=ADVANCED_FACE('',(#2794),#23996,.F.);
#24748=ADVANCED_FACE('',(#2795),#23997,.T.);
#24749=ADVANCED_FACE('',(#2796),#23998,.F.);
#24750=ADVANCED_FACE('',(#2797),#23999,.F.);
#24751=ADVANCED_FACE('',(#2798),#1824,.T.);
#24752=ADVANCED_FACE('',(#2799),#1825,.T.);
#24753=ADVANCED_FACE('',(#2800),#24000,.F.);
#24754=ADVANCED_FACE('',(#2801),#24001,.F.);
#24755=ADVANCED_FACE('',(#2802),#24002,.T.);
#24756=ADVANCED_FACE('',(#2803),#1826,.T.);
#24757=ADVANCED_FACE('',(#2804),#1827,.T.);
#24758=ADVANCED_FACE('',(#2805),#24003,.F.);
#24759=ADVANCED_FACE('',(#2806),#24004,.F.);
#24760=ADVANCED_FACE('',(#2807),#24005,.T.);
#24761=ADVANCED_FACE('',(#2808),#24006,.F.);
#24762=ADVANCED_FACE('',(#2809),#24007,.F.);
#24763=ADVANCED_FACE('',(#2810),#1828,.T.);
#24764=ADVANCED_FACE('',(#2811),#1829,.T.);
#24765=ADVANCED_FACE('',(#2812),#1830,.T.);
#24766=ADVANCED_FACE('',(#2813),#24008,.F.);
#24767=ADVANCED_FACE('',(#2814),#24009,.F.);
#24768=ADVANCED_FACE('',(#2815),#24010,.T.);
#24769=ADVANCED_FACE('',(#2816),#24011,.T.);
#24770=ADVANCED_FACE('',(#2817),#24012,.T.);
#24771=ADVANCED_FACE('',(#2818),#1831,.F.);
#24772=ADVANCED_FACE('',(#2819,#1296),#1832,.F.);
#24773=ADVANCED_FACE('',(#2820),#1833,.F.);
#24774=ADVANCED_FACE('',(#2821),#1834,.F.);
#24775=ADVANCED_FACE('',(#2822),#1835,.T.);
#24776=ADVANCED_FACE('',(#2823),#1836,.T.);
#24777=ADVANCED_FACE('',(#2824),#1837,.T.);
#24778=ADVANCED_FACE('',(#2825),#1838,.T.);
#24779=ADVANCED_FACE('',(#2826),#1839,.T.);
#24780=ADVANCED_FACE('',(#2827),#1840,.T.);
#24781=ADVANCED_FACE('',(#2828),#1841,.T.);
#24782=ADVANCED_FACE('',(#2829),#1842,.T.);
#24783=ADVANCED_FACE('',(#2830,#1297),#1843,.T.);
#24784=ADVANCED_FACE('',(#2831,#1298),#1844,.F.);
#24785=ADVANCED_FACE('',(#2832),#1845,.F.);
#24786=ADVANCED_FACE('',(#2833),#24013,.F.);
#24787=ADVANCED_FACE('',(#2834),#1846,.F.);
#24788=ADVANCED_FACE('',(#2835),#1847,.T.);
#24789=ADVANCED_FACE('',(#2836),#24014,.F.);
#24790=ADVANCED_FACE('',(#2837),#24015,.F.);
#24791=ADVANCED_FACE('',(#2838),#24016,.F.);
#24792=ADVANCED_FACE('',(#2839),#24017,.F.);
#25671=CLOSED_SHELL('',(#24454,#24455,#24456,#24457,#24458,#24459,#24460,
#24461,#24462,#24463,#24464,#24465,#24466,#24467,#24468,#24469,#24470,#24471,
#24472,#24473,#24474,#24475,#24476,#24477,#24478,#24479,#24480,#24481,#24482,
#24483,#24484,#24485,#24486,#24487,#24488,#24489,#24490,#24491,#24492,#24493,
#24494,#24495,#24496,#24497,#24498,#24499,#24500,#24501,#24502,#24503,#24504,
#24505,#24506,#24507,#24508,#24509,#24510,#24511,#24512,#24513,#24514,#24515,
#24516,#24517,#24518,#24519,#24520,#24521,#24522,#24523,#24524,#24525,#24526,
#24527,#24528,#24529,#24530,#24531,#24532,#24533,#24534,#24535,#24536,#24537,
#24538,#24539,#24540,#24541,#24542,#24543,#24544,#24545,#24546,#24547,#24548,
#24549,#24550,#24551,#24552,#24553,#24554,#24555,#24556,#24557,#24558,#24559,
#24560,#24561,#24562,#24563,#24564,#24565,#24566,#24567,#24568,#24569,#24570,
#24571,#24572,#24573,#24574,#24575,#24576,#24577,#24578,#24579,#24580,#24581,
#24582,#24583,#24584,#24585,#24586,#24587,#24588,#24589,#24590,#24591,#24592,
#24593,#24594,#24595,#24596,#24597,#24598,#24599,#24600,#24601,#24602,#24603,
#24604,#24605,#24606,#24607,#24608,#24609,#24610,#24611,#24612,#24613,#24614,
#24615,#24616,#24617,#24618,#24619,#24620,#24621,#24622,#24623,#24624,#24625,
#24626,#24627,#24628,#24629,#24630,#24631,#24632,#24633,#24634,#24635,#24636,
#24637,#24638,#24639,#24640,#24641,#24642,#24643,#24644,#24645,#24646,#24647,
#24648,#24649,#24650,#24651,#24652,#24653,#24654,#24655,#24656,#24657,#24658,
#24659,#24660,#24661,#24662,#24663,#24664,#24665,#24666,#24667,#24668,#24669,
#24670,#24671,#24672,#24673,#24674,#24675,#24676,#24677,#24678,#24679,#24680,
#24681,#24682,#24683,#24684,#24685,#24686,#24687,#24688,#24689,#24690,#24691,
#24692,#24693,#24694,#24695,#24696,#24697,#24698,#24699,#24700,#24701,#24702,
#24703,#24704,#24705,#24706,#24707,#24708,#24709,#24710,#24711,#24712,#24713,
#24714,#24715,#24716,#24717,#24718,#24719,#24720,#24721,#24722,#24723,#24724,
#24725,#24726,#24727,#24728,#24729,#24730,#24731,#24732,#24733,#24734,#24735,
#24736,#24737,#24738,#24739,#24740,#24741,#24742,#24743,#24744,#24745,#24746,
#24747,#24748,#24749,#24750,#24751,#24752,#24753,#24754,#24755,#24756,#24757,
#24758,#24759,#24760,#24761,#24762,#24763,#24764,#24765,#24766,#24767,#24768,
#24769,#24770,#24771,#24772,#24773,#24774,#24775,#24776,#24777,#24778,#24779,
#24780,#24781,#24782,#24783,#24784,#24785,#24786,#24787,#24788,#24789,#24790,
#24791,#24792));
#26592=AXIS2_PLACEMENT_3D('',#37495,#30197,#30198);
#26593=AXIS2_PLACEMENT_3D('',#37496,#30199,#30200);
#26594=AXIS2_PLACEMENT_3D('',#37498,#30201,#30202);
#26595=AXIS2_PLACEMENT_3D('',#37501,#30204,#30205);
#26596=AXIS2_PLACEMENT_3D('',#37502,#30206,#30207);
#26597=AXIS2_PLACEMENT_3D('',#37504,#30208,#30209);
#26598=AXIS2_PLACEMENT_3D('',#37507,#30211,#30212);
#26599=AXIS2_PLACEMENT_3D('',#37508,#30213,#30214);
#26600=AXIS2_PLACEMENT_3D('',#37510,#30215,#30216);
#26601=AXIS2_PLACEMENT_3D('',#37513,#30218,#30219);
#26602=AXIS2_PLACEMENT_3D('',#37514,#30220,#30221);
#26603=AXIS2_PLACEMENT_3D('',#37517,#30223,#30224);
#26604=AXIS2_PLACEMENT_3D('',#37520,#30226,#30227);
#26605=AXIS2_PLACEMENT_3D('',#37522,#30228,#30229);
#26606=AXIS2_PLACEMENT_3D('',#37525,#30231,#30232);
#26607=AXIS2_PLACEMENT_3D('',#37526,#30233,#30234);
#26608=AXIS2_PLACEMENT_3D('',#37528,#30235,#30236);
#26609=AXIS2_PLACEMENT_3D('',#37531,#30238,#30239);
#26610=AXIS2_PLACEMENT_3D('',#37532,#30240,#30241);
#26611=AXIS2_PLACEMENT_3D('',#37534,#30242,#30243);
#26612=AXIS2_PLACEMENT_3D('',#37537,#30245,#30246);
#26613=AXIS2_PLACEMENT_3D('',#37538,#30247,#30248);
#26614=AXIS2_PLACEMENT_3D('',#37540,#30249,#30250);
#26615=AXIS2_PLACEMENT_3D('',#37543,#30252,#30253);
#26616=AXIS2_PLACEMENT_3D('',#37544,#30254,#30255);
#26617=AXIS2_PLACEMENT_3D('',#37546,#30256,#30257);
#26618=AXIS2_PLACEMENT_3D('',#37549,#30259,#30260);
#26619=AXIS2_PLACEMENT_3D('',#37550,#30261,#30262);
#26620=AXIS2_PLACEMENT_3D('',#37552,#30263,#30264);
#26621=AXIS2_PLACEMENT_3D('',#37555,#30266,#30267);
#26622=AXIS2_PLACEMENT_3D('',#37556,#30268,#30269);
#26623=AXIS2_PLACEMENT_3D('',#37558,#30270,#30271);
#26624=AXIS2_PLACEMENT_3D('',#37561,#30273,#30274);
#26625=AXIS2_PLACEMENT_3D('',#37562,#30275,#30276);
#26626=AXIS2_PLACEMENT_3D('',#37564,#30277,#30278);
#26627=AXIS2_PLACEMENT_3D('',#37568,#30280,#30281);
#26628=AXIS2_PLACEMENT_3D('',#37572,#30283,#30284);
#26629=AXIS2_PLACEMENT_3D('',#37574,#30286,#30287);
#26630=AXIS2_PLACEMENT_3D('',#37577,#30289,#30290);
#26631=AXIS2_PLACEMENT_3D('',#37580,#30292,#30293);
#26632=AXIS2_PLACEMENT_3D('',#37582,#30294,#30295);
#26633=AXIS2_PLACEMENT_3D('',#37588,#30298,#30299);
#26634=AXIS2_PLACEMENT_3D('',#37591,#30301,#30302);
#26635=AXIS2_PLACEMENT_3D('',#37658,#30303,#30304);
#26636=AXIS2_PLACEMENT_3D('',#37659,#30305,#30306);
#26637=AXIS2_PLACEMENT_3D('',#37692,#30307,#30308);
#26638=AXIS2_PLACEMENT_3D('',#37694,#30309,#30310);
#26639=AXIS2_PLACEMENT_3D('',#37696,#30312,#30313);
#26640=AXIS2_PLACEMENT_3D('',#37698,#30314,#30315);
#26641=AXIS2_PLACEMENT_3D('',#37701,#30317,#30318);
#26642=AXIS2_PLACEMENT_3D('',#37702,#30319,#30320);
#26643=AXIS2_PLACEMENT_3D('',#37705,#30321,#30322);
#26644=AXIS2_PLACEMENT_3D('',#37711,#30326,#30327);
#26645=AXIS2_PLACEMENT_3D('',#37713,#30328,#30329);
#26646=AXIS2_PLACEMENT_3D('',#37717,#30331,#30332);
#26647=AXIS2_PLACEMENT_3D('',#37719,#30334,#30335);
#26648=AXIS2_PLACEMENT_3D('',#37722,#30336,#30337);
#26649=AXIS2_PLACEMENT_3D('',#37726,#30339,#30340);
#26650=AXIS2_PLACEMENT_3D('',#37728,#30342,#30343);
#26651=AXIS2_PLACEMENT_3D('',#37730,#30344,#30345);
#26652=AXIS2_PLACEMENT_3D('',#37736,#30349,#30350);
#26653=AXIS2_PLACEMENT_3D('',#37745,#30355,#30356);
#26654=AXIS2_PLACEMENT_3D('',#37754,#30361,#30362);
#26655=AXIS2_PLACEMENT_3D('',#37763,#30367,#30368);
#26656=AXIS2_PLACEMENT_3D('',#37772,#30373,#30374);
#26657=AXIS2_PLACEMENT_3D('',#37781,#30379,#30380);
#26658=AXIS2_PLACEMENT_3D('',#37790,#30385,#30386);
#26659=AXIS2_PLACEMENT_3D('',#37799,#30391,#30392);
#26660=AXIS2_PLACEMENT_3D('',#37808,#30397,#30398);
#26661=AXIS2_PLACEMENT_3D('',#37817,#30403,#30404);
#26662=AXIS2_PLACEMENT_3D('',#37823,#30408,#30409);
#26663=AXIS2_PLACEMENT_3D('',#37832,#30414,#30415);
#26664=AXIS2_PLACEMENT_3D('',#37838,#30419,#30420);
#26665=AXIS2_PLACEMENT_3D('',#37847,#30425,#30426);
#26666=AXIS2_PLACEMENT_3D('',#37856,#30431,#30432);
#26667=AXIS2_PLACEMENT_3D('',#37865,#30437,#30438);
#26668=AXIS2_PLACEMENT_3D('',#37874,#30443,#30444);
#26669=AXIS2_PLACEMENT_3D('',#37877,#30447,#30448);
#26670=AXIS2_PLACEMENT_3D('',#37880,#30449,#30450);
#26671=AXIS2_PLACEMENT_3D('',#37884,#30452,#30453);
#26672=AXIS2_PLACEMENT_3D('',#37886,#30455,#30456);
#26673=AXIS2_PLACEMENT_3D('',#37889,#30457,#30458);
#26674=AXIS2_PLACEMENT_3D('',#37893,#30460,#30461);
#26675=AXIS2_PLACEMENT_3D('',#37895,#30463,#30464);
#26676=AXIS2_PLACEMENT_3D('',#37898,#30465,#30466);
#26677=AXIS2_PLACEMENT_3D('',#37902,#30468,#30469);
#26678=AXIS2_PLACEMENT_3D('',#37904,#30471,#30472);
#26679=AXIS2_PLACEMENT_3D('',#37907,#30473,#30474);
#26680=AXIS2_PLACEMENT_3D('',#37911,#30476,#30477);
#26681=AXIS2_PLACEMENT_3D('',#37913,#30479,#30480);
#26682=AXIS2_PLACEMENT_3D('',#37914,#30481,#30482);
#26683=AXIS2_PLACEMENT_3D('',#37915,#30483,#30484);
#26684=AXIS2_PLACEMENT_3D('',#37916,#30485,#30486);
#26685=AXIS2_PLACEMENT_3D('',#37917,#30487,#30488);
#26686=AXIS2_PLACEMENT_3D('',#37918,#30489,#30490);
#26687=AXIS2_PLACEMENT_3D('',#37919,#30491,#30492);
#26688=AXIS2_PLACEMENT_3D('',#37920,#30493,#30494);
#26689=AXIS2_PLACEMENT_3D('',#37921,#30495,#30496);
#26690=AXIS2_PLACEMENT_3D('',#37922,#30497,#30498);
#26691=AXIS2_PLACEMENT_3D('',#37923,#30499,#30500);
#26692=AXIS2_PLACEMENT_3D('',#37924,#30501,#30502);
#26693=AXIS2_PLACEMENT_3D('',#37925,#30503,#30504);
#26694=AXIS2_PLACEMENT_3D('',#37926,#30505,#30506);
#26695=AXIS2_PLACEMENT_3D('',#37927,#30507,#30508);
#26696=AXIS2_PLACEMENT_3D('',#37928,#30509,#30510);
#26697=AXIS2_PLACEMENT_3D('',#37929,#30511,#30512);
#26698=AXIS2_PLACEMENT_3D('',#37930,#30513,#30514);
#26699=AXIS2_PLACEMENT_3D('',#37931,#30515,#30516);
#26700=AXIS2_PLACEMENT_3D('',#37932,#30517,#30518);
#26701=AXIS2_PLACEMENT_3D('',#37933,#30519,#30520);
#26702=AXIS2_PLACEMENT_3D('',#37934,#30521,#30522);
#26703=AXIS2_PLACEMENT_3D('',#37935,#30523,#30524);
#26704=AXIS2_PLACEMENT_3D('',#37936,#30525,#30526);
#26705=AXIS2_PLACEMENT_3D('',#37937,#30527,#30528);
#26706=AXIS2_PLACEMENT_3D('',#37938,#30529,#30530);
#26707=AXIS2_PLACEMENT_3D('',#37939,#30531,#30532);
#26708=AXIS2_PLACEMENT_3D('',#37940,#30533,#30534);
#26709=AXIS2_PLACEMENT_3D('',#37941,#30535,#30536);
#26710=AXIS2_PLACEMENT_3D('',#37942,#30537,#30538);
#26711=AXIS2_PLACEMENT_3D('',#37943,#30539,#30540);
#26712=AXIS2_PLACEMENT_3D('',#37944,#30541,#30542);
#26713=AXIS2_PLACEMENT_3D('',#37945,#30543,#30544);
#26714=AXIS2_PLACEMENT_3D('',#37946,#30545,#30546);
#26715=AXIS2_PLACEMENT_3D('',#37947,#30547,#30548);
#26716=AXIS2_PLACEMENT_3D('',#37948,#30549,#30550);
#26717=AXIS2_PLACEMENT_3D('',#37949,#30551,#30552);
#26718=AXIS2_PLACEMENT_3D('',#37950,#30553,#30554);
#26719=AXIS2_PLACEMENT_3D('',#37951,#30555,#30556);
#26720=AXIS2_PLACEMENT_3D('',#37952,#30557,#30558);
#26721=AXIS2_PLACEMENT_3D('',#37953,#30559,#30560);
#26722=AXIS2_PLACEMENT_3D('',#37954,#30561,#30562);
#26723=AXIS2_PLACEMENT_3D('',#37955,#30563,#30564);
#26724=AXIS2_PLACEMENT_3D('',#37956,#30565,#30566);
#26725=AXIS2_PLACEMENT_3D('',#37957,#30567,#30568);
#26726=AXIS2_PLACEMENT_3D('',#37958,#30569,#30570);
#26727=AXIS2_PLACEMENT_3D('',#37959,#30571,#30572);
#26728=AXIS2_PLACEMENT_3D('',#37960,#30573,#30574);
#26729=AXIS2_PLACEMENT_3D('',#37961,#30575,#30576);
#26730=AXIS2_PLACEMENT_3D('',#37962,#30577,#30578);
#26731=AXIS2_PLACEMENT_3D('',#37971,#30583,#30584);
#26732=AXIS2_PLACEMENT_3D('',#37982,#30591,#30592);
#26733=AXIS2_PLACEMENT_3D('',#37986,#30595,#30596);
#26734=AXIS2_PLACEMENT_3D('',#37990,#30599,#30600);
#26735=AXIS2_PLACEMENT_3D('',#37992,#30602,#30603);
#26736=AXIS2_PLACEMENT_3D('',#37996,#30606,#30607);
#26737=AXIS2_PLACEMENT_3D('',#38000,#30610,#30611);
#26738=AXIS2_PLACEMENT_3D('',#38002,#30613,#30614);
#26739=AXIS2_PLACEMENT_3D('',#38008,#30618,#30619);
#26740=AXIS2_PLACEMENT_3D('',#38012,#30622,#30623);
#26741=AXIS2_PLACEMENT_3D('',#38016,#30626,#30627);
#26742=AXIS2_PLACEMENT_3D('',#38020,#30630,#30631);
#26743=AXIS2_PLACEMENT_3D('',#38024,#30634,#30635);
#26744=AXIS2_PLACEMENT_3D('',#38026,#30637,#30638);
#26745=AXIS2_PLACEMENT_3D('',#38027,#30639,#30640);
#26746=AXIS2_PLACEMENT_3D('',#38032,#30642,#30643);
#26747=AXIS2_PLACEMENT_3D('',#38036,#30645,#30646);
#26748=AXIS2_PLACEMENT_3D('',#38040,#30648,#30649);
#26749=AXIS2_PLACEMENT_3D('',#38042,#30650,#30651);
#26750=AXIS2_PLACEMENT_3D('',#38044,#30652,#30653);
#26751=AXIS2_PLACEMENT_3D('',#38048,#30655,#30656);
#26752=AXIS2_PLACEMENT_3D('',#38052,#30658,#30659);
#26753=AXIS2_PLACEMENT_3D('',#38056,#30661,#30662);
#26754=AXIS2_PLACEMENT_3D('',#38058,#30663,#30664);
#26755=AXIS2_PLACEMENT_3D('',#38060,#30665,#30666);
#26756=AXIS2_PLACEMENT_3D('',#38068,#30670,#30671);
#26757=AXIS2_PLACEMENT_3D('',#38070,#30672,#30673);
#26758=AXIS2_PLACEMENT_3D('',#38072,#30674,#30675);
#26759=AXIS2_PLACEMENT_3D('',#38076,#30677,#30678);
#26760=AXIS2_PLACEMENT_3D('',#38080,#30680,#30681);
#26761=AXIS2_PLACEMENT_3D('',#38084,#30683,#30684);
#26762=AXIS2_PLACEMENT_3D('',#38086,#30685,#30686);
#26763=AXIS2_PLACEMENT_3D('',#38088,#30687,#30688);
#26764=AXIS2_PLACEMENT_3D('',#38092,#30690,#30691);
#26765=AXIS2_PLACEMENT_3D('',#38096,#30693,#30694);
#26766=AXIS2_PLACEMENT_3D('',#38116,#30705,#30706);
#26767=AXIS2_PLACEMENT_3D('',#38122,#30710,#30711);
#26768=AXIS2_PLACEMENT_3D('',#38124,#30712,#30713);
#26769=AXIS2_PLACEMENT_3D('',#38126,#30715,#30716);
#26770=AXIS2_PLACEMENT_3D('',#38130,#30719,#30720);
#26771=AXIS2_PLACEMENT_3D('',#38132,#30721,#30722);
#26772=AXIS2_PLACEMENT_3D('',#38134,#30724,#30725);
#26773=AXIS2_PLACEMENT_3D('',#38138,#30728,#30729);
#26774=AXIS2_PLACEMENT_3D('',#38140,#30730,#30731);
#26775=AXIS2_PLACEMENT_3D('',#38142,#30733,#30734);
#26776=AXIS2_PLACEMENT_3D('',#38144,#30735,#30736);
#26777=AXIS2_PLACEMENT_3D('',#38146,#30738,#30739);
#26778=AXIS2_PLACEMENT_3D('',#38148,#30740,#30741);
#26779=AXIS2_PLACEMENT_3D('',#38150,#30743,#30744);
#26780=AXIS2_PLACEMENT_3D('',#38154,#30747,#30748);
#26781=AXIS2_PLACEMENT_3D('',#38156,#30749,#30750);
#26782=AXIS2_PLACEMENT_3D('',#38158,#30752,#30753);
#26783=AXIS2_PLACEMENT_3D('',#38162,#30756,#30757);
#26784=AXIS2_PLACEMENT_3D('',#38164,#30758,#30759);
#26785=AXIS2_PLACEMENT_3D('',#38166,#30761,#30762);
#26786=AXIS2_PLACEMENT_3D('',#38170,#30765,#30766);
#26787=AXIS2_PLACEMENT_3D('',#38172,#30767,#30768);
#26788=AXIS2_PLACEMENT_3D('',#38174,#30770,#30771);
#26789=AXIS2_PLACEMENT_3D('',#38176,#30772,#30773);
#26790=AXIS2_PLACEMENT_3D('',#38178,#30775,#30776);
#26791=AXIS2_PLACEMENT_3D('',#38180,#30777,#30778);
#26792=AXIS2_PLACEMENT_3D('',#38182,#30780,#30781);
#26793=AXIS2_PLACEMENT_3D('',#38186,#30784,#30785);
#26794=AXIS2_PLACEMENT_3D('',#38190,#30788,#30789);
#26795=AXIS2_PLACEMENT_3D('',#38194,#30792,#30793);
#26796=AXIS2_PLACEMENT_3D('',#38196,#30794,#30795);
#26797=AXIS2_PLACEMENT_3D('',#38198,#30797,#30798);
#26798=AXIS2_PLACEMENT_3D('',#38200,#30799,#30800);
#26799=AXIS2_PLACEMENT_3D('',#38202,#30802,#30803);
#26800=AXIS2_PLACEMENT_3D('',#38204,#30804,#30805);
#26801=AXIS2_PLACEMENT_3D('',#38206,#30807,#30808);
#26802=AXIS2_PLACEMENT_3D('',#38210,#30811,#30812);
#26803=AXIS2_PLACEMENT_3D('',#38212,#30813,#30814);
#26804=AXIS2_PLACEMENT_3D('',#38214,#30816,#30817);
#26805=AXIS2_PLACEMENT_3D('',#38218,#30820,#30821);
#26806=AXIS2_PLACEMENT_3D('',#38220,#30822,#30823);
#26807=AXIS2_PLACEMENT_3D('',#38222,#30825,#30826);
#26808=AXIS2_PLACEMENT_3D('',#38226,#30829,#30830);
#26809=AXIS2_PLACEMENT_3D('',#38228,#30831,#30832);
#26810=AXIS2_PLACEMENT_3D('',#38230,#30834,#30835);
#26811=AXIS2_PLACEMENT_3D('',#38232,#30836,#30837);
#26812=AXIS2_PLACEMENT_3D('',#38234,#30839,#30840);
#26813=AXIS2_PLACEMENT_3D('',#38236,#30841,#30842);
#26814=AXIS2_PLACEMENT_3D('',#38238,#30844,#30845);
#26815=AXIS2_PLACEMENT_3D('',#38242,#30848,#30849);
#26816=AXIS2_PLACEMENT_3D('',#38244,#30850,#30851);
#26817=AXIS2_PLACEMENT_3D('',#38246,#30853,#30854);
#26818=AXIS2_PLACEMENT_3D('',#38250,#30857,#30858);
#26819=AXIS2_PLACEMENT_3D('',#38252,#30859,#30860);
#26820=AXIS2_PLACEMENT_3D('',#38254,#30862,#30863);
#26821=AXIS2_PLACEMENT_3D('',#38258,#30866,#30867);
#26822=AXIS2_PLACEMENT_3D('',#38262,#30870,#30871);
#26823=AXIS2_PLACEMENT_3D('',#38266,#30874,#30875);
#26824=AXIS2_PLACEMENT_3D('',#38270,#30878,#30879);
#26825=AXIS2_PLACEMENT_3D('',#38274,#30882,#30883);
#26826=AXIS2_PLACEMENT_3D('',#38278,#30886,#30887);
#26827=AXIS2_PLACEMENT_3D('',#38282,#30890,#30891);
#26828=AXIS2_PLACEMENT_3D('',#38286,#30894,#30895);
#26829=AXIS2_PLACEMENT_3D('',#38290,#30898,#30899);
#26830=AXIS2_PLACEMENT_3D('',#38292,#30901,#30902);
#26831=AXIS2_PLACEMENT_3D('',#38293,#30903,#30904);
#26832=AXIS2_PLACEMENT_3D('',#38297,#30906,#30907);
#26833=AXIS2_PLACEMENT_3D('',#38299,#30909,#30910);
#26834=AXIS2_PLACEMENT_3D('',#38306,#30913,#30914);
#26835=AXIS2_PLACEMENT_3D('',#38322,#30922,#30923);
#26836=AXIS2_PLACEMENT_3D('',#38326,#30925,#30926);
#26837=AXIS2_PLACEMENT_3D('',#38330,#30928,#30929);
#26838=AXIS2_PLACEMENT_3D('',#38332,#30930,#30931);
#26839=AXIS2_PLACEMENT_3D('',#38334,#30932,#30933);
#26840=AXIS2_PLACEMENT_3D('',#38338,#30935,#30936);
#26841=AXIS2_PLACEMENT_3D('',#38342,#30938,#30939);
#26842=AXIS2_PLACEMENT_3D('',#38346,#30941,#30942);
#26843=AXIS2_PLACEMENT_3D('',#38348,#30943,#30944);
#26844=AXIS2_PLACEMENT_3D('',#38350,#30945,#30946);
#26845=AXIS2_PLACEMENT_3D('',#38358,#30950,#30951);
#26846=AXIS2_PLACEMENT_3D('',#38360,#30952,#30953);
#26847=AXIS2_PLACEMENT_3D('',#38362,#30954,#30955);
#26848=AXIS2_PLACEMENT_3D('',#38366,#30957,#30958);
#26849=AXIS2_PLACEMENT_3D('',#38370,#30960,#30961);
#26850=AXIS2_PLACEMENT_3D('',#38374,#30963,#30964);
#26851=AXIS2_PLACEMENT_3D('',#38376,#30965,#30966);
#26852=AXIS2_PLACEMENT_3D('',#38378,#30967,#30968);
#26853=AXIS2_PLACEMENT_3D('',#38382,#30970,#30971);
#26854=AXIS2_PLACEMENT_3D('',#38386,#30973,#30974);
#26855=AXIS2_PLACEMENT_3D('',#38396,#30980,#30981);
#26856=AXIS2_PLACEMENT_3D('',#38400,#30984,#30985);
#26857=AXIS2_PLACEMENT_3D('',#38404,#30988,#30989);
#26858=AXIS2_PLACEMENT_3D('',#38405,#30990,#30991);
#26859=AXIS2_PLACEMENT_3D('',#38406,#30992,#30993);
#26860=AXIS2_PLACEMENT_3D('',#38407,#30994,#30995);
#26861=AXIS2_PLACEMENT_3D('',#38411,#30997,#30998);
#26862=AXIS2_PLACEMENT_3D('',#38413,#31000,#31001);
#26863=AXIS2_PLACEMENT_3D('',#38419,#31005,#31006);
#26864=AXIS2_PLACEMENT_3D('',#38423,#31009,#31010);
#26865=AXIS2_PLACEMENT_3D('',#38427,#31013,#31014);
#26866=AXIS2_PLACEMENT_3D('',#38431,#31017,#31018);
#26867=AXIS2_PLACEMENT_3D('',#38440,#31024,#31025);
#26868=AXIS2_PLACEMENT_3D('',#38444,#31028,#31029);
#26869=AXIS2_PLACEMENT_3D('',#38448,#31032,#31033);
#26870=AXIS2_PLACEMENT_3D('',#38452,#31036,#31037);
#26871=AXIS2_PLACEMENT_3D('',#38456,#31040,#31041);
#26872=AXIS2_PLACEMENT_3D('',#38460,#31044,#31045);
#26873=AXIS2_PLACEMENT_3D('',#38462,#31046,#31047);
#26874=AXIS2_PLACEMENT_3D('',#38464,#31049,#31050);
#26875=AXIS2_PLACEMENT_3D('',#38468,#31053,#31054);
#26876=AXIS2_PLACEMENT_3D('',#38470,#31055,#31056);
#26877=AXIS2_PLACEMENT_3D('',#38472,#31058,#31059);
#26878=AXIS2_PLACEMENT_3D('',#38476,#31062,#31063);
#26879=AXIS2_PLACEMENT_3D('',#38478,#31064,#31065);
#26880=AXIS2_PLACEMENT_3D('',#38480,#31067,#31068);
#26881=AXIS2_PLACEMENT_3D('',#38482,#31069,#31070);
#26882=AXIS2_PLACEMENT_3D('',#38484,#31072,#31073);
#26883=AXIS2_PLACEMENT_3D('',#38486,#31074,#31075);
#26884=AXIS2_PLACEMENT_3D('',#38488,#31077,#31078);
#26885=AXIS2_PLACEMENT_3D('',#38492,#31081,#31082);
#26886=AXIS2_PLACEMENT_3D('',#38494,#31083,#31084);
#26887=AXIS2_PLACEMENT_3D('',#38496,#31086,#31087);
#26888=AXIS2_PLACEMENT_3D('',#38500,#31090,#31091);
#26889=AXIS2_PLACEMENT_3D('',#38502,#31092,#31093);
#26890=AXIS2_PLACEMENT_3D('',#38504,#31095,#31096);
#26891=AXIS2_PLACEMENT_3D('',#38508,#31099,#31100);
#26892=AXIS2_PLACEMENT_3D('',#38510,#31101,#31102);
#26893=AXIS2_PLACEMENT_3D('',#38512,#31104,#31105);
#26894=AXIS2_PLACEMENT_3D('',#38514,#31106,#31107);
#26895=AXIS2_PLACEMENT_3D('',#38516,#31109,#31110);
#26896=AXIS2_PLACEMENT_3D('',#38518,#31111,#31112);
#26897=AXIS2_PLACEMENT_3D('',#38520,#31114,#31115);
#26898=AXIS2_PLACEMENT_3D('',#38524,#31118,#31119);
#26899=AXIS2_PLACEMENT_3D('',#38528,#31122,#31123);
#26900=AXIS2_PLACEMENT_3D('',#38532,#31126,#31127);
#26901=AXIS2_PLACEMENT_3D('',#38534,#31128,#31129);
#26902=AXIS2_PLACEMENT_3D('',#38536,#31131,#31132);
#26903=AXIS2_PLACEMENT_3D('',#38538,#31133,#31134);
#26904=AXIS2_PLACEMENT_3D('',#38540,#31136,#31137);
#26905=AXIS2_PLACEMENT_3D('',#38542,#31138,#31139);
#26906=AXIS2_PLACEMENT_3D('',#38544,#31141,#31142);
#26907=AXIS2_PLACEMENT_3D('',#38548,#31145,#31146);
#26908=AXIS2_PLACEMENT_3D('',#38550,#31147,#31148);
#26909=AXIS2_PLACEMENT_3D('',#38552,#31150,#31151);
#26910=AXIS2_PLACEMENT_3D('',#38556,#31154,#31155);
#26911=AXIS2_PLACEMENT_3D('',#38558,#31156,#31157);
#26912=AXIS2_PLACEMENT_3D('',#38560,#31159,#31160);
#26913=AXIS2_PLACEMENT_3D('',#38564,#31163,#31164);
#26914=AXIS2_PLACEMENT_3D('',#38566,#31165,#31166);
#26915=AXIS2_PLACEMENT_3D('',#38568,#31168,#31169);
#26916=AXIS2_PLACEMENT_3D('',#38570,#31170,#31171);
#26917=AXIS2_PLACEMENT_3D('',#38572,#31173,#31174);
#26918=AXIS2_PLACEMENT_3D('',#38574,#31175,#31176);
#26919=AXIS2_PLACEMENT_3D('',#38576,#31178,#31179);
#26920=AXIS2_PLACEMENT_3D('',#38580,#31182,#31183);
#26921=AXIS2_PLACEMENT_3D('',#38582,#31184,#31185);
#26922=AXIS2_PLACEMENT_3D('',#38584,#31187,#31188);
#26923=AXIS2_PLACEMENT_3D('',#38588,#31191,#31192);
#26924=AXIS2_PLACEMENT_3D('',#38590,#31193,#31194);
#26925=AXIS2_PLACEMENT_3D('',#38592,#31196,#31197);
#26926=AXIS2_PLACEMENT_3D('',#38594,#31199,#31200);
#26927=AXIS2_PLACEMENT_3D('',#38595,#31201,#31202);
#26928=AXIS2_PLACEMENT_3D('',#38604,#31207,#31208);
#26929=AXIS2_PLACEMENT_3D('',#38613,#31213,#31214);
#26930=AXIS2_PLACEMENT_3D('',#38617,#31217,#31218);
#26931=AXIS2_PLACEMENT_3D('',#38621,#31221,#31222);
#26932=AXIS2_PLACEMENT_3D('',#38622,#31223,#31224);
#26933=AXIS2_PLACEMENT_3D('',#38623,#31225,#31226);
#26934=AXIS2_PLACEMENT_3D('',#38625,#31227,#31228);
#26935=AXIS2_PLACEMENT_3D('',#38627,#31229,#31230);
#26936=AXIS2_PLACEMENT_3D('',#38629,#31232,#31233);
#26937=AXIS2_PLACEMENT_3D('',#38637,#31238,#31239);
#26938=AXIS2_PLACEMENT_3D('',#38643,#31243,#31244);
#26939=AXIS2_PLACEMENT_3D('',#38652,#31249,#31250);
#26940=AXIS2_PLACEMENT_3D('',#38655,#31252,#31253);
#26941=AXIS2_PLACEMENT_3D('',#38659,#31256,#31257);
#26942=AXIS2_PLACEMENT_3D('',#38662,#31259,#31260);
#26943=AXIS2_PLACEMENT_3D('',#38663,#31261,#31262);
#26944=AXIS2_PLACEMENT_3D('',#38686,#31273,#31274);
#26945=AXIS2_PLACEMENT_3D('',#38690,#31276,#31277);
#26946=AXIS2_PLACEMENT_3D('',#38694,#31279,#31280);
#26947=AXIS2_PLACEMENT_3D('',#38696,#31281,#31282);
#26948=AXIS2_PLACEMENT_3D('',#38698,#31283,#31284);
#26949=AXIS2_PLACEMENT_3D('',#38702,#31286,#31287);
#26950=AXIS2_PLACEMENT_3D('',#38706,#31289,#31290);
#26951=AXIS2_PLACEMENT_3D('',#38710,#31292,#31293);
#26952=AXIS2_PLACEMENT_3D('',#38712,#31294,#31295);
#26953=AXIS2_PLACEMENT_3D('',#38714,#31296,#31297);
#26954=AXIS2_PLACEMENT_3D('',#38722,#31301,#31302);
#26955=AXIS2_PLACEMENT_3D('',#38724,#31303,#31304);
#26956=AXIS2_PLACEMENT_3D('',#38726,#31305,#31306);
#26957=AXIS2_PLACEMENT_3D('',#38730,#31308,#31309);
#26958=AXIS2_PLACEMENT_3D('',#38734,#31311,#31312);
#26959=AXIS2_PLACEMENT_3D('',#38738,#31314,#31315);
#26960=AXIS2_PLACEMENT_3D('',#38740,#31316,#31317);
#26961=AXIS2_PLACEMENT_3D('',#38742,#31318,#31319);
#26962=AXIS2_PLACEMENT_3D('',#38746,#31321,#31322);
#26963=AXIS2_PLACEMENT_3D('',#38750,#31324,#31325);
#26964=AXIS2_PLACEMENT_3D('',#38752,#31327,#31328);
#26965=AXIS2_PLACEMENT_3D('',#38756,#31331,#31332);
#26966=AXIS2_PLACEMENT_3D('',#38760,#31335,#31336);
#26967=AXIS2_PLACEMENT_3D('',#38766,#31340,#31341);
#26968=AXIS2_PLACEMENT_3D('',#38772,#31345,#31346);
#26969=AXIS2_PLACEMENT_3D('',#38778,#31350,#31351);
#26970=AXIS2_PLACEMENT_3D('',#38784,#31355,#31356);
#26971=AXIS2_PLACEMENT_3D('',#38785,#31357,#31358);
#26972=AXIS2_PLACEMENT_3D('',#38786,#31359,#31360);
#26973=AXIS2_PLACEMENT_3D('',#38787,#31361,#31362);
#26974=AXIS2_PLACEMENT_3D('',#38788,#31363,#31364);
#26975=AXIS2_PLACEMENT_3D('',#38790,#31365,#31366);
#26976=AXIS2_PLACEMENT_3D('',#38796,#31370,#31371);
#26977=AXIS2_PLACEMENT_3D('',#38802,#31375,#31376);
#26978=AXIS2_PLACEMENT_3D('',#38804,#31377,#31378);
#26979=AXIS2_PLACEMENT_3D('',#38808,#31381,#31382);
#26980=AXIS2_PLACEMENT_3D('',#38814,#31386,#31387);
#26981=AXIS2_PLACEMENT_3D('',#38818,#31390,#31391);
#26982=AXIS2_PLACEMENT_3D('',#38819,#31392,#31393);
#26983=AXIS2_PLACEMENT_3D('',#38821,#31394,#31395);
#26984=AXIS2_PLACEMENT_3D('',#38825,#31398,#31399);
#26985=AXIS2_PLACEMENT_3D('',#38826,#31400,#31401);
#26986=AXIS2_PLACEMENT_3D('',#38827,#31402,#31403);
#26987=AXIS2_PLACEMENT_3D('',#38828,#31404,#31405);
#26988=AXIS2_PLACEMENT_3D('',#38834,#31409,#31410);
#26989=AXIS2_PLACEMENT_3D('',#38838,#31413,#31414);
#26990=AXIS2_PLACEMENT_3D('',#38842,#31417,#31418);
#26991=AXIS2_PLACEMENT_3D('',#38846,#31421,#31422);
#26992=AXIS2_PLACEMENT_3D('',#38850,#31425,#31426);
#26993=AXIS2_PLACEMENT_3D('',#38854,#31429,#31430);
#26994=AXIS2_PLACEMENT_3D('',#38858,#31433,#31434);
#26995=AXIS2_PLACEMENT_3D('',#38862,#31437,#31438);
#26996=AXIS2_PLACEMENT_3D('',#38866,#31441,#31442);
#26997=AXIS2_PLACEMENT_3D('',#38870,#31445,#31446);
#26998=AXIS2_PLACEMENT_3D('',#38872,#31447,#31448);
#26999=AXIS2_PLACEMENT_3D('',#38874,#31450,#31451);
#27000=AXIS2_PLACEMENT_3D('',#38878,#31454,#31455);
#27001=AXIS2_PLACEMENT_3D('',#38880,#31456,#31457);
#27002=AXIS2_PLACEMENT_3D('',#38882,#31459,#31460);
#27003=AXIS2_PLACEMENT_3D('',#38886,#31463,#31464);
#27004=AXIS2_PLACEMENT_3D('',#38888,#31465,#31466);
#27005=AXIS2_PLACEMENT_3D('',#38890,#31468,#31469);
#27006=AXIS2_PLACEMENT_3D('',#38892,#31470,#31471);
#27007=AXIS2_PLACEMENT_3D('',#38894,#31473,#31474);
#27008=AXIS2_PLACEMENT_3D('',#38896,#31475,#31476);
#27009=AXIS2_PLACEMENT_3D('',#38898,#31478,#31479);
#27010=AXIS2_PLACEMENT_3D('',#38902,#31482,#31483);
#27011=AXIS2_PLACEMENT_3D('',#38904,#31484,#31485);
#27012=AXIS2_PLACEMENT_3D('',#38906,#31487,#31488);
#27013=AXIS2_PLACEMENT_3D('',#38910,#31491,#31492);
#27014=AXIS2_PLACEMENT_3D('',#38912,#31493,#31494);
#27015=AXIS2_PLACEMENT_3D('',#38914,#31496,#31497);
#27016=AXIS2_PLACEMENT_3D('',#38918,#31500,#31501);
#27017=AXIS2_PLACEMENT_3D('',#38920,#31502,#31503);
#27018=AXIS2_PLACEMENT_3D('',#38922,#31505,#31506);
#27019=AXIS2_PLACEMENT_3D('',#38924,#31507,#31508);
#27020=AXIS2_PLACEMENT_3D('',#38926,#31510,#31511);
#27021=AXIS2_PLACEMENT_3D('',#38928,#31512,#31513);
#27022=AXIS2_PLACEMENT_3D('',#38930,#31515,#31516);
#27023=AXIS2_PLACEMENT_3D('',#38934,#31519,#31520);
#27024=AXIS2_PLACEMENT_3D('',#38938,#31523,#31524);
#27025=AXIS2_PLACEMENT_3D('',#38942,#31527,#31528);
#27026=AXIS2_PLACEMENT_3D('',#38944,#31529,#31530);
#27027=AXIS2_PLACEMENT_3D('',#38946,#31532,#31533);
#27028=AXIS2_PLACEMENT_3D('',#38948,#31534,#31535);
#27029=AXIS2_PLACEMENT_3D('',#38950,#31537,#31538);
#27030=AXIS2_PLACEMENT_3D('',#38952,#31539,#31540);
#27031=AXIS2_PLACEMENT_3D('',#38954,#31542,#31543);
#27032=AXIS2_PLACEMENT_3D('',#38958,#31546,#31547);
#27033=AXIS2_PLACEMENT_3D('',#38960,#31548,#31549);
#27034=AXIS2_PLACEMENT_3D('',#38962,#31551,#31552);
#27035=AXIS2_PLACEMENT_3D('',#38966,#31555,#31556);
#27036=AXIS2_PLACEMENT_3D('',#38968,#31557,#31558);
#27037=AXIS2_PLACEMENT_3D('',#38970,#31560,#31561);
#27038=AXIS2_PLACEMENT_3D('',#38974,#31564,#31565);
#27039=AXIS2_PLACEMENT_3D('',#38976,#31566,#31567);
#27040=AXIS2_PLACEMENT_3D('',#38978,#31569,#31570);
#27041=AXIS2_PLACEMENT_3D('',#38980,#31571,#31572);
#27042=AXIS2_PLACEMENT_3D('',#38982,#31574,#31575);
#27043=AXIS2_PLACEMENT_3D('',#38984,#31576,#31577);
#27044=AXIS2_PLACEMENT_3D('',#38986,#31579,#31580);
#27045=AXIS2_PLACEMENT_3D('',#38990,#31583,#31584);
#27046=AXIS2_PLACEMENT_3D('',#38992,#31585,#31586);
#27047=AXIS2_PLACEMENT_3D('',#38994,#31588,#31589);
#27048=AXIS2_PLACEMENT_3D('',#38998,#31592,#31593);
#27049=AXIS2_PLACEMENT_3D('',#39000,#31594,#31595);
#27050=AXIS2_PLACEMENT_3D('',#39002,#31597,#31598);
#27051=AXIS2_PLACEMENT_3D('',#39004,#31600,#31601);
#27052=AXIS2_PLACEMENT_3D('',#39013,#31606,#31607);
#27053=AXIS2_PLACEMENT_3D('',#39019,#31611,#31612);
#27054=AXIS2_PLACEMENT_3D('',#39025,#31616,#31617);
#27055=AXIS2_PLACEMENT_3D('',#39031,#31621,#31622);
#27056=AXIS2_PLACEMENT_3D('',#39037,#31626,#31627);
#27057=AXIS2_PLACEMENT_3D('',#39046,#31632,#31633);
#27058=AXIS2_PLACEMENT_3D('',#39052,#31637,#31638);
#27059=AXIS2_PLACEMENT_3D('',#39058,#31642,#31643);
#27060=AXIS2_PLACEMENT_3D('',#39061,#31646,#31647);
#27061=AXIS2_PLACEMENT_3D('',#39069,#31652,#31653);
#27062=AXIS2_PLACEMENT_3D('',#39075,#31657,#31658);
#27063=AXIS2_PLACEMENT_3D('',#39081,#31662,#31663);
#27064=AXIS2_PLACEMENT_3D('',#39087,#31667,#31668);
#27065=AXIS2_PLACEMENT_3D('',#39093,#31672,#31673);
#27066=AXIS2_PLACEMENT_3D('',#39099,#31677,#31678);
#27067=AXIS2_PLACEMENT_3D('',#39105,#31682,#31683);
#27068=AXIS2_PLACEMENT_3D('',#39111,#31687,#31688);
#27069=AXIS2_PLACEMENT_3D('',#39117,#31692,#31693);
#27070=AXIS2_PLACEMENT_3D('',#39123,#31697,#31698);
#27071=AXIS2_PLACEMENT_3D('',#39129,#31702,#31703);
#27072=AXIS2_PLACEMENT_3D('',#39135,#31707,#31708);
#27073=AXIS2_PLACEMENT_3D('',#39141,#31712,#31713);
#27074=AXIS2_PLACEMENT_3D('',#39147,#31717,#31718);
#27075=AXIS2_PLACEMENT_3D('',#39152,#31722,#31723);
#27076=AXIS2_PLACEMENT_3D('',#39154,#31724,#31725);
#27077=AXIS2_PLACEMENT_3D('',#39158,#31728,#31729);
#27078=AXIS2_PLACEMENT_3D('',#39164,#31733,#31734);
#27079=AXIS2_PLACEMENT_3D('',#39166,#31735,#31736);
#27080=AXIS2_PLACEMENT_3D('',#39170,#31739,#31740);
#27081=AXIS2_PLACEMENT_3D('',#39172,#31741,#31742);
#27082=AXIS2_PLACEMENT_3D('',#39176,#31745,#31746);
#27083=AXIS2_PLACEMENT_3D('',#39182,#31750,#31751);
#27084=AXIS2_PLACEMENT_3D('',#39184,#31753,#31754);
#27085=AXIS2_PLACEMENT_3D('',#39185,#31755,#31756);
#27086=AXIS2_PLACEMENT_3D('',#39186,#31757,#31758);
#27087=AXIS2_PLACEMENT_3D('',#39190,#31761,#31762);
#27088=AXIS2_PLACEMENT_3D('',#39196,#31766,#31767);
#27089=AXIS2_PLACEMENT_3D('',#39202,#31771,#31772);
#27090=AXIS2_PLACEMENT_3D('',#39207,#31776,#31777);
#27091=AXIS2_PLACEMENT_3D('',#39208,#31778,#31779);
#27092=AXIS2_PLACEMENT_3D('',#39210,#31781,#31782);
#27093=AXIS2_PLACEMENT_3D('',#39216,#31785,#31786);
#27094=AXIS2_PLACEMENT_3D('',#39220,#31788,#31789);
#27095=AXIS2_PLACEMENT_3D('',#39224,#31791,#31792);
#27096=AXIS2_PLACEMENT_3D('',#39226,#31793,#31794);
#27097=AXIS2_PLACEMENT_3D('',#39228,#31795,#31796);
#27098=AXIS2_PLACEMENT_3D('',#39232,#31798,#31799);
#27099=AXIS2_PLACEMENT_3D('',#39236,#31801,#31802);
#27100=AXIS2_PLACEMENT_3D('',#39240,#31804,#31805);
#27101=AXIS2_PLACEMENT_3D('',#39242,#31806,#31807);
#27102=AXIS2_PLACEMENT_3D('',#39244,#31808,#31809);
#27103=AXIS2_PLACEMENT_3D('',#39252,#31813,#31814);
#27104=AXIS2_PLACEMENT_3D('',#39254,#31815,#31816);
#27105=AXIS2_PLACEMENT_3D('',#39256,#31817,#31818);
#27106=AXIS2_PLACEMENT_3D('',#39260,#31820,#31821);
#27107=AXIS2_PLACEMENT_3D('',#39264,#31823,#31824);
#27108=AXIS2_PLACEMENT_3D('',#39268,#31826,#31827);
#27109=AXIS2_PLACEMENT_3D('',#39270,#31828,#31829);
#27110=AXIS2_PLACEMENT_3D('',#39272,#31830,#31831);
#27111=AXIS2_PLACEMENT_3D('',#39276,#31833,#31834);
#27112=AXIS2_PLACEMENT_3D('',#39280,#31836,#31837);
#27113=AXIS2_PLACEMENT_3D('',#39284,#31840,#31841);
#27114=AXIS2_PLACEMENT_3D('',#39310,#31855,#31856);
#27115=AXIS2_PLACEMENT_3D('',#39316,#31860,#31861);
#27116=AXIS2_PLACEMENT_3D('',#39322,#31865,#31866);
#27117=AXIS2_PLACEMENT_3D('',#39326,#31869,#31870);
#27118=AXIS2_PLACEMENT_3D('',#39330,#31873,#31874);
#27119=AXIS2_PLACEMENT_3D('',#39334,#31877,#31878);
#27120=AXIS2_PLACEMENT_3D('',#39338,#31880,#31881);
#27121=AXIS2_PLACEMENT_3D('',#39340,#31883,#31884);
#27122=AXIS2_PLACEMENT_3D('',#39344,#31886,#31887);
#27123=AXIS2_PLACEMENT_3D('',#39346,#31889,#31890);
#27124=AXIS2_PLACEMENT_3D('',#39348,#31892,#31893);
#27125=AXIS2_PLACEMENT_3D('',#39352,#31896,#31897);
#27126=AXIS2_PLACEMENT_3D('',#39354,#31899,#31900);
#27127=AXIS2_PLACEMENT_3D('',#39357,#31901,#31902);
#27128=AXIS2_PLACEMENT_3D('',#39360,#31905,#31906);
#27129=AXIS2_PLACEMENT_3D('',#39363,#31907,#31908);
#27130=AXIS2_PLACEMENT_3D('',#39366,#31911,#31912);
#27131=AXIS2_PLACEMENT_3D('',#39367,#31913,#31914);
#27132=AXIS2_PLACEMENT_3D('',#39368,#31915,#31916);
#27133=AXIS2_PLACEMENT_3D('',#39371,#31917,#31918);
#27134=AXIS2_PLACEMENT_3D('',#39374,#31921,#31922);
#27135=AXIS2_PLACEMENT_3D('',#39377,#31923,#31924);
#27136=AXIS2_PLACEMENT_3D('',#39380,#31927,#31928);
#27137=AXIS2_PLACEMENT_3D('',#39382,#31930,#31931);
#27138=AXIS2_PLACEMENT_3D('',#39384,#31933,#31934);
#27139=AXIS2_PLACEMENT_3D('',#39387,#31935,#31936);
#27140=AXIS2_PLACEMENT_3D('',#39390,#31939,#31940);
#27141=AXIS2_PLACEMENT_3D('',#39393,#31941,#31942);
#27142=AXIS2_PLACEMENT_3D('',#39396,#31945,#31946);
#27143=AXIS2_PLACEMENT_3D('',#39397,#31947,#31948);
#27144=AXIS2_PLACEMENT_3D('',#39398,#31949,#31950);
#27145=AXIS2_PLACEMENT_3D('',#39404,#31954,#31955);
#27146=AXIS2_PLACEMENT_3D('',#39406,#31957,#31958);
#27147=AXIS2_PLACEMENT_3D('',#39409,#31959,#31960);
#27148=AXIS2_PLACEMENT_3D('',#39412,#31963,#31964);
#27149=AXIS2_PLACEMENT_3D('',#39415,#31965,#31966);
#27150=AXIS2_PLACEMENT_3D('',#39418,#31969,#31970);
#27151=AXIS2_PLACEMENT_3D('',#39419,#31971,#31972);
#27152=AXIS2_PLACEMENT_3D('',#39420,#31973,#31974);
#27153=AXIS2_PLACEMENT_3D('',#39423,#31975,#31976);
#27154=AXIS2_PLACEMENT_3D('',#39426,#31979,#31980);
#27155=AXIS2_PLACEMENT_3D('',#39429,#31981,#31982);
#27156=AXIS2_PLACEMENT_3D('',#39432,#31985,#31986);
#27157=AXIS2_PLACEMENT_3D('',#39434,#31988,#31989);
#27158=AXIS2_PLACEMENT_3D('',#39436,#31991,#31992);
#27159=AXIS2_PLACEMENT_3D('',#39438,#31994,#31995);
#27160=AXIS2_PLACEMENT_3D('',#39441,#31996,#31997);
#27161=AXIS2_PLACEMENT_3D('',#39444,#32000,#32001);
#27162=AXIS2_PLACEMENT_3D('',#39447,#32002,#32003);
#27163=AXIS2_PLACEMENT_3D('',#39450,#32006,#32007);
#27164=AXIS2_PLACEMENT_3D('',#39451,#32008,#32009);
#27165=AXIS2_PLACEMENT_3D('',#39452,#32010,#32011);
#27166=AXIS2_PLACEMENT_3D('',#39456,#32013,#32014);
#27167=AXIS2_PLACEMENT_3D('',#39458,#32016,#32017);
#27168=AXIS2_PLACEMENT_3D('',#39462,#32019,#32020);
#27169=AXIS2_PLACEMENT_3D('',#39464,#32022,#32023);
#27170=AXIS2_PLACEMENT_3D('',#39470,#32027,#32028);
#27171=AXIS2_PLACEMENT_3D('',#39474,#32031,#32032);
#27172=AXIS2_PLACEMENT_3D('',#39478,#32035,#32036);
#27173=AXIS2_PLACEMENT_3D('',#39480,#32038,#32039);
#27174=AXIS2_PLACEMENT_3D('',#39484,#32042,#32043);
#27175=AXIS2_PLACEMENT_3D('',#39486,#32045,#32046);
#27176=AXIS2_PLACEMENT_3D('',#39488,#32048,#32049);
#27177=AXIS2_PLACEMENT_3D('',#39490,#32051,#32052);
#27178=AXIS2_PLACEMENT_3D('',#39492,#32054,#32055);
#27179=AXIS2_PLACEMENT_3D('',#39494,#32057,#32058);
#27180=AXIS2_PLACEMENT_3D('',#39496,#32060,#32061);
#27181=AXIS2_PLACEMENT_3D('',#39500,#32064,#32065);
#27182=AXIS2_PLACEMENT_3D('',#39502,#32067,#32068);
#27183=AXIS2_PLACEMENT_3D('',#39503,#32069,#32070);
#27184=AXIS2_PLACEMENT_3D('',#39507,#32073,#32074);
#27185=AXIS2_PLACEMENT_3D('',#39509,#32075,#32076);
#27186=AXIS2_PLACEMENT_3D('',#39511,#32078,#32079);
#27187=AXIS2_PLACEMENT_3D('',#39513,#32081,#32082);
#27188=AXIS2_PLACEMENT_3D('',#39514,#32083,#32084);
#27189=AXIS2_PLACEMENT_3D('',#39515,#32085,#32086);
#27190=AXIS2_PLACEMENT_3D('',#39516,#32087,#32088);
#27191=AXIS2_PLACEMENT_3D('',#39517,#32089,#32090);
#30197=DIRECTION('axis',(0.,0.,1.));
#30198=DIRECTION('refdir',(1.,0.,0.));
#30199=DIRECTION('center_axis',(1.,0.,0.));
#30200=DIRECTION('ref_axis',(0.,0.,-1.));
#30201=DIRECTION('center_axis',(1.,0.,0.));
#30202=DIRECTION('ref_axis',(0.,0.,-1.));
#30203=DIRECTION('',(1.,0.,0.));
#30204=DIRECTION('center_axis',(1.,0.,0.));
#30205=DIRECTION('ref_axis',(0.,0.,-1.));
#30206=DIRECTION('center_axis',(-1.,0.,0.));
#30207=DIRECTION('ref_axis',(0.,0.,1.));
#30208=DIRECTION('center_axis',(-1.,0.,0.));
#30209=DIRECTION('ref_axis',(0.,0.,1.));
#30210=DIRECTION('',(-1.,0.,0.));
#30211=DIRECTION('center_axis',(-1.,0.,0.));
#30212=DIRECTION('ref_axis',(0.,0.,1.));
#30213=DIRECTION('center_axis',(-1.30104260698261E-15,1.,-1.73611473352215E-31));
#30214=DIRECTION('ref_axis',(-1.,-1.30104260698261E-15,-2.16593351677506E-47));
#30215=DIRECTION('center_axis',(-1.30104260698261E-15,1.,-1.73611473352215E-31));
#30216=DIRECTION('ref_axis',(-1.,-1.30104260698261E-15,-2.16593351677507E-47));
#30217=DIRECTION('',(-1.30104260698261E-15,1.,-1.73611473352215E-31));
#30218=DIRECTION('center_axis',(-1.30104260698261E-15,1.,-1.73611473352215E-31));
#30219=DIRECTION('ref_axis',(-1.,-1.30104260698261E-15,-2.16593351677507E-47));
#30220=DIRECTION('center_axis',(1.,0.,0.));
#30221=DIRECTION('ref_axis',(0.,0.,-1.));
#30222=DIRECTION('',(0.515038074910055,-1.04972719113862E-16,0.857167300702112));
#30223=DIRECTION('center_axis',(-1.,0.,0.));
#30224=DIRECTION('ref_axis',(0.,0.,1.));
#30225=DIRECTION('',(-0.515038074910054,-1.04972719113862E-16,-0.857167300702112));
#30226=DIRECTION('center_axis',(0.,1.,0.));
#30227=DIRECTION('ref_axis',(0.,0.,1.));
#30228=DIRECTION('center_axis',(-1.2823896663807E-16,1.,0.));
#30229=DIRECTION('ref_axis',(-1.,-1.2823896663807E-16,0.));
#30230=DIRECTION('',(0.,1.,0.));
#30231=DIRECTION('center_axis',(0.,1.,0.));
#30232=DIRECTION('ref_axis',(0.,0.,1.));
#30233=DIRECTION('center_axis',(0.,1.,0.));
#30234=DIRECTION('ref_axis',(0.,0.,1.));
#30235=DIRECTION('center_axis',(-1.2823896663807E-16,1.,0.));
#30236=DIRECTION('ref_axis',(-1.,-1.2823896663807E-16,0.));
#30237=DIRECTION('',(0.,1.,0.));
#30238=DIRECTION('center_axis',(0.,1.,0.));
#30239=DIRECTION('ref_axis',(0.,0.,1.));
#30240=DIRECTION('center_axis',(0.,1.,0.));
#30241=DIRECTION('ref_axis',(0.,0.,1.));
#30242=DIRECTION('center_axis',(1.2823896663807E-16,1.,0.));
#30243=DIRECTION('ref_axis',(-1.,1.2823896663807E-16,0.));
#30244=DIRECTION('',(0.,1.,0.));
#30245=DIRECTION('center_axis',(0.,1.,0.));
#30246=DIRECTION('ref_axis',(0.,0.,1.));
#30247=DIRECTION('center_axis',(0.,1.,0.));
#30248=DIRECTION('ref_axis',(0.,0.,1.));
#30249=DIRECTION('center_axis',(1.2823896663807E-16,1.,0.));
#30250=DIRECTION('ref_axis',(-1.,1.2823896663807E-16,0.));
#30251=DIRECTION('',(0.,1.,0.));
#30252=DIRECTION('center_axis',(0.,1.,0.));
#30253=DIRECTION('ref_axis',(0.,0.,1.));
#30254=DIRECTION('center_axis',(-1.,0.,0.));
#30255=DIRECTION('ref_axis',(0.,0.,1.));
#30256=DIRECTION('center_axis',(-1.,0.,0.));
#30257=DIRECTION('ref_axis',(0.,0.,1.));
#30258=DIRECTION('',(-1.,0.,0.));
#30259=DIRECTION('center_axis',(-1.,0.,0.));
#30260=DIRECTION('ref_axis',(0.,0.,1.));
#30261=DIRECTION('center_axis',(1.,0.,0.));
#30262=DIRECTION('ref_axis',(0.,0.,-1.));
#30263=DIRECTION('center_axis',(1.,0.,0.));
#30264=DIRECTION('ref_axis',(0.,0.,-1.));
#30265=DIRECTION('',(1.,0.,0.));
#30266=DIRECTION('center_axis',(1.,0.,0.));
#30267=DIRECTION('ref_axis',(0.,0.,-1.));
#30268=DIRECTION('center_axis',(-1.30104260698261E-15,1.,-1.73611473352215E-31));
#30269=DIRECTION('ref_axis',(-1.,-1.30104260698261E-15,-2.16593351677506E-47));
#30270=DIRECTION('center_axis',(-1.30104260698261E-15,1.,-1.73611473352215E-31));
#30271=DIRECTION('ref_axis',(-1.,-1.30104260698261E-15,-2.16593351677507E-47));
#30272=DIRECTION('',(-1.30104260698261E-15,1.,-1.73611473352215E-31));
#30273=DIRECTION('center_axis',(-1.30104260698261E-15,1.,-1.73611473352215E-31));
#30274=DIRECTION('ref_axis',(-1.,-1.30104260698261E-15,-2.16593351677507E-47));
#30275=DIRECTION('center_axis',(-1.30104260698261E-15,1.,-1.73611473352215E-31));
#30276=DIRECTION('ref_axis',(-1.,-1.30104260698261E-15,2.25875923892257E-46));
#30277=DIRECTION('center_axis',(-1.30104260698261E-15,1.,-1.73611473352215E-31));
#30278=DIRECTION('ref_axis',(-1.,-1.30104260698261E-15,2.25875923892257E-46));
#30279=DIRECTION('',(-1.30104260698261E-15,1.,-1.73611473352215E-31));
#30280=DIRECTION('center_axis',(-1.30104260698261E-15,1.,-1.73611473352215E-31));
#30281=DIRECTION('ref_axis',(-1.,-1.30104260698261E-15,2.25875923892257E-46));
#30282=DIRECTION('',(-1.30104260698261E-15,1.,-1.73611473352215E-31));
#30283=DIRECTION('center_axis',(-1.30104260698261E-15,1.,-1.73611473352215E-31));
#30284=DIRECTION('ref_axis',(-1.,-1.30104260698261E-15,2.25875923892257E-46));
#30285=DIRECTION('',(-1.30104260698261E-15,1.,-1.73611473352215E-31));
#30286=DIRECTION('center_axis',(-1.,0.,0.));
#30287=DIRECTION('ref_axis',(0.,0.,1.));
#30288=DIRECTION('',(-0.515038074910054,-1.04972719113862E-16,-0.857167300702112));
#30289=DIRECTION('center_axis',(1.,0.,0.));
#30290=DIRECTION('ref_axis',(0.,0.,-1.));
#30291=DIRECTION('',(0.515038074910055,-1.04972719113862E-16,0.857167300702112));
#30292=DIRECTION('center_axis',(-1.30104260698261E-15,1.,-1.73611473352215E-31));
#30293=DIRECTION('ref_axis',(-1.,-1.30104260698261E-15,2.25875923892257E-46));
#30294=DIRECTION('center_axis',(-1.30104260698261E-15,1.,-1.73611473352215E-31));
#30295=DIRECTION('ref_axis',(-1.,-1.30104260698261E-15,2.25875923892257E-46));
#30296=DIRECTION('',(-1.30104260698261E-15,1.,-1.73611473352215E-31));
#30297=DIRECTION('',(-1.30104260698261E-15,1.,-1.73611473352215E-31));
#30298=DIRECTION('center_axis',(-1.30104260698261E-15,1.,-1.73611473352215E-31));
#30299=DIRECTION('ref_axis',(-1.,-1.30104260698261E-15,2.25875923892257E-46));
#30300=DIRECTION('',(-1.30104260698261E-15,1.,-1.73611473352215E-31));
#30301=DIRECTION('center_axis',(-1.30104260698261E-15,1.,-1.73611473352215E-31));
#30302=DIRECTION('ref_axis',(-1.,-1.30104260698261E-15,2.25875923892257E-46));
#30303=DIRECTION('center_axis',(0.,0.,1.));
#30304=DIRECTION('ref_axis',(-1.,0.,0.));
#30305=DIRECTION('center_axis',(0.,0.,1.));
#30306=DIRECTION('ref_axis',(-1.,0.,0.));
#30307=DIRECTION('center_axis',(0.,0.,1.));
#30308=DIRECTION('ref_axis',(1.,0.,0.));
#30309=DIRECTION('center_axis',(0.,0.,-1.));
#30310=DIRECTION('ref_axis',(-1.,0.,0.));
#30311=DIRECTION('',(0.,0.,-1.));
#30312=DIRECTION('center_axis',(0.,0.,-1.));
#30313=DIRECTION('ref_axis',(-1.,0.,0.));
#30314=DIRECTION('center_axis',(0.,0.,-1.));
#30315=DIRECTION('ref_axis',(-1.,0.,0.));
#30316=DIRECTION('',(0.,0.,-1.));
#30317=DIRECTION('center_axis',(0.,0.,-1.));
#30318=DIRECTION('ref_axis',(-1.,0.,0.));
#30319=DIRECTION('center_axis',(0.61566147532566,-0.788010753606721,0.));
#30320=DIRECTION('ref_axis',(0.78801075360672,0.61566147532566,0.));
#30321=DIRECTION('center_axis',(0.615661475325656,-0.788010753606724,-5.22755357805913E-15));
#30322=DIRECTION('ref_axis',(0.788010753606724,0.615661475325656,-5.17730530723809E-13));
#30323=DIRECTION('',(0.,0.,1.));
#30324=DIRECTION('',(0.78801075360672,0.61566147532566,0.));
#30325=DIRECTION('',(0.,0.,1.));
#30326=DIRECTION('center_axis',(0.61566147532566,-0.788010753606721,0.));
#30327=DIRECTION('ref_axis',(0.78801075360672,0.61566147532566,0.));
#30328=DIRECTION('center_axis',(0.615661475325656,-0.788010753606724,5.27148259972344E-15));
#30329=DIRECTION('ref_axis',(0.788010753606724,0.615661475325656,-9.16833363821094E-14));
#30330=DIRECTION('',(0.,0.,1.));
#30331=DIRECTION('center_axis',(0.615661475325662,-0.788010753606719,1.40572869325959E-15));
#30332=DIRECTION('ref_axis',(0.788010753606719,0.615661475325662,-7.1472163446861E-13));
#30333=DIRECTION('',(0.,0.,1.));
#30334=DIRECTION('center_axis',(-0.61566147532566,-0.788010753606721,0.));
#30335=DIRECTION('ref_axis',(0.78801075360672,-0.61566147532566,0.));
#30336=DIRECTION('center_axis',(-0.615661475325663,-0.788010753606718,-3.73396684147081E-15));
#30337=DIRECTION('ref_axis',(0.788010753606718,-0.615661475325663,1.05496270744081E-13));
#30338=DIRECTION('',(0.,0.,1.));
#30339=DIRECTION('center_axis',(-0.615661475325666,-0.788010753606716,6.32577911966821E-15));
#30340=DIRECTION('ref_axis',(0.788010753606716,-0.615661475325666,2.12834187078208E-13));
#30341=DIRECTION('',(0.,0.,1.));
#30342=DIRECTION('center_axis',(-0.61566147532566,-0.788010753606721,0.));
#30343=DIRECTION('ref_axis',(0.78801075360672,-0.61566147532566,0.));
#30344=DIRECTION('center_axis',(-0.615661475325663,-0.788010753606718,-3.64610879814206E-15));
#30345=DIRECTION('ref_axis',(0.788010753606718,-0.615661475325663,-2.42930938978673E-14));
#30346=DIRECTION('',(0.,0.,1.));
#30347=DIRECTION('',(0.78801075360672,-0.61566147532566,0.));
#30348=DIRECTION('',(0.,0.,1.));
#30349=DIRECTION('center_axis',(-0.707106781186546,0.707106781186549,0.));
#30350=DIRECTION('ref_axis',(-0.707106781186549,-0.707106781186546,0.));
#30351=DIRECTION('',(-0.707106781186549,-0.707106781186546,0.));
#30352=DIRECTION('',(0.,0.,-1.));
#30353=DIRECTION('',(-0.707106781186549,-0.707106781186546,0.));
#30354=DIRECTION('',(0.,0.,1.));
#30355=DIRECTION('center_axis',(-0.707106781186549,-0.707106781186546,0.));
#30356=DIRECTION('ref_axis',(0.707106781186546,-0.707106781186549,0.));
#30357=DIRECTION('',(0.707106781186545,-0.70710678118655,0.));
#30358=DIRECTION('',(0.,0.,-1.));
#30359=DIRECTION('',(0.707106781186546,-0.707106781186549,0.));
#30360=DIRECTION('',(0.,0.,1.));
#30361=DIRECTION('center_axis',(0.707106781186546,0.707106781186549,0.));
#30362=DIRECTION('ref_axis',(-0.707106781186549,0.707106781186546,0.));
#30363=DIRECTION('',(-0.707106781186548,0.707106781186547,0.));
#30364=DIRECTION('',(0.,0.,-1.));
#30365=DIRECTION('',(-0.707106781186549,0.707106781186546,0.));
#30366=DIRECTION('',(0.,0.,1.));
#30367=DIRECTION('center_axis',(0.707106781186549,-0.707106781186546,0.));
#30368=DIRECTION('ref_axis',(0.707106781186546,0.707106781186549,0.));
#30369=DIRECTION('',(0.707106781186546,0.707106781186549,0.));
#30370=DIRECTION('',(0.,0.,-1.));
#30371=DIRECTION('',(0.707106781186546,0.707106781186549,0.));
#30372=DIRECTION('',(0.,0.,1.));
#30373=DIRECTION('center_axis',(0.707106781186549,-0.707106781186546,0.));
#30374=DIRECTION('ref_axis',(0.707106781186546,0.707106781186549,0.));
#30375=DIRECTION('',(0.707106781186545,0.70710678118655,0.));
#30376=DIRECTION('',(0.,0.,-1.));
#30377=DIRECTION('',(0.707106781186546,0.707106781186549,0.));
#30378=DIRECTION('',(0.,0.,1.));
#30379=DIRECTION('center_axis',(1.,0.,0.));
#30380=DIRECTION('ref_axis',(0.,0.,-1.));
#30381=DIRECTION('',(0.,1.,0.));
#30382=DIRECTION('',(0.,0.,-1.));
#30383=DIRECTION('',(0.,1.,0.));
#30384=DIRECTION('',(0.,0.,1.));
#30385=DIRECTION('center_axis',(0.707106781186546,0.707106781186549,0.));
#30386=DIRECTION('ref_axis',(-0.707106781186549,0.707106781186546,0.));
#30387=DIRECTION('',(-0.707106781186549,0.707106781186546,0.));
#30388=DIRECTION('',(0.,0.,-1.));
#30389=DIRECTION('',(-0.707106781186549,0.707106781186546,0.));
#30390=DIRECTION('',(0.,0.,1.));
#30391=DIRECTION('center_axis',(1.,0.,0.));
#30392=DIRECTION('ref_axis',(0.,0.,-1.));
#30393=DIRECTION('',(0.,1.,0.));
#30394=DIRECTION('',(0.,0.,-1.));
#30395=DIRECTION('',(0.,1.,0.));
#30396=DIRECTION('',(0.,0.,1.));
#30397=DIRECTION('center_axis',(0.707106781186549,-0.707106781186546,0.));
#30398=DIRECTION('ref_axis',(0.707106781186546,0.707106781186549,0.));
#30399=DIRECTION('',(0.707106781186546,0.707106781186549,0.));
#30400=DIRECTION('',(0.,0.,1.));
#30401=DIRECTION('',(0.707106781186546,0.707106781186549,0.));
#30402=DIRECTION('',(0.,0.,1.));
#30403=DIRECTION('center_axis',(0.,-1.,0.));
#30404=DIRECTION('ref_axis',(0.,0.,-1.));
#30405=DIRECTION('',(1.,0.,0.));
#30406=DIRECTION('',(0.,0.,1.));
#30407=DIRECTION('',(1.,0.,0.));
#30408=DIRECTION('center_axis',(-6.49101394191508E-16,-1.,0.));
#30409=DIRECTION('ref_axis',(1.,-6.49101394191508E-16,0.));
#30410=DIRECTION('',(1.,-3.50803534070133E-16,0.));
#30411=DIRECTION('',(0.,0.,1.));
#30412=DIRECTION('',(1.,-6.49101394191508E-16,0.));
#30413=DIRECTION('',(0.,0.,1.));
#30414=DIRECTION('center_axis',(-0.707106781186549,-0.707106781186546,0.));
#30415=DIRECTION('ref_axis',(0.707106781186546,-0.707106781186549,0.));
#30416=DIRECTION('',(0.707106781186546,-0.707106781186549,0.));
#30417=DIRECTION('',(0.,0.,-1.));
#30418=DIRECTION('',(0.707106781186546,-0.707106781186549,0.));
#30419=DIRECTION('center_axis',(-1.,0.,0.));
#30420=DIRECTION('ref_axis',(0.,0.,1.));
#30421=DIRECTION('',(0.,-1.,0.));
#30422=DIRECTION('',(0.,0.,-1.));
#30423=DIRECTION('',(0.,-1.,0.));
#30424=DIRECTION('',(0.,0.,1.));
#30425=DIRECTION('center_axis',(-0.707106781186546,0.707106781186549,0.));
#30426=DIRECTION('ref_axis',(-0.707106781186549,-0.707106781186546,0.));
#30427=DIRECTION('',(-0.707106781186548,-0.707106781186547,0.));
#30428=DIRECTION('',(0.,0.,-1.));
#30429=DIRECTION('',(-0.707106781186549,-0.707106781186546,0.));
#30430=DIRECTION('',(0.,0.,1.));
#30431=DIRECTION('center_axis',(-1.,0.,0.));
#30432=DIRECTION('ref_axis',(0.,0.,1.));
#30433=DIRECTION('',(0.,-1.,0.));
#30434=DIRECTION('',(0.,0.,-1.));
#30435=DIRECTION('',(0.,-1.,0.));
#30436=DIRECTION('',(0.,0.,1.));
#30437=DIRECTION('center_axis',(-0.707106781186549,-0.707106781186546,0.));
#30438=DIRECTION('ref_axis',(0.707106781186546,-0.707106781186549,0.));
#30439=DIRECTION('',(0.707106781186546,-0.707106781186549,0.));
#30440=DIRECTION('',(0.,0.,1.));
#30441=DIRECTION('',(0.707106781186546,-0.707106781186549,0.));
#30442=DIRECTION('',(0.,0.,1.));
#30443=DIRECTION('center_axis',(1.22464679914735E-16,-1.,0.));
#30444=DIRECTION('ref_axis',(1.,1.22464679914735E-16,0.));
#30445=DIRECTION('',(1.,1.22464679914735E-16,0.));
#30446=DIRECTION('',(1.,1.22464679914735E-16,0.));
#30447=DIRECTION('center_axis',(0.,0.,1.));
#30448=DIRECTION('ref_axis',(1.,0.,0.));
#30449=DIRECTION('center_axis',(0.,0.,1.));
#30450=DIRECTION('ref_axis',(1.,0.,0.));
#30451=DIRECTION('',(0.,0.,-1.));
#30452=DIRECTION('center_axis',(0.,0.,1.));
#30453=DIRECTION('ref_axis',(1.,0.,0.));
#30454=DIRECTION('',(0.,0.,1.));
#30455=DIRECTION('center_axis',(0.,0.,1.));
#30456=DIRECTION('ref_axis',(1.,0.,0.));
#30457=DIRECTION('center_axis',(0.,0.,1.));
#30458=DIRECTION('ref_axis',(1.,0.,0.));
#30459=DIRECTION('',(0.,0.,-1.));
#30460=DIRECTION('center_axis',(0.,0.,1.));
#30461=DIRECTION('ref_axis',(1.,0.,0.));
#30462=DIRECTION('',(0.,0.,1.));
#30463=DIRECTION('center_axis',(0.,0.,1.));
#30464=DIRECTION('ref_axis',(1.,0.,0.));
#30465=DIRECTION('center_axis',(0.,0.,1.));
#30466=DIRECTION('ref_axis',(1.,0.,0.));
#30467=DIRECTION('',(0.,0.,-1.));
#30468=DIRECTION('center_axis',(0.,0.,1.));
#30469=DIRECTION('ref_axis',(1.,0.,0.));
#30470=DIRECTION('',(0.,0.,1.));
#30471=DIRECTION('center_axis',(0.,0.,1.));
#30472=DIRECTION('ref_axis',(1.,0.,0.));
#30473=DIRECTION('center_axis',(0.,0.,1.));
#30474=DIRECTION('ref_axis',(1.,0.,0.));
#30475=DIRECTION('',(0.,0.,-1.));
#30476=DIRECTION('center_axis',(0.,0.,1.));
#30477=DIRECTION('ref_axis',(1.,0.,0.));
#30478=DIRECTION('',(0.,0.,1.));
#30479=DIRECTION('center_axis',(0.,0.,1.));
#30480=DIRECTION('ref_axis',(1.,0.,0.));
#30481=DIRECTION('center_axis',(0.,0.,1.));
#30482=DIRECTION('ref_axis',(1.,0.,0.));
#30483=DIRECTION('center_axis',(0.,0.,-1.));
#30484=DIRECTION('ref_axis',(-1.,0.,0.));
#30485=DIRECTION('center_axis',(0.,0.,1.));
#30486=DIRECTION('ref_axis',(1.,0.,0.));
#30487=DIRECTION('center_axis',(0.,0.,1.));
#30488=DIRECTION('ref_axis',(1.,0.,0.));
#30489=DIRECTION('center_axis',(0.,0.,-1.));
#30490=DIRECTION('ref_axis',(-1.,0.,0.));
#30491=DIRECTION('center_axis',(0.,0.,-1.));
#30492=DIRECTION('ref_axis',(-1.,0.,0.));
#30493=DIRECTION('center_axis',(0.,0.,-1.));
#30494=DIRECTION('ref_axis',(1.,0.,0.));
#30495=DIRECTION('center_axis',(0.,0.,1.));
#30496=DIRECTION('ref_axis',(-1.,0.,0.));
#30497=DIRECTION('center_axis',(0.,0.,-1.));
#30498=DIRECTION('ref_axis',(-1.,0.,0.));
#30499=DIRECTION('center_axis',(0.,0.,-1.));
#30500=DIRECTION('ref_axis',(1.,0.,0.));
#30501=DIRECTION('center_axis',(0.,0.,1.));
#30502=DIRECTION('ref_axis',(-1.,-5.20417042793042E-15,0.));
#30503=DIRECTION('center_axis',(0.,0.,1.));
#30504=DIRECTION('ref_axis',(1.,0.,0.));
#30505=DIRECTION('center_axis',(0.,0.,-1.));
#30506=DIRECTION('ref_axis',(1.,0.,0.));
#30507=DIRECTION('center_axis',(0.,0.,1.));
#30508=DIRECTION('ref_axis',(-1.,-3.46944695195361E-15,0.));
#30509=DIRECTION('center_axis',(0.,0.,1.));
#30510=DIRECTION('ref_axis',(1.,0.,0.));
#30511=DIRECTION('center_axis',(0.,0.,-1.));
#30512=DIRECTION('ref_axis',(1.,0.,0.));
#30513=DIRECTION('center_axis',(0.,0.,1.));
#30514=DIRECTION('ref_axis',(-1.,5.42101086242752E-15,0.));
#30515=DIRECTION('center_axis',(0.,0.,1.));
#30516=DIRECTION('ref_axis',(1.,0.,0.));
#30517=DIRECTION('center_axis',(0.,0.,-1.));
#30518=DIRECTION('ref_axis',(1.,0.,0.));
#30519=DIRECTION('center_axis',(0.,0.,1.));
#30520=DIRECTION('ref_axis',(-1.,-1.73472347597681E-15,0.));
#30521=DIRECTION('center_axis',(0.,0.,1.));
#30522=DIRECTION('ref_axis',(1.,0.,0.));
#30523=DIRECTION('center_axis',(0.,0.,-1.));
#30524=DIRECTION('ref_axis',(1.,0.,0.));
#30525=DIRECTION('center_axis',(0.,0.,1.));
#30526=DIRECTION('ref_axis',(-1.,8.67361737988403E-15,0.));
#30527=DIRECTION('center_axis',(0.,0.,1.));
#30528=DIRECTION('ref_axis',(1.,0.,0.));
#30529=DIRECTION('center_axis',(0.,0.,1.));
#30530=DIRECTION('ref_axis',(1.,0.,0.));
#30531=DIRECTION('center_axis',(0.,0.,-1.));
#30532=DIRECTION('ref_axis',(-1.,0.,0.));
#30533=DIRECTION('center_axis',(0.,0.,1.));
#30534=DIRECTION('ref_axis',(1.,0.,0.));
#30535=DIRECTION('center_axis',(0.,0.,1.));
#30536=DIRECTION('ref_axis',(1.,0.,0.));
#30537=DIRECTION('center_axis',(0.,0.,-1.));
#30538=DIRECTION('ref_axis',(-1.,0.,0.));
#30539=DIRECTION('center_axis',(0.,0.,1.));
#30540=DIRECTION('ref_axis',(1.,0.,0.));
#30541=DIRECTION('center_axis',(0.,0.,-1.));
#30542=DIRECTION('ref_axis',(1.,0.,0.));
#30543=DIRECTION('center_axis',(0.,0.,1.));
#30544=DIRECTION('ref_axis',(-1.,1.73472347597681E-15,0.));
#30545=DIRECTION('center_axis',(0.,0.,1.));
#30546=DIRECTION('ref_axis',(1.,0.,0.));
#30547=DIRECTION('center_axis',(0.,0.,-1.));
#30548=DIRECTION('ref_axis',(1.,0.,0.));
#30549=DIRECTION('center_axis',(0.,0.,1.));
#30550=DIRECTION('ref_axis',(-1.,0.,0.));
#30551=DIRECTION('center_axis',(0.,0.,-1.));
#30552=DIRECTION('ref_axis',(-1.,0.,0.));
#30553=DIRECTION('center_axis',(0.,0.,-1.));
#30554=DIRECTION('ref_axis',(1.,0.,0.));
#30555=DIRECTION('center_axis',(0.,0.,1.));
#30556=DIRECTION('ref_axis',(-1.,0.,0.));
#30557=DIRECTION('center_axis',(0.,0.,-1.));
#30558=DIRECTION('ref_axis',(-1.,0.,0.));
#30559=DIRECTION('center_axis',(0.,0.,-1.));
#30560=DIRECTION('ref_axis',(1.,0.,0.));
#30561=DIRECTION('center_axis',(0.,0.,1.));
#30562=DIRECTION('ref_axis',(-1.,-1.64798730217797E-14,0.));
#30563=DIRECTION('center_axis',(0.,0.,1.));
#30564=DIRECTION('ref_axis',(1.,0.,0.));
#30565=DIRECTION('center_axis',(0.,0.,-1.));
#30566=DIRECTION('ref_axis',(1.,0.,0.));
#30567=DIRECTION('center_axis',(0.,0.,1.));
#30568=DIRECTION('ref_axis',(-1.,-1.73472347597681E-14,0.));
#30569=DIRECTION('center_axis',(0.,0.,1.));
#30570=DIRECTION('ref_axis',(1.,0.,0.));
#30571=DIRECTION('center_axis',(0.,0.,-1.));
#30572=DIRECTION('ref_axis',(1.,0.,0.));
#30573=DIRECTION('center_axis',(0.,0.,1.));
#30574=DIRECTION('ref_axis',(-1.,1.95156391047391E-14,0.));
#30575=DIRECTION('center_axis',(0.,0.,-1.));
#30576=DIRECTION('ref_axis',(-1.,0.,0.));
#30577=DIRECTION('center_axis',(0.,-1.,0.));
#30578=DIRECTION('ref_axis',(0.,0.,-1.));
#30579=DIRECTION('',(0.,0.,1.));
#30580=DIRECTION('',(-1.,0.,0.));
#30581=DIRECTION('',(0.,0.,1.));
#30582=DIRECTION('',(1.,0.,0.));
#30583=DIRECTION('center_axis',(0.,0.,-1.));
#30584=DIRECTION('ref_axis',(-1.,0.,0.));
#30585=DIRECTION('',(-0.707106781186547,0.707106781186548,0.));
#30586=DIRECTION('',(-1.26161707343768E-16,1.,0.));
#30587=DIRECTION('',(0.707106781186562,0.707106781186533,0.));
#30588=DIRECTION('',(0.707106781186562,-0.707106781186533,0.));
#30589=DIRECTION('',(-1.26161707343768E-16,-1.,0.));
#30590=DIRECTION('',(-0.707106781186547,-0.707106781186548,0.));
#30591=DIRECTION('center_axis',(0.707106781186533,-0.707106781186562,0.));
#30592=DIRECTION('ref_axis',(0.707106781186562,0.707106781186533,0.));
#30593=DIRECTION('',(0.,0.,1.));
#30594=DIRECTION('',(-0.707106781186562,-0.707106781186533,0.));
#30595=DIRECTION('center_axis',(1.,1.26161707343768E-16,0.));
#30596=DIRECTION('ref_axis',(-1.26161707343768E-16,1.,0.));
#30597=DIRECTION('',(0.,0.,1.));
#30598=DIRECTION('',(1.26161707343768E-16,-1.,0.));
#30599=DIRECTION('center_axis',(0.707106781186548,0.707106781186547,0.));
#30600=DIRECTION('ref_axis',(-0.707106781186547,0.707106781186548,0.));
#30601=DIRECTION('',(0.707106781186547,-0.707106781186548,0.));
#30602=DIRECTION('center_axis',(-0.707106781186548,0.707106781186547,0.));
#30603=DIRECTION('ref_axis',(-0.707106781186547,-0.707106781186548,0.));
#30604=DIRECTION('',(0.,0.,1.));
#30605=DIRECTION('',(0.707106781186547,0.707106781186548,0.));
#30606=DIRECTION('center_axis',(-1.,1.26161707343768E-16,0.));
#30607=DIRECTION('ref_axis',(-1.26161707343768E-16,-1.,0.));
#30608=DIRECTION('',(0.,0.,1.));
#30609=DIRECTION('',(1.26161707343768E-16,1.,0.));
#30610=DIRECTION('center_axis',(-0.707106781186533,-0.707106781186562,0.));
#30611=DIRECTION('ref_axis',(0.707106781186562,-0.707106781186533,0.));
#30612=DIRECTION('',(-0.707106781186562,0.707106781186533,0.));
#30613=DIRECTION('center_axis',(-0.866025403784439,0.5,0.));
#30614=DIRECTION('ref_axis',(-0.5,-0.866025403784439,0.));
#30615=DIRECTION('',(0.,0.,-1.));
#30616=DIRECTION('',(0.,0.,-1.));
#30617=DIRECTION('',(0.5,0.866025403784439,0.));
#30618=DIRECTION('center_axis',(-0.866025403784438,-0.5,0.));
#30619=DIRECTION('ref_axis',(0.5,-0.866025403784438,0.));
#30620=DIRECTION('',(-0.5,0.866025403784438,0.));
#30621=DIRECTION('',(0.,0.,-1.));
#30622=DIRECTION('center_axis',(7.51157299368579E-16,-1.,0.));
#30623=DIRECTION('ref_axis',(1.,7.5115729936858E-16,0.));
#30624=DIRECTION('',(0.,0.,-1.));
#30625=DIRECTION('',(-1.,-7.5115729936858E-16,0.));
#30626=DIRECTION('center_axis',(0.866025403784439,-0.5,0.));
#30627=DIRECTION('ref_axis',(0.5,0.866025403784439,0.));
#30628=DIRECTION('',(0.,0.,-1.));
#30629=DIRECTION('',(-0.5,-0.866025403784439,0.));
#30630=DIRECTION('center_axis',(0.866025403784439,0.5,0.));
#30631=DIRECTION('ref_axis',(-0.5,0.866025403784439,0.));
#30632=DIRECTION('',(0.,0.,-1.));
#30633=DIRECTION('',(0.5,-0.866025403784438,0.));
#30634=DIRECTION('center_axis',(0.,1.,0.));
#30635=DIRECTION('ref_axis',(0.,0.,1.));
#30636=DIRECTION('',(1.,0.,0.));
#30637=DIRECTION('center_axis',(0.,0.,-1.));
#30638=DIRECTION('ref_axis',(-1.,0.,0.));
#30639=DIRECTION('center_axis',(0.,0.,-1.));
#30640=DIRECTION('ref_axis',(1.,0.,0.));
#30641=DIRECTION('',(0.707106781186546,-0.707106781186549,0.));
#30642=DIRECTION('center_axis',(0.,0.,1.));
#30643=DIRECTION('ref_axis',(1.,0.,0.));
#30644=DIRECTION('',(0.,-1.,0.));
#30645=DIRECTION('center_axis',(0.,0.,1.));
#30646=DIRECTION('ref_axis',(1.,0.,0.));
#30647=DIRECTION('',(-0.707106781186552,-0.707106781186543,0.));
#30648=DIRECTION('center_axis',(0.,0.,-1.));
#30649=DIRECTION('ref_axis',(1.,0.,0.));
#30650=DIRECTION('center_axis',(0.,0.,1.));
#30651=DIRECTION('ref_axis',(1.,0.,0.));
#30652=DIRECTION('center_axis',(0.,0.,-1.));
#30653=DIRECTION('ref_axis',(1.,0.,0.));
#30654=DIRECTION('',(-0.707106781186552,-0.707106781186543,0.));
#30655=DIRECTION('center_axis',(0.,0.,-1.));
#30656=DIRECTION('ref_axis',(1.,0.,0.));
#30657=DIRECTION('',(0.,-1.,0.));
#30658=DIRECTION('center_axis',(0.,0.,-1.));
#30659=DIRECTION('ref_axis',(1.,0.,0.));
#30660=DIRECTION('',(0.707106781186547,-0.707106781186547,0.));
#30661=DIRECTION('center_axis',(0.,0.,-1.));
#30662=DIRECTION('ref_axis',(1.,0.,0.));
#30663=DIRECTION('center_axis',(0.,0.,1.));
#30664=DIRECTION('ref_axis',(1.,0.,0.));
#30665=DIRECTION('center_axis',(0.,0.,-1.));
#30666=DIRECTION('ref_axis',(1.,0.,0.));
#30667=DIRECTION('',(0.707106781186546,-0.707106781186549,0.));
#30668=DIRECTION('',(1.,4.61786466713945E-17,0.));
#30669=DIRECTION('',(0.707106781186547,0.707106781186548,0.));
#30670=DIRECTION('center_axis',(0.,0.,-1.));
#30671=DIRECTION('ref_axis',(1.,0.,0.));
#30672=DIRECTION('center_axis',(0.,0.,1.));
#30673=DIRECTION('ref_axis',(1.,0.,0.));
#30674=DIRECTION('center_axis',(0.,0.,-1.));
#30675=DIRECTION('ref_axis',(1.,0.,0.));
#30676=DIRECTION('',(0.707106781186546,0.707106781186549,0.));
#30677=DIRECTION('center_axis',(0.,0.,-1.));
#30678=DIRECTION('ref_axis',(1.,0.,0.));
#30679=DIRECTION('',(0.,1.,0.));
#30680=DIRECTION('center_axis',(0.,0.,-1.));
#30681=DIRECTION('ref_axis',(1.,0.,0.));
#30682=DIRECTION('',(-0.707106781186546,0.707106781186549,0.));
#30683=DIRECTION('center_axis',(0.,0.,-1.));
#30684=DIRECTION('ref_axis',(1.,0.,0.));
#30685=DIRECTION('center_axis',(0.,0.,1.));
#30686=DIRECTION('ref_axis',(1.,0.,0.));
#30687=DIRECTION('center_axis',(0.,0.,-1.));
#30688=DIRECTION('ref_axis',(1.,0.,0.));
#30689=DIRECTION('',(-0.707106781186552,0.707106781186543,0.));
#30690=DIRECTION('center_axis',(0.,0.,1.));
#30691=DIRECTION('ref_axis',(1.,0.,0.));
#30692=DIRECTION('',(0.,1.,0.));
#30693=DIRECTION('center_axis',(0.,0.,1.));
#30694=DIRECTION('ref_axis',(1.,0.,0.));
#30695=DIRECTION('',(0.707106781186546,0.707106781186549,0.));
#30696=DIRECTION('',(1.,0.,0.));
#30697=DIRECTION('',(0.707106781186547,-0.707106781186548,0.));
#30698=DIRECTION('',(1.26352022694434E-16,-1.,0.));
#30699=DIRECTION('',(-0.707106781186562,-0.707106781186533,0.));
#30700=DIRECTION('',(-1.,-1.95534159233113E-16,0.));
#30701=DIRECTION('',(-0.707106781186561,0.707106781186534,0.));
#30702=DIRECTION('',(0.,1.,0.));
#30703=DIRECTION('',(0.707106781186546,0.707106781186549,0.));
#30704=DIRECTION('',(1.,0.,0.));
#30705=DIRECTION('center_axis',(-0.707106781186549,-0.707106781186546,0.));
#30706=DIRECTION('ref_axis',(0.707106781186546,-0.707106781186549,0.));
#30707=DIRECTION('',(0.707106781186546,-0.707106781186549,0.));
#30708=DIRECTION('',(0.,0.,1.));
#30709=DIRECTION('',(0.,0.,1.));
#30710=DIRECTION('center_axis',(0.,0.,1.));
#30711=DIRECTION('ref_axis',(1.,0.,0.));
#30712=DIRECTION('center_axis',(0.,0.,1.));
#30713=DIRECTION('ref_axis',(1.,0.,0.));
#30714=DIRECTION('',(0.,0.,1.));
#30715=DIRECTION('center_axis',(-1.,0.,0.));
#30716=DIRECTION('ref_axis',(0.,0.,1.));
#30717=DIRECTION('',(0.,-1.,0.));
#30718=DIRECTION('',(0.,0.,1.));
#30719=DIRECTION('center_axis',(0.,0.,1.));
#30720=DIRECTION('ref_axis',(1.,0.,0.));
#30721=DIRECTION('center_axis',(0.,0.,1.));
#30722=DIRECTION('ref_axis',(1.,0.,0.));
#30723=DIRECTION('',(0.,0.,1.));
#30724=DIRECTION('center_axis',(-0.707106781186543,0.707106781186552,0.));
#30725=DIRECTION('ref_axis',(-0.707106781186552,-0.707106781186543,0.));
#30726=DIRECTION('',(-0.707106781186552,-0.707106781186543,0.));
#30727=DIRECTION('',(0.,0.,1.));
#30728=DIRECTION('center_axis',(0.,0.,1.));
#30729=DIRECTION('ref_axis',(1.,0.,0.));
#30730=DIRECTION('center_axis',(0.,0.,-1.));
#30731=DIRECTION('ref_axis',(1.,0.,0.));
#30732=DIRECTION('',(0.,0.,1.));
#30733=DIRECTION('center_axis',(0.,0.,1.));
#30734=DIRECTION('ref_axis',(1.,0.,0.));
#30735=DIRECTION('center_axis',(0.,0.,1.));
#30736=DIRECTION('ref_axis',(1.,0.,0.));
#30737=DIRECTION('',(0.,0.,1.));
#30738=DIRECTION('center_axis',(0.,0.,1.));
#30739=DIRECTION('ref_axis',(1.,0.,0.));
#30740=DIRECTION('center_axis',(0.,0.,-1.));
#30741=DIRECTION('ref_axis',(1.,0.,0.));
#30742=DIRECTION('',(0.,0.,1.));
#30743=DIRECTION('center_axis',(-0.707106781186543,0.707106781186552,0.));
#30744=DIRECTION('ref_axis',(-0.707106781186552,-0.707106781186543,0.));
#30745=DIRECTION('',(-0.707106781186552,-0.707106781186543,0.));
#30746=DIRECTION('',(0.,0.,1.));
#30747=DIRECTION('center_axis',(0.,0.,1.));
#30748=DIRECTION('ref_axis',(1.,0.,0.));
#30749=DIRECTION('center_axis',(0.,0.,-1.));
#30750=DIRECTION('ref_axis',(1.,0.,0.));
#30751=DIRECTION('',(0.,0.,1.));
#30752=DIRECTION('center_axis',(-1.,0.,0.));
#30753=DIRECTION('ref_axis',(0.,0.,1.));
#30754=DIRECTION('',(0.,-1.,0.));
#30755=DIRECTION('',(0.,0.,1.));
#30756=DIRECTION('center_axis',(0.,0.,1.));
#30757=DIRECTION('ref_axis',(1.,0.,0.));
#30758=DIRECTION('center_axis',(0.,0.,-1.));
#30759=DIRECTION('ref_axis',(1.,0.,0.));
#30760=DIRECTION('',(0.,0.,1.));
#30761=DIRECTION('center_axis',(-0.707106781186548,-0.707106781186548,0.));
#30762=DIRECTION('ref_axis',(0.707106781186548,-0.707106781186548,0.));
#30763=DIRECTION('',(0.707106781186547,-0.707106781186547,0.));
#30764=DIRECTION('',(0.,0.,1.));
#30765=DIRECTION('center_axis',(0.,0.,1.));
#30766=DIRECTION('ref_axis',(1.,0.,0.));
#30767=DIRECTION('center_axis',(0.,0.,-1.));
#30768=DIRECTION('ref_axis',(1.,0.,0.));
#30769=DIRECTION('',(0.,0.,1.));
#30770=DIRECTION('center_axis',(0.,0.,1.));
#30771=DIRECTION('ref_axis',(1.,0.,0.));
#30772=DIRECTION('center_axis',(0.,0.,1.));
#30773=DIRECTION('ref_axis',(1.,0.,0.));
#30774=DIRECTION('',(0.,0.,1.));
#30775=DIRECTION('center_axis',(0.,0.,1.));
#30776=DIRECTION('ref_axis',(1.,0.,0.));
#30777=DIRECTION('center_axis',(0.,0.,-1.));
#30778=DIRECTION('ref_axis',(1.,0.,0.));
#30779=DIRECTION('',(0.,0.,1.));
#30780=DIRECTION('center_axis',(-0.707106781186549,-0.707106781186546,0.));
#30781=DIRECTION('ref_axis',(0.707106781186546,-0.707106781186549,0.));
#30782=DIRECTION('',(0.707106781186546,-0.707106781186549,0.));
#30783=DIRECTION('',(0.,0.,1.));
#30784=DIRECTION('center_axis',(4.61786466713945E-17,-1.,0.));
#30785=DIRECTION('ref_axis',(1.,4.61786466713945E-17,0.));
#30786=DIRECTION('',(1.,4.61786466713945E-17,0.));
#30787=DIRECTION('',(0.,0.,1.));
#30788=DIRECTION('center_axis',(0.707106781186548,-0.707106781186547,0.));
#30789=DIRECTION('ref_axis',(0.707106781186547,0.707106781186548,0.));
#30790=DIRECTION('',(0.707106781186547,0.707106781186548,0.));
#30791=DIRECTION('',(0.,0.,1.));
#30792=DIRECTION('center_axis',(0.,0.,1.));
#30793=DIRECTION('ref_axis',(1.,0.,0.));
#30794=DIRECTION('center_axis',(0.,0.,-1.));
#30795=DIRECTION('ref_axis',(1.,0.,0.));
#30796=DIRECTION('',(0.,0.,1.));
#30797=DIRECTION('center_axis',(0.,0.,1.));
#30798=DIRECTION('ref_axis',(1.,0.,0.));
#30799=DIRECTION('center_axis',(0.,0.,1.));
#30800=DIRECTION('ref_axis',(1.,0.,0.));
#30801=DIRECTION('',(0.,0.,1.));
#30802=DIRECTION('center_axis',(0.,0.,1.));
#30803=DIRECTION('ref_axis',(1.,0.,0.));
#30804=DIRECTION('center_axis',(0.,0.,-1.));
#30805=DIRECTION('ref_axis',(1.,0.,0.));
#30806=DIRECTION('',(0.,0.,1.));
#30807=DIRECTION('center_axis',(0.70710678118655,-0.707106781186545,0.));
#30808=DIRECTION('ref_axis',(0.707106781186545,0.70710678118655,0.));
#30809=DIRECTION('',(0.707106781186546,0.707106781186549,0.));
#30810=DIRECTION('',(0.,0.,1.));
#30811=DIRECTION('center_axis',(0.,0.,1.));
#30812=DIRECTION('ref_axis',(1.,0.,0.));
#30813=DIRECTION('center_axis',(0.,0.,-1.));
#30814=DIRECTION('ref_axis',(1.,0.,0.));
#30815=DIRECTION('',(0.,0.,1.));
#30816=DIRECTION('center_axis',(1.,0.,0.));
#30817=DIRECTION('ref_axis',(0.,0.,-1.));
#30818=DIRECTION('',(0.,1.,0.));
#30819=DIRECTION('',(0.,0.,1.));
#30820=DIRECTION('center_axis',(0.,0.,1.));
#30821=DIRECTION('ref_axis',(1.,0.,0.));
#30822=DIRECTION('center_axis',(0.,0.,-1.));
#30823=DIRECTION('ref_axis',(1.,0.,0.));
#30824=DIRECTION('',(0.,0.,1.));
#30825=DIRECTION('center_axis',(0.707106781186549,0.707106781186546,0.));
#30826=DIRECTION('ref_axis',(-0.707106781186546,0.707106781186549,0.));
#30827=DIRECTION('',(-0.707106781186546,0.707106781186549,0.));
#30828=DIRECTION('',(0.,0.,1.));
#30829=DIRECTION('center_axis',(0.,0.,1.));
#30830=DIRECTION('ref_axis',(1.,0.,0.));
#30831=DIRECTION('center_axis',(0.,0.,-1.));
#30832=DIRECTION('ref_axis',(1.,0.,0.));
#30833=DIRECTION('',(0.,0.,1.));
#30834=DIRECTION('center_axis',(0.,0.,1.));
#30835=DIRECTION('ref_axis',(1.,0.,0.));
#30836=DIRECTION('center_axis',(0.,0.,1.));
#30837=DIRECTION('ref_axis',(1.,0.,0.));
#30838=DIRECTION('',(0.,0.,1.));
#30839=DIRECTION('center_axis',(0.,0.,1.));
#30840=DIRECTION('ref_axis',(1.,0.,0.));
#30841=DIRECTION('center_axis',(0.,0.,-1.));
#30842=DIRECTION('ref_axis',(1.,0.,0.));
#30843=DIRECTION('',(0.,0.,1.));
#30844=DIRECTION('center_axis',(0.707106781186543,0.707106781186552,0.));
#30845=DIRECTION('ref_axis',(-0.707106781186553,0.707106781186543,0.));
#30846=DIRECTION('',(-0.707106781186552,0.707106781186543,0.));
#30847=DIRECTION('',(0.,0.,1.));
#30848=DIRECTION('center_axis',(0.,0.,1.));
#30849=DIRECTION('ref_axis',(1.,0.,0.));
#30850=DIRECTION('center_axis',(0.,0.,1.));
#30851=DIRECTION('ref_axis',(1.,0.,0.));
#30852=DIRECTION('',(0.,0.,1.));
#30853=DIRECTION('center_axis',(1.,0.,0.));
#30854=DIRECTION('ref_axis',(0.,0.,-1.));
#30855=DIRECTION('',(0.,1.,0.));
#30856=DIRECTION('',(0.,0.,1.));
#30857=DIRECTION('center_axis',(0.,0.,1.));
#30858=DIRECTION('ref_axis',(1.,0.,0.));
#30859=DIRECTION('center_axis',(0.,0.,1.));
#30860=DIRECTION('ref_axis',(1.,0.,0.));
#30861=DIRECTION('',(0.,0.,1.));
#30862=DIRECTION('center_axis',(0.707106781186549,-0.707106781186546,0.));
#30863=DIRECTION('ref_axis',(0.707106781186546,0.707106781186549,0.));
#30864=DIRECTION('',(0.707106781186546,0.707106781186549,0.));
#30865=DIRECTION('',(0.,0.,1.));
#30866=DIRECTION('center_axis',(0.,-1.,0.));
#30867=DIRECTION('ref_axis',(0.,0.,-1.));
#30868=DIRECTION('',(1.,0.,0.));
#30869=DIRECTION('',(0.,0.,1.));
#30870=DIRECTION('center_axis',(-0.707106781186548,-0.707106781186547,0.));
#30871=DIRECTION('ref_axis',(0.707106781186547,-0.707106781186548,0.));
#30872=DIRECTION('',(0.707106781186547,-0.707106781186548,0.));
#30873=DIRECTION('',(0.,0.,1.));
#30874=DIRECTION('center_axis',(-1.,-1.26352022694434E-16,0.));
#30875=DIRECTION('ref_axis',(1.26352022694434E-16,-1.,0.));
#30876=DIRECTION('',(1.26352022694434E-16,-1.,0.));
#30877=DIRECTION('',(0.,0.,1.));
#30878=DIRECTION('center_axis',(-0.707106781186533,0.707106781186562,0.));
#30879=DIRECTION('ref_axis',(-0.707106781186562,-0.707106781186533,0.));
#30880=DIRECTION('',(-0.707106781186562,-0.707106781186533,0.));
#30881=DIRECTION('',(0.,0.,1.));
#30882=DIRECTION('center_axis',(-1.95534159233113E-16,1.,0.));
#30883=DIRECTION('ref_axis',(-1.,-1.95534159233113E-16,0.));
#30884=DIRECTION('',(-1.,-1.95534159233113E-16,0.));
#30885=DIRECTION('',(0.,0.,1.));
#30886=DIRECTION('center_axis',(0.707106781186534,0.707106781186561,0.));
#30887=DIRECTION('ref_axis',(-0.707106781186561,0.707106781186534,0.));
#30888=DIRECTION('',(-0.707106781186561,0.707106781186534,0.));
#30889=DIRECTION('',(0.,0.,1.));
#30890=DIRECTION('center_axis',(1.,0.,0.));
#30891=DIRECTION('ref_axis',(0.,0.,-1.));
#30892=DIRECTION('',(0.,1.,0.));
#30893=DIRECTION('',(0.,0.,1.));
#30894=DIRECTION('center_axis',(0.707106781186549,-0.707106781186546,0.));
#30895=DIRECTION('ref_axis',(0.707106781186546,0.707106781186549,0.));
#30896=DIRECTION('',(0.707106781186546,0.707106781186549,0.));
#30897=DIRECTION('',(0.,0.,1.));
#30898=DIRECTION('center_axis',(0.,-1.,0.));
#30899=DIRECTION('ref_axis',(0.,0.,-1.));
#30900=DIRECTION('',(1.,0.,0.));
#30901=DIRECTION('center_axis',(-1.30104260698261E-15,1.,-1.73611473352215E-31));
#30902=DIRECTION('ref_axis',(-1.,-1.30104260698261E-15,0.));
#30903=DIRECTION('center_axis',(-1.30104260698261E-15,1.,-1.73611473352215E-31));
#30904=DIRECTION('ref_axis',(-1.,-1.30104260698261E-15,0.));
#30905=DIRECTION('',(4.33680868994202E-17,0.,1.));
#30906=DIRECTION('center_axis',(-1.30104260698261E-15,1.,-1.73611473352215E-31));
#30907=DIRECTION('ref_axis',(-1.,-1.30104260698261E-15,2.25875923892257E-46));
#30908=DIRECTION('',(4.33680868994202E-17,0.,-1.));
#30909=DIRECTION('center_axis',(0.,0.,-1.));
#30910=DIRECTION('ref_axis',(-1.,0.,0.));
#30911=DIRECTION('',(1.,0.,0.));
#30912=DIRECTION('',(-1.73472347597681E-16,1.,0.));
#30913=DIRECTION('center_axis',(0.,0.,1.));
#30914=DIRECTION('ref_axis',(1.,0.,0.));
#30915=DIRECTION('',(-1.73472347597681E-16,-1.,0.));
#30916=DIRECTION('',(1.,0.,0.));
#30917=DIRECTION('',(0.707106781186562,0.707106781186533,0.));
#30918=DIRECTION('',(-1.26161707343768E-16,1.,0.));
#30919=DIRECTION('',(-0.707106781186547,0.707106781186548,0.));
#30920=DIRECTION('',(1.,0.,0.));
#30921=DIRECTION('',(0.707106781186546,0.707106781186549,0.));
#30922=DIRECTION('center_axis',(0.,0.,1.));
#30923=DIRECTION('ref_axis',(-1.,0.,0.));
#30924=DIRECTION('',(0.,1.,0.));
#30925=DIRECTION('center_axis',(0.,0.,1.));
#30926=DIRECTION('ref_axis',(-1.,0.,0.));
#30927=DIRECTION('',(-0.707106781186549,0.707106781186546,0.));
#30928=DIRECTION('center_axis',(0.,0.,-1.));
#30929=DIRECTION('ref_axis',(-1.,0.,0.));
#30930=DIRECTION('center_axis',(0.,0.,1.));
#30931=DIRECTION('ref_axis',(1.,0.,0.));
#30932=DIRECTION('center_axis',(0.,0.,-1.));
#30933=DIRECTION('ref_axis',(-1.,0.,0.));
#30934=DIRECTION('',(-0.707106781186549,0.707106781186546,0.));
#30935=DIRECTION('center_axis',(0.,0.,-1.));
#30936=DIRECTION('ref_axis',(-1.,0.,0.));
#30937=DIRECTION('',(0.,1.,0.));
#30938=DIRECTION('center_axis',(0.,0.,-1.));
#30939=DIRECTION('ref_axis',(-1.,0.,0.));
#30940=DIRECTION('',(0.707106781186546,0.707106781186549,0.));
#30941=DIRECTION('center_axis',(0.,0.,-1.));
#30942=DIRECTION('ref_axis',(-1.,0.,0.));
#30943=DIRECTION('center_axis',(0.,0.,1.));
#30944=DIRECTION('ref_axis',(1.,0.,0.));
#30945=DIRECTION('center_axis',(0.,0.,-1.));
#30946=DIRECTION('ref_axis',(-1.,0.,0.));
#30947=DIRECTION('',(0.707106781186546,0.707106781186549,0.));
#30948=DIRECTION('',(1.,1.22464679914735E-16,0.));
#30949=DIRECTION('',(0.707106781186546,-0.707106781186549,0.));
#30950=DIRECTION('center_axis',(0.,0.,-1.));
#30951=DIRECTION('ref_axis',(-1.,0.,0.));
#30952=DIRECTION('center_axis',(0.,0.,1.));
#30953=DIRECTION('ref_axis',(1.,0.,0.));
#30954=DIRECTION('center_axis',(0.,0.,-1.));
#30955=DIRECTION('ref_axis',(-1.,0.,0.));
#30956=DIRECTION('',(0.707106781186546,-0.707106781186549,0.));
#30957=DIRECTION('center_axis',(0.,0.,-1.));
#30958=DIRECTION('ref_axis',(-1.,0.,0.));
#30959=DIRECTION('',(0.,-1.,0.));
#30960=DIRECTION('center_axis',(0.,0.,-1.));
#30961=DIRECTION('ref_axis',(-1.,0.,0.));
#30962=DIRECTION('',(-0.707106781186549,-0.707106781186546,0.));
#30963=DIRECTION('center_axis',(0.,0.,-1.));
#30964=DIRECTION('ref_axis',(-1.,0.,0.));
#30965=DIRECTION('center_axis',(0.,0.,1.));
#30966=DIRECTION('ref_axis',(1.,0.,0.));
#30967=DIRECTION('center_axis',(0.,0.,-1.));
#30968=DIRECTION('ref_axis',(-1.,0.,0.));
#30969=DIRECTION('',(-0.707106781186549,-0.707106781186546,0.));
#30970=DIRECTION('center_axis',(0.,0.,1.));
#30971=DIRECTION('ref_axis',(-1.,-3.46944695195361E-15,0.));
#30972=DIRECTION('',(0.,-1.,0.));
#30973=DIRECTION('center_axis',(0.,0.,1.));
#30974=DIRECTION('ref_axis',(-1.,0.,0.));
#30975=DIRECTION('',(0.707106781186546,-0.707106781186549,0.));
#30976=DIRECTION('',(1.,-6.49101394191508E-16,0.));
#30977=DIRECTION('',(-0.707106781186547,-0.707106781186548,0.));
#30978=DIRECTION('',(-1.26161707343768E-16,-1.,0.));
#30979=DIRECTION('',(0.707106781186562,-0.707106781186533,0.));
#30980=DIRECTION('center_axis',(1.,1.30104260698261E-15,4.33680868994202E-17));
#30981=DIRECTION('ref_axis',(-1.30104260698261E-15,1.,5.08894400801554E-48));
#30982=DIRECTION('',(4.33680868994202E-17,0.,-1.));
#30983=DIRECTION('',(-1.30104260698261E-15,1.,-1.73611473352215E-31));
#30984=DIRECTION('center_axis',(-1.,-1.30104260698261E-15,4.33680868994202E-17));
#30985=DIRECTION('ref_axis',(1.30104260698261E-15,-1.,5.08894400801554E-48));
#30986=DIRECTION('',(4.33680868994202E-17,0.,1.));
#30987=DIRECTION('',(-1.30104260698261E-15,1.,-1.73611473352215E-31));
#30988=DIRECTION('center_axis',(-1.30104260698261E-15,1.,-1.73611473352215E-31));
#30989=DIRECTION('ref_axis',(-1.,-1.30104260698261E-15,2.25875923892257E-46));
#30990=DIRECTION('center_axis',(-1.30104260698261E-15,1.,-1.73611473352215E-31));
#30991=DIRECTION('ref_axis',(-1.,-1.30104260698261E-15,2.25875923892257E-46));
#30992=DIRECTION('center_axis',(-1.30104260698261E-15,1.,-1.73611473352215E-31));
#30993=DIRECTION('ref_axis',(-1.,-1.30104260698261E-15,0.));
#30994=DIRECTION('center_axis',(-1.30104260698261E-15,1.,-1.73611473352215E-31));
#30995=DIRECTION('ref_axis',(-1.,-1.30104260698261E-15,0.));
#30996=DIRECTION('',(-1.3010426069826E-16,0.,-1.));
#30997=DIRECTION('center_axis',(-1.30104260698261E-15,1.,-1.73611473352215E-31));
#30998=DIRECTION('ref_axis',(-1.,-1.30104260698261E-15,2.25875923892257E-46));
#30999=DIRECTION('',(1.3010426069826E-16,0.,1.));
#31000=DIRECTION('center_axis',(-6.49101394191508E-16,-1.,0.));
#31001=DIRECTION('ref_axis',(1.,-6.49101394191508E-16,0.));
#31002=DIRECTION('',(1.,-3.50803534070133E-16,0.));
#31003=DIRECTION('',(0.,0.,1.));
#31004=DIRECTION('',(0.,0.,1.));
#31005=DIRECTION('center_axis',(-0.707106781186548,0.707106781186547,0.));
#31006=DIRECTION('ref_axis',(-0.707106781186547,-0.707106781186548,0.));
#31007=DIRECTION('',(0.707106781186547,0.707106781186548,0.));
#31008=DIRECTION('',(0.,0.,1.));
#31009=DIRECTION('center_axis',(-1.,1.26161707343768E-16,0.));
#31010=DIRECTION('ref_axis',(-1.26161707343768E-16,-1.,0.));
#31011=DIRECTION('',(1.26161707343768E-16,1.,0.));
#31012=DIRECTION('',(0.,0.,1.));
#31013=DIRECTION('center_axis',(-0.707106781186533,-0.707106781186562,0.));
#31014=DIRECTION('ref_axis',(0.707106781186562,-0.707106781186533,0.));
#31015=DIRECTION('',(-0.707106781186562,0.707106781186533,0.));
#31016=DIRECTION('',(0.,0.,1.));
#31017=DIRECTION('center_axis',(0.,-1.,0.));
#31018=DIRECTION('ref_axis',(0.,0.,-1.));
#31019=DIRECTION('',(-1.,0.,0.));
#31020=DIRECTION('',(0.,0.,1.));
#31021=DIRECTION('',(-1.,0.,0.));
#31022=DIRECTION('',(0.,0.,1.));
#31023=DIRECTION('',(0.,0.,1.));
#31024=DIRECTION('center_axis',(0.707106781186533,-0.707106781186562,0.));
#31025=DIRECTION('ref_axis',(0.707106781186562,0.707106781186533,0.));
#31026=DIRECTION('',(-0.707106781186562,-0.707106781186533,0.));
#31027=DIRECTION('',(0.,0.,1.));
#31028=DIRECTION('center_axis',(1.,1.26161707343768E-16,0.));
#31029=DIRECTION('ref_axis',(-1.26161707343768E-16,1.,0.));
#31030=DIRECTION('',(1.26161707343768E-16,-1.,0.));
#31031=DIRECTION('',(0.,0.,1.));
#31032=DIRECTION('center_axis',(0.707106781186548,0.707106781186547,0.));
#31033=DIRECTION('ref_axis',(-0.707106781186547,0.707106781186548,0.));
#31034=DIRECTION('',(0.707106781186547,-0.707106781186548,0.));
#31035=DIRECTION('',(0.,0.,1.));
#31036=DIRECTION('center_axis',(0.,-1.,0.));
#31037=DIRECTION('ref_axis',(0.,0.,-1.));
#31038=DIRECTION('',(1.,0.,0.));
#31039=DIRECTION('',(0.,0.,1.));
#31040=DIRECTION('center_axis',(0.707106781186549,-0.707106781186546,0.));
#31041=DIRECTION('ref_axis',(0.707106781186546,0.707106781186549,0.));
#31042=DIRECTION('',(0.707106781186546,0.707106781186549,0.));
#31043=DIRECTION('',(0.,0.,1.));
#31044=DIRECTION('center_axis',(0.,0.,1.));
#31045=DIRECTION('ref_axis',(1.,0.,0.));
#31046=DIRECTION('center_axis',(0.,0.,1.));
#31047=DIRECTION('ref_axis',(1.,0.,0.));
#31048=DIRECTION('',(0.,0.,-1.));
#31049=DIRECTION('center_axis',(1.,0.,0.));
#31050=DIRECTION('ref_axis',(0.,0.,-1.));
#31051=DIRECTION('',(0.,1.,0.));
#31052=DIRECTION('',(0.,0.,1.));
#31053=DIRECTION('center_axis',(0.,0.,1.));
#31054=DIRECTION('ref_axis',(1.,0.,0.));
#31055=DIRECTION('center_axis',(0.,0.,1.));
#31056=DIRECTION('ref_axis',(1.,0.,0.));
#31057=DIRECTION('',(0.,0.,-1.));
#31058=DIRECTION('center_axis',(0.707106781186546,0.707106781186549,0.));
#31059=DIRECTION('ref_axis',(-0.707106781186549,0.707106781186546,0.));
#31060=DIRECTION('',(-0.707106781186549,0.707106781186546,0.));
#31061=DIRECTION('',(0.,0.,1.));
#31062=DIRECTION('center_axis',(0.,0.,1.));
#31063=DIRECTION('ref_axis',(1.,0.,0.));
#31064=DIRECTION('center_axis',(0.,0.,-1.));
#31065=DIRECTION('ref_axis',(1.,0.,0.));
#31066=DIRECTION('',(0.,0.,-1.));
#31067=DIRECTION('center_axis',(0.,0.,1.));
#31068=DIRECTION('ref_axis',(1.,0.,0.));
#31069=DIRECTION('center_axis',(0.,0.,1.));
#31070=DIRECTION('ref_axis',(1.,0.,0.));
#31071=DIRECTION('',(0.,0.,1.));
#31072=DIRECTION('center_axis',(0.,0.,1.));
#31073=DIRECTION('ref_axis',(1.,0.,0.));
#31074=DIRECTION('center_axis',(0.,0.,-1.));
#31075=DIRECTION('ref_axis',(1.,0.,0.));
#31076=DIRECTION('',(0.,0.,-1.));
#31077=DIRECTION('center_axis',(0.707106781186546,0.707106781186549,0.));
#31078=DIRECTION('ref_axis',(-0.707106781186549,0.707106781186546,0.));
#31079=DIRECTION('',(-0.707106781186548,0.707106781186547,0.));
#31080=DIRECTION('',(0.,0.,1.));
#31081=DIRECTION('center_axis',(0.,0.,-1.));
#31082=DIRECTION('ref_axis',(-1.,0.,0.));
#31083=DIRECTION('center_axis',(0.,0.,-1.));
#31084=DIRECTION('ref_axis',(1.,0.,0.));
#31085=DIRECTION('',(0.,0.,-1.));
#31086=DIRECTION('center_axis',(1.,0.,0.));
#31087=DIRECTION('ref_axis',(0.,0.,-1.));
#31088=DIRECTION('',(0.,1.,0.));
#31089=DIRECTION('',(0.,0.,1.));
#31090=DIRECTION('center_axis',(0.,0.,-1.));
#31091=DIRECTION('ref_axis',(-1.,0.,0.));
#31092=DIRECTION('center_axis',(0.,0.,-1.));
#31093=DIRECTION('ref_axis',(1.,0.,0.));
#31094=DIRECTION('',(0.,0.,-1.));
#31095=DIRECTION('center_axis',(0.707106781186549,-0.707106781186546,0.));
#31096=DIRECTION('ref_axis',(0.707106781186546,0.707106781186549,0.));
#31097=DIRECTION('',(0.707106781186545,0.70710678118655,0.));
#31098=DIRECTION('',(0.,0.,1.));
#31099=DIRECTION('center_axis',(0.,0.,1.));
#31100=DIRECTION('ref_axis',(1.,0.,0.));
#31101=DIRECTION('center_axis',(0.,0.,-1.));
#31102=DIRECTION('ref_axis',(1.,0.,0.));
#31103=DIRECTION('',(0.,0.,-1.));
#31104=DIRECTION('center_axis',(0.,0.,1.));
#31105=DIRECTION('ref_axis',(1.,0.,0.));
#31106=DIRECTION('center_axis',(0.,0.,1.));
#31107=DIRECTION('ref_axis',(1.,0.,0.));
#31108=DIRECTION('',(0.,0.,1.));
#31109=DIRECTION('center_axis',(0.,0.,1.));
#31110=DIRECTION('ref_axis',(1.,0.,0.));
#31111=DIRECTION('center_axis',(0.,0.,-1.));
#31112=DIRECTION('ref_axis',(1.,0.,0.));
#31113=DIRECTION('',(0.,0.,-1.));
#31114=DIRECTION('center_axis',(0.707106781186549,-0.707106781186546,0.));
#31115=DIRECTION('ref_axis',(0.707106781186546,0.707106781186549,0.));
#31116=DIRECTION('',(0.707106781186546,0.707106781186549,0.));
#31117=DIRECTION('',(0.,0.,1.));
#31118=DIRECTION('center_axis',(1.22464679914735E-16,-1.,0.));
#31119=DIRECTION('ref_axis',(1.,1.22464679914735E-16,0.));
#31120=DIRECTION('',(1.,1.22464679914735E-16,0.));
#31121=DIRECTION('',(0.,0.,1.));
#31122=DIRECTION('center_axis',(-0.707106781186549,-0.707106781186546,0.));
#31123=DIRECTION('ref_axis',(0.707106781186546,-0.707106781186549,0.));
#31124=DIRECTION('',(0.707106781186546,-0.707106781186549,0.));
#31125=DIRECTION('',(0.,0.,1.));
#31126=DIRECTION('center_axis',(0.,0.,1.));
#31127=DIRECTION('ref_axis',(1.,0.,0.));
#31128=DIRECTION('center_axis',(0.,0.,-1.));
#31129=DIRECTION('ref_axis',(1.,0.,0.));
#31130=DIRECTION('',(0.,0.,-1.));
#31131=DIRECTION('center_axis',(0.,0.,1.));
#31132=DIRECTION('ref_axis',(1.,0.,0.));
#31133=DIRECTION('center_axis',(0.,0.,1.));
#31134=DIRECTION('ref_axis',(1.,0.,0.));
#31135=DIRECTION('',(0.,0.,1.));
#31136=DIRECTION('center_axis',(0.,0.,1.));
#31137=DIRECTION('ref_axis',(1.,0.,0.));
#31138=DIRECTION('center_axis',(0.,0.,-1.));
#31139=DIRECTION('ref_axis',(1.,0.,0.));
#31140=DIRECTION('',(0.,0.,-1.));
#31141=DIRECTION('center_axis',(-0.707106781186549,-0.707106781186546,0.));
#31142=DIRECTION('ref_axis',(0.707106781186546,-0.707106781186549,0.));
#31143=DIRECTION('',(0.707106781186545,-0.70710678118655,0.));
#31144=DIRECTION('',(0.,0.,1.));
#31145=DIRECTION('center_axis',(0.,0.,-1.));
#31146=DIRECTION('ref_axis',(-1.,0.,0.));
#31147=DIRECTION('center_axis',(0.,0.,-1.));
#31148=DIRECTION('ref_axis',(1.,0.,0.));
#31149=DIRECTION('',(0.,0.,-1.));
#31150=DIRECTION('center_axis',(-1.,0.,0.));
#31151=DIRECTION('ref_axis',(0.,0.,1.));
#31152=DIRECTION('',(0.,-1.,0.));
#31153=DIRECTION('',(0.,0.,1.));
#31154=DIRECTION('center_axis',(0.,0.,-1.));
#31155=DIRECTION('ref_axis',(-1.,0.,0.));
#31156=DIRECTION('center_axis',(0.,0.,-1.));
#31157=DIRECTION('ref_axis',(1.,0.,0.));
#31158=DIRECTION('',(0.,0.,-1.));
#31159=DIRECTION('center_axis',(-0.707106781186546,0.707106781186549,0.));
#31160=DIRECTION('ref_axis',(-0.707106781186549,-0.707106781186546,0.));
#31161=DIRECTION('',(-0.707106781186548,-0.707106781186547,0.));
#31162=DIRECTION('',(0.,0.,1.));
#31163=DIRECTION('center_axis',(0.,0.,1.));
#31164=DIRECTION('ref_axis',(1.,0.,0.));
#31165=DIRECTION('center_axis',(0.,0.,-1.));
#31166=DIRECTION('ref_axis',(1.,0.,0.));
#31167=DIRECTION('',(0.,0.,-1.));
#31168=DIRECTION('center_axis',(0.,0.,1.));
#31169=DIRECTION('ref_axis',(1.,0.,0.));
#31170=DIRECTION('center_axis',(0.,0.,1.));
#31171=DIRECTION('ref_axis',(1.,0.,0.));
#31172=DIRECTION('',(0.,0.,1.));
#31173=DIRECTION('center_axis',(0.,0.,1.));
#31174=DIRECTION('ref_axis',(1.,0.,0.));
#31175=DIRECTION('center_axis',(0.,0.,-1.));
#31176=DIRECTION('ref_axis',(1.,0.,0.));
#31177=DIRECTION('',(0.,0.,-1.));
#31178=DIRECTION('center_axis',(-0.707106781186546,0.707106781186549,0.));
#31179=DIRECTION('ref_axis',(-0.707106781186549,-0.707106781186546,0.));
#31180=DIRECTION('',(-0.707106781186549,-0.707106781186546,0.));
#31181=DIRECTION('',(0.,0.,1.));
#31182=DIRECTION('center_axis',(0.,0.,1.));
#31183=DIRECTION('ref_axis',(1.,0.,0.));
#31184=DIRECTION('center_axis',(0.,0.,1.));
#31185=DIRECTION('ref_axis',(1.,0.,0.));
#31186=DIRECTION('',(0.,0.,-1.));
#31187=DIRECTION('center_axis',(-1.,0.,0.));
#31188=DIRECTION('ref_axis',(0.,0.,1.));
#31189=DIRECTION('',(0.,-1.,0.));
#31190=DIRECTION('',(0.,0.,1.));
#31191=DIRECTION('center_axis',(0.,0.,1.));
#31192=DIRECTION('ref_axis',(1.,0.,0.));
#31193=DIRECTION('center_axis',(0.,0.,1.));
#31194=DIRECTION('ref_axis',(1.,0.,0.));
#31195=DIRECTION('',(0.,0.,-1.));
#31196=DIRECTION('center_axis',(-0.707106781186549,-0.707106781186546,0.));
#31197=DIRECTION('ref_axis',(0.707106781186546,-0.707106781186549,0.));
#31198=DIRECTION('',(0.707106781186546,-0.707106781186549,0.));
#31199=DIRECTION('center_axis',(-1.30104260698261E-15,1.,-1.73611473352215E-31));
#31200=DIRECTION('ref_axis',(-1.,-1.30104260698261E-15,0.));
#31201=DIRECTION('center_axis',(-7.96355992932556E-18,-1.,0.));
#31202=DIRECTION('ref_axis',(1.,-7.96355992932556E-18,0.));
#31203=DIRECTION('',(0.,0.,1.));
#31204=DIRECTION('',(-1.,7.96355992932556E-18,0.));
#31205=DIRECTION('',(0.,0.,-1.));
#31206=DIRECTION('',(1.,-7.96355992932556E-18,0.));
#31207=DIRECTION('center_axis',(4.11015771401436E-16,-1.,0.));
#31208=DIRECTION('ref_axis',(1.,4.11015771401436E-16,0.));
#31209=DIRECTION('',(0.,0.,1.));
#31210=DIRECTION('',(-1.,-4.11015771401436E-16,0.));
#31211=DIRECTION('',(0.,0.,-1.));
#31212=DIRECTION('',(-1.,-4.11015771401436E-16,0.));
#31213=DIRECTION('center_axis',(-1.,-1.30104260698261E-15,1.3010426069826E-16));
#31214=DIRECTION('ref_axis',(1.30104260698261E-15,-1.,-3.07902494602621E-48));
#31215=DIRECTION('',(1.3010426069826E-16,0.,1.));
#31216=DIRECTION('',(-1.30104260698261E-15,1.,-1.73611473352215E-31));
#31217=DIRECTION('center_axis',(1.,1.30104260698261E-15,-1.3010426069826E-16));
#31218=DIRECTION('ref_axis',(-1.30104260698261E-15,1.,3.07902494602621E-48));
#31219=DIRECTION('',(-1.3010426069826E-16,0.,-1.));
#31220=DIRECTION('',(-1.30104260698261E-15,1.,-1.73611473352215E-31));
#31221=DIRECTION('center_axis',(-1.30104260698261E-15,1.,-1.73611473352215E-31));
#31222=DIRECTION('ref_axis',(-1.,-1.30104260698261E-15,2.25875923892257E-46));
#31223=DIRECTION('center_axis',(-1.30104260698261E-15,1.,-1.73611473352215E-31));
#31224=DIRECTION('ref_axis',(-1.,-1.30104260698261E-15,2.25875923892257E-46));
#31225=DIRECTION('center_axis',(0.,0.,-1.));
#31226=DIRECTION('ref_axis',(-1.,0.,0.));
#31227=DIRECTION('center_axis',(0.,0.,-1.));
#31228=DIRECTION('ref_axis',(1.,0.,0.));
#31229=DIRECTION('center_axis',(0.,0.,1.));
#31230=DIRECTION('ref_axis',(-1.,-1.73472347597681E-15,0.));
#31231=DIRECTION('',(0.,0.,-1.));
#31232=DIRECTION('center_axis',(0.,0.,1.));
#31233=DIRECTION('ref_axis',(1.,0.,0.));
#31234=DIRECTION('',(-0.258819045102518,0.965925826289069,0.));
#31235=DIRECTION('',(2.04085114820801E-16,1.,0.));
#31236=DIRECTION('',(-1.,1.2823896663807E-16,0.));
#31237=DIRECTION('',(-0.707106781186548,0.707106781186547,0.));
#31238=DIRECTION('center_axis',(1.,-2.04085114820801E-16,0.));
#31239=DIRECTION('ref_axis',(2.04085114820801E-16,1.,0.));
#31240=DIRECTION('',(0.,0.,1.));
#31241=DIRECTION('',(0.,1.,0.));
#31242=DIRECTION('',(0.,0.,1.));
#31243=DIRECTION('center_axis',(-1.,-2.04085114820801E-16,0.));
#31244=DIRECTION('ref_axis',(2.04085114820801E-16,-1.,0.));
#31245=DIRECTION('',(0.,0.,1.));
#31246=DIRECTION('',(0.,-1.,0.));
#31247=DIRECTION('',(0.,0.,-1.));
#31248=DIRECTION('',(2.04085114820801E-16,-1.,0.));
#31249=DIRECTION('center_axis',(0.,0.,1.));
#31250=DIRECTION('ref_axis',(1.,0.,0.));
#31251=DIRECTION('',(-0.258819045102518,-0.965925826289069,0.));
#31252=DIRECTION('center_axis',(0.,0.,-1.));
#31253=DIRECTION('ref_axis',(1.,-1.73472347597681E-15,0.));
#31254=DIRECTION('',(-0.707106781186557,-0.707106781186538,0.));
#31255=DIRECTION('',(-1.,-1.2823896663807E-16,0.));
#31256=DIRECTION('center_axis',(0.,0.,-1.));
#31257=DIRECTION('ref_axis',(-1.,0.,0.));
#31258=DIRECTION('',(0.,0.,1.));
#31259=DIRECTION('center_axis',(0.,0.,-1.));
#31260=DIRECTION('ref_axis',(1.,0.,0.));
#31261=DIRECTION('center_axis',(0.,0.,1.));
#31262=DIRECTION('ref_axis',(1.,0.,0.));
#31263=DIRECTION('',(1.,0.,0.));
#31264=DIRECTION('',(0.707106781186546,0.707106781186549,0.));
#31265=DIRECTION('',(0.,1.,0.));
#31266=DIRECTION('',(-0.707106781186561,0.707106781186534,0.));
#31267=DIRECTION('',(-1.,-1.95534159233113E-16,0.));
#31268=DIRECTION('',(-0.707106781186562,-0.707106781186533,0.));
#31269=DIRECTION('',(1.26352022694434E-16,-1.,0.));
#31270=DIRECTION('',(0.707106781186547,-0.707106781186548,0.));
#31271=DIRECTION('',(1.,0.,0.));
#31272=DIRECTION('',(0.707106781186546,0.707106781186549,0.));
#31273=DIRECTION('center_axis',(0.,0.,1.));
#31274=DIRECTION('ref_axis',(1.,0.,0.));
#31275=DIRECTION('',(0.,1.,0.));
#31276=DIRECTION('center_axis',(0.,0.,1.));
#31277=DIRECTION('ref_axis',(1.,0.,0.));
#31278=DIRECTION('',(-0.707106781186552,0.707106781186543,0.));
#31279=DIRECTION('center_axis',(0.,0.,-1.));
#31280=DIRECTION('ref_axis',(1.,0.,0.));
#31281=DIRECTION('center_axis',(0.,0.,1.));
#31282=DIRECTION('ref_axis',(1.,0.,0.));
#31283=DIRECTION('center_axis',(0.,0.,-1.));
#31284=DIRECTION('ref_axis',(1.,0.,0.));
#31285=DIRECTION('',(-0.707106781186546,0.707106781186549,0.));
#31286=DIRECTION('center_axis',(0.,0.,-1.));
#31287=DIRECTION('ref_axis',(1.,0.,0.));
#31288=DIRECTION('',(0.,1.,0.));
#31289=DIRECTION('center_axis',(0.,0.,-1.));
#31290=DIRECTION('ref_axis',(1.,0.,0.));
#31291=DIRECTION('',(0.707106781186546,0.707106781186549,0.));
#31292=DIRECTION('center_axis',(0.,0.,-1.));
#31293=DIRECTION('ref_axis',(1.,0.,0.));
#31294=DIRECTION('center_axis',(0.,0.,1.));
#31295=DIRECTION('ref_axis',(1.,0.,0.));
#31296=DIRECTION('center_axis',(0.,0.,-1.));
#31297=DIRECTION('ref_axis',(1.,0.,0.));
#31298=DIRECTION('',(0.707106781186547,0.707106781186548,0.));
#31299=DIRECTION('',(1.,4.61786466713945E-17,0.));
#31300=DIRECTION('',(0.707106781186546,-0.707106781186549,0.));
#31301=DIRECTION('center_axis',(0.,0.,-1.));
#31302=DIRECTION('ref_axis',(1.,0.,0.));
#31303=DIRECTION('center_axis',(0.,0.,1.));
#31304=DIRECTION('ref_axis',(1.,0.,0.));
#31305=DIRECTION('center_axis',(0.,0.,-1.));
#31306=DIRECTION('ref_axis',(1.,0.,0.));
#31307=DIRECTION('',(0.707106781186547,-0.707106781186547,0.));
#31308=DIRECTION('center_axis',(0.,0.,-1.));
#31309=DIRECTION('ref_axis',(1.,0.,0.));
#31310=DIRECTION('',(0.,-1.,0.));
#31311=DIRECTION('center_axis',(0.,0.,-1.));
#31312=DIRECTION('ref_axis',(1.,0.,0.));
#31313=DIRECTION('',(-0.707106781186552,-0.707106781186543,0.));
#31314=DIRECTION('center_axis',(0.,0.,-1.));
#31315=DIRECTION('ref_axis',(1.,0.,0.));
#31316=DIRECTION('center_axis',(0.,0.,1.));
#31317=DIRECTION('ref_axis',(1.,0.,0.));
#31318=DIRECTION('center_axis',(0.,0.,-1.));
#31319=DIRECTION('ref_axis',(1.,0.,0.));
#31320=DIRECTION('',(-0.707106781186552,-0.707106781186543,0.));
#31321=DIRECTION('center_axis',(0.,0.,1.));
#31322=DIRECTION('ref_axis',(1.,0.,0.));
#31323=DIRECTION('',(0.,-1.,0.));
#31324=DIRECTION('center_axis',(0.,0.,1.));
#31325=DIRECTION('ref_axis',(1.,0.,0.));
#31326=DIRECTION('',(0.707106781186546,-0.707106781186549,0.));
#31327=DIRECTION('center_axis',(-0.707106781186538,0.707106781186557,0.));
#31328=DIRECTION('ref_axis',(0.,0.,1.));
#31329=DIRECTION('',(0.,0.,-1.));
#31330=DIRECTION('',(-0.707106781186557,-0.707106781186538,0.));
#31331=DIRECTION('center_axis',(0.707106781186547,0.707106781186548,0.));
#31332=DIRECTION('ref_axis',(0.,0.,1.));
#31333=DIRECTION('',(0.,0.,1.));
#31334=DIRECTION('',(0.707106781186548,-0.707106781186547,0.));
#31335=DIRECTION('center_axis',(0.,0.,-1.));
#31336=DIRECTION('ref_axis',(-1.,0.,0.));
#31337=DIRECTION('',(-2.04085114820801E-16,-1.,0.));
#31338=DIRECTION('',(0.258819045102518,-0.965925826289069,0.));
#31339=DIRECTION('',(1.,-1.2823896663807E-16,0.));
#31340=DIRECTION('center_axis',(1.,-2.04085114820801E-16,0.));
#31341=DIRECTION('ref_axis',(2.04085114820801E-16,1.,0.));
#31342=DIRECTION('',(0.,0.,-1.));
#31343=DIRECTION('',(0.,-1.,0.));
#31344=DIRECTION('',(0.,0.,1.));
#31345=DIRECTION('center_axis',(0.,0.,1.));
#31346=DIRECTION('ref_axis',(1.,0.,0.));
#31347=DIRECTION('',(1.,1.2823896663807E-16,0.));
#31348=DIRECTION('',(-0.258819045102518,-0.965925826289069,0.));
#31349=DIRECTION('',(-2.04085114820801E-16,1.,0.));
#31350=DIRECTION('center_axis',(-1.,-2.04085114820801E-16,0.));
#31351=DIRECTION('ref_axis',(2.04085114820801E-16,-1.,0.));
#31352=DIRECTION('',(0.,0.,-1.));
#31353=DIRECTION('',(0.,1.,0.));
#31354=DIRECTION('',(0.,0.,-1.));
#31355=DIRECTION('center_axis',(-1.30104260698261E-15,1.,-1.73611473352215E-31));
#31356=DIRECTION('ref_axis',(-1.,-1.30104260698261E-15,0.));
#31357=DIRECTION('center_axis',(-0.965925826289069,-0.258819045102518,0.));
#31358=DIRECTION('ref_axis',(0.258819045102518,-0.965925826289069,0.));
#31359=DIRECTION('center_axis',(-0.965925826289069,-0.258819045102518,0.));
#31360=DIRECTION('ref_axis',(0.258819045102518,-0.965925826289069,0.));
#31361=DIRECTION('center_axis',(-0.965925826289069,-0.258819045102518,0.));
#31362=DIRECTION('ref_axis',(0.258819045102518,-0.965925826289069,0.));
#31363=DIRECTION('center_axis',(-1.2823896663807E-16,1.,0.));
#31364=DIRECTION('ref_axis',(-1.,-1.2823896663807E-16,0.));
#31365=DIRECTION('center_axis',(-1.2823896663807E-16,-1.,0.));
#31366=DIRECTION('ref_axis',(-1.,1.2823896663807E-16,0.));
#31367=DIRECTION('',(0.,0.,-1.));
#31368=DIRECTION('',(-1.,-1.2823896663807E-16,0.));
#31369=DIRECTION('',(0.,0.,1.));
#31370=DIRECTION('center_axis',(-1.,-2.04085114820801E-16,0.));
#31371=DIRECTION('ref_axis',(2.04085114820801E-16,-1.,0.));
#31372=DIRECTION('',(0.,0.,-1.));
#31373=DIRECTION('',(0.,1.,0.));
#31374=DIRECTION('',(2.04085114820801E-16,-1.,0.));
#31375=DIRECTION('center_axis',(-0.965925826289069,-0.258819045102518,0.));
#31376=DIRECTION('ref_axis',(0.258819045102518,-0.965925826289069,0.));
#31377=DIRECTION('center_axis',(-0.965925826289069,-0.258819045102518,0.));
#31378=DIRECTION('ref_axis',(0.258819045102518,-0.965925826289069,0.));
#31379=DIRECTION('',(0.258819045102518,-0.965925826289069,0.));
#31380=DIRECTION('',(0.,0.,1.));
#31381=DIRECTION('center_axis',(1.,-2.04085114820801E-16,0.));
#31382=DIRECTION('ref_axis',(2.04085114820801E-16,1.,0.));
#31383=DIRECTION('',(0.,0.,1.));
#31384=DIRECTION('',(0.,-1.,0.));
#31385=DIRECTION('',(2.04085114820801E-16,1.,0.));
#31386=DIRECTION('center_axis',(1.2823896663807E-16,1.,0.));
#31387=DIRECTION('ref_axis',(-1.,1.2823896663807E-16,0.));
#31388=DIRECTION('',(-1.,1.2823896663807E-16,0.));
#31389=DIRECTION('',(0.,0.,1.));
#31390=DIRECTION('center_axis',(-1.2823896663807E-16,-1.,0.));
#31391=DIRECTION('ref_axis',(-1.,1.2823896663807E-16,0.));
#31392=DIRECTION('center_axis',(0.965925826289069,-0.258819045102518,0.));
#31393=DIRECTION('ref_axis',(0.258819045102518,0.965925826289069,0.));
#31394=DIRECTION('center_axis',(0.965925826289069,-0.258819045102518,0.));
#31395=DIRECTION('ref_axis',(0.258819045102518,0.965925826289069,0.));
#31396=DIRECTION('',(0.258819045102518,0.965925826289069,0.));
#31397=DIRECTION('',(0.,0.,1.));
#31398=DIRECTION('center_axis',(0.965925826289069,-0.258819045102518,0.));
#31399=DIRECTION('ref_axis',(0.258819045102518,0.965925826289069,0.));
#31400=DIRECTION('center_axis',(0.965925826289069,-0.258819045102518,0.));
#31401=DIRECTION('ref_axis',(0.258819045102518,0.965925826289069,0.));
#31402=DIRECTION('center_axis',(0.965925826289069,-0.258819045102518,0.));
#31403=DIRECTION('ref_axis',(0.258819045102518,0.965925826289069,0.));
#31404=DIRECTION('center_axis',(0.,1.,0.));
#31405=DIRECTION('ref_axis',(0.,0.,1.));
#31406=DIRECTION('',(1.,0.,0.));
#31407=DIRECTION('',(0.,0.,-1.));
#31408=DIRECTION('',(0.,0.,-1.));
#31409=DIRECTION('center_axis',(-0.707106781186549,0.707106781186546,0.));
#31410=DIRECTION('ref_axis',(-0.707106781186546,-0.707106781186549,0.));
#31411=DIRECTION('',(0.707106781186546,0.707106781186549,0.));
#31412=DIRECTION('',(0.,0.,-1.));
#31413=DIRECTION('center_axis',(-1.,0.,0.));
#31414=DIRECTION('ref_axis',(0.,0.,1.));
#31415=DIRECTION('',(0.,1.,0.));
#31416=DIRECTION('',(0.,0.,-1.));
#31417=DIRECTION('center_axis',(-0.707106781186534,-0.707106781186561,0.));
#31418=DIRECTION('ref_axis',(0.707106781186561,-0.707106781186534,0.));
#31419=DIRECTION('',(-0.707106781186561,0.707106781186534,0.));
#31420=DIRECTION('',(0.,0.,-1.));
#31421=DIRECTION('center_axis',(1.95534159233113E-16,-1.,0.));
#31422=DIRECTION('ref_axis',(1.,1.95534159233113E-16,0.));
#31423=DIRECTION('',(-1.,-1.95534159233113E-16,0.));
#31424=DIRECTION('',(0.,0.,-1.));
#31425=DIRECTION('center_axis',(0.707106781186533,-0.707106781186562,0.));
#31426=DIRECTION('ref_axis',(0.707106781186562,0.707106781186533,0.));
#31427=DIRECTION('',(-0.707106781186562,-0.707106781186533,0.));
#31428=DIRECTION('',(0.,0.,-1.));
#31429=DIRECTION('center_axis',(1.,1.26352022694434E-16,0.));
#31430=DIRECTION('ref_axis',(-1.26352022694434E-16,1.,0.));
#31431=DIRECTION('',(1.26352022694434E-16,-1.,0.));
#31432=DIRECTION('',(0.,0.,-1.));
#31433=DIRECTION('center_axis',(0.707106781186548,0.707106781186547,0.));
#31434=DIRECTION('ref_axis',(-0.707106781186547,0.707106781186548,0.));
#31435=DIRECTION('',(0.707106781186547,-0.707106781186548,0.));
#31436=DIRECTION('',(0.,0.,-1.));
#31437=DIRECTION('center_axis',(0.,1.,0.));
#31438=DIRECTION('ref_axis',(0.,0.,1.));
#31439=DIRECTION('',(1.,0.,0.));
#31440=DIRECTION('',(0.,0.,-1.));
#31441=DIRECTION('center_axis',(-0.707106781186549,0.707106781186546,0.));
#31442=DIRECTION('ref_axis',(-0.707106781186546,-0.707106781186549,0.));
#31443=DIRECTION('',(0.707106781186546,0.707106781186549,0.));
#31444=DIRECTION('',(0.,0.,-1.));
#31445=DIRECTION('center_axis',(0.,0.,-1.));
#31446=DIRECTION('ref_axis',(-1.,0.,0.));
#31447=DIRECTION('center_axis',(0.,0.,1.));
#31448=DIRECTION('ref_axis',(1.,0.,0.));
#31449=DIRECTION('',(0.,0.,-1.));
#31450=DIRECTION('center_axis',(-1.,0.,0.));
#31451=DIRECTION('ref_axis',(0.,0.,1.));
#31452=DIRECTION('',(0.,1.,0.));
#31453=DIRECTION('',(0.,0.,-1.));
#31454=DIRECTION('center_axis',(0.,0.,-1.));
#31455=DIRECTION('ref_axis',(-1.,0.,0.));
#31456=DIRECTION('center_axis',(0.,0.,1.));
#31457=DIRECTION('ref_axis',(1.,0.,0.));
#31458=DIRECTION('',(0.,0.,-1.));
#31459=DIRECTION('center_axis',(-0.707106781186543,-0.707106781186552,0.));
#31460=DIRECTION('ref_axis',(0.707106781186553,-0.707106781186543,0.));
#31461=DIRECTION('',(-0.707106781186552,0.707106781186543,0.));
#31462=DIRECTION('',(0.,0.,-1.));
#31463=DIRECTION('center_axis',(0.,0.,-1.));
#31464=DIRECTION('ref_axis',(-1.,0.,0.));
#31465=DIRECTION('center_axis',(0.,0.,-1.));
#31466=DIRECTION('ref_axis',(1.,0.,0.));
#31467=DIRECTION('',(0.,0.,-1.));
#31468=DIRECTION('center_axis',(0.,0.,-1.));
#31469=DIRECTION('ref_axis',(-1.,0.,0.));
#31470=DIRECTION('center_axis',(0.,0.,1.));
#31471=DIRECTION('ref_axis',(1.,0.,0.));
#31472=DIRECTION('',(0.,0.,-1.));
#31473=DIRECTION('center_axis',(0.,0.,-1.));
#31474=DIRECTION('ref_axis',(-1.,0.,0.));
#31475=DIRECTION('center_axis',(0.,0.,-1.));
#31476=DIRECTION('ref_axis',(1.,0.,0.));
#31477=DIRECTION('',(0.,0.,-1.));
#31478=DIRECTION('center_axis',(-0.707106781186549,-0.707106781186546,0.));
#31479=DIRECTION('ref_axis',(0.707106781186546,-0.707106781186549,0.));
#31480=DIRECTION('',(-0.707106781186546,0.707106781186549,0.));
#31481=DIRECTION('',(0.,0.,-1.));
#31482=DIRECTION('center_axis',(0.,0.,-1.));
#31483=DIRECTION('ref_axis',(-1.,0.,0.));
#31484=DIRECTION('center_axis',(0.,0.,-1.));
#31485=DIRECTION('ref_axis',(1.,0.,0.));
#31486=DIRECTION('',(0.,0.,-1.));
#31487=DIRECTION('center_axis',(-1.,0.,0.));
#31488=DIRECTION('ref_axis',(0.,0.,1.));
#31489=DIRECTION('',(0.,1.,0.));
#31490=DIRECTION('',(0.,0.,-1.));
#31491=DIRECTION('center_axis',(0.,0.,-1.));
#31492=DIRECTION('ref_axis',(-1.,0.,0.));
#31493=DIRECTION('center_axis',(0.,0.,-1.));
#31494=DIRECTION('ref_axis',(1.,0.,0.));
#31495=DIRECTION('',(0.,0.,-1.));
#31496=DIRECTION('center_axis',(-0.70710678118655,0.707106781186545,0.));
#31497=DIRECTION('ref_axis',(-0.707106781186545,-0.70710678118655,0.));
#31498=DIRECTION('',(0.707106781186546,0.707106781186549,0.));
#31499=DIRECTION('',(0.,0.,-1.));
#31500=DIRECTION('center_axis',(0.,0.,-1.));
#31501=DIRECTION('ref_axis',(-1.,0.,0.));
#31502=DIRECTION('center_axis',(0.,0.,-1.));
#31503=DIRECTION('ref_axis',(1.,0.,0.));
#31504=DIRECTION('',(0.,0.,-1.));
#31505=DIRECTION('center_axis',(0.,0.,-1.));
#31506=DIRECTION('ref_axis',(-1.,0.,0.));
#31507=DIRECTION('center_axis',(0.,0.,1.));
#31508=DIRECTION('ref_axis',(1.,0.,0.));
#31509=DIRECTION('',(0.,0.,-1.));
#31510=DIRECTION('center_axis',(0.,0.,-1.));
#31511=DIRECTION('ref_axis',(-1.,0.,0.));
#31512=DIRECTION('center_axis',(0.,0.,-1.));
#31513=DIRECTION('ref_axis',(1.,0.,0.));
#31514=DIRECTION('',(0.,0.,-1.));
#31515=DIRECTION('center_axis',(-0.707106781186548,0.707106781186547,0.));
#31516=DIRECTION('ref_axis',(-0.707106781186547,-0.707106781186548,0.));
#31517=DIRECTION('',(0.707106781186547,0.707106781186548,0.));
#31518=DIRECTION('',(0.,0.,-1.));
#31519=DIRECTION('center_axis',(-4.61786466713945E-17,1.,0.));
#31520=DIRECTION('ref_axis',(-1.,-4.61786466713945E-17,0.));
#31521=DIRECTION('',(1.,4.61786466713945E-17,0.));
#31522=DIRECTION('',(0.,0.,-1.));
#31523=DIRECTION('center_axis',(0.707106781186549,0.707106781186546,0.));
#31524=DIRECTION('ref_axis',(-0.707106781186546,0.707106781186549,0.));
#31525=DIRECTION('',(0.707106781186546,-0.707106781186549,0.));
#31526=DIRECTION('',(0.,0.,-1.));
#31527=DIRECTION('center_axis',(0.,0.,-1.));
#31528=DIRECTION('ref_axis',(-1.,0.,0.));
#31529=DIRECTION('center_axis',(0.,0.,-1.));
#31530=DIRECTION('ref_axis',(1.,0.,0.));
#31531=DIRECTION('',(0.,0.,-1.));
#31532=DIRECTION('center_axis',(0.,0.,-1.));
#31533=DIRECTION('ref_axis',(-1.,0.,0.));
#31534=DIRECTION('center_axis',(0.,0.,1.));
#31535=DIRECTION('ref_axis',(1.,0.,0.));
#31536=DIRECTION('',(0.,0.,-1.));
#31537=DIRECTION('center_axis',(0.,0.,-1.));
#31538=DIRECTION('ref_axis',(-1.,0.,0.));
#31539=DIRECTION('center_axis',(0.,0.,-1.));
#31540=DIRECTION('ref_axis',(1.,0.,0.));
#31541=DIRECTION('',(0.,0.,-1.));
#31542=DIRECTION('center_axis',(0.707106781186548,0.707106781186548,0.));
#31543=DIRECTION('ref_axis',(-0.707106781186548,0.707106781186548,0.));
#31544=DIRECTION('',(0.707106781186547,-0.707106781186547,0.));
#31545=DIRECTION('',(0.,0.,-1.));
#31546=DIRECTION('center_axis',(0.,0.,-1.));
#31547=DIRECTION('ref_axis',(-1.,0.,0.));
#31548=DIRECTION('center_axis',(0.,0.,-1.));
#31549=DIRECTION('ref_axis',(1.,0.,0.));
#31550=DIRECTION('',(0.,0.,-1.));
#31551=DIRECTION('center_axis',(1.,0.,0.));
#31552=DIRECTION('ref_axis',(0.,0.,-1.));
#31553=DIRECTION('',(0.,-1.,0.));
#31554=DIRECTION('',(0.,0.,-1.));
#31555=DIRECTION('center_axis',(0.,0.,-1.));
#31556=DIRECTION('ref_axis',(-1.,0.,0.));
#31557=DIRECTION('center_axis',(0.,0.,-1.));
#31558=DIRECTION('ref_axis',(1.,0.,0.));
#31559=DIRECTION('',(0.,0.,-1.));
#31560=DIRECTION('center_axis',(0.707106781186543,-0.707106781186552,0.));
#31561=DIRECTION('ref_axis',(0.707106781186552,0.707106781186543,0.));
#31562=DIRECTION('',(-0.707106781186552,-0.707106781186543,0.));
#31563=DIRECTION('',(0.,0.,-1.));
#31564=DIRECTION('center_axis',(0.,0.,-1.));
#31565=DIRECTION('ref_axis',(-1.,0.,0.));
#31566=DIRECTION('center_axis',(0.,0.,-1.));
#31567=DIRECTION('ref_axis',(1.,0.,0.));
#31568=DIRECTION('',(0.,0.,-1.));
#31569=DIRECTION('center_axis',(0.,0.,-1.));
#31570=DIRECTION('ref_axis',(-1.,0.,0.));
#31571=DIRECTION('center_axis',(0.,0.,1.));
#31572=DIRECTION('ref_axis',(1.,0.,0.));
#31573=DIRECTION('',(0.,0.,-1.));
#31574=DIRECTION('center_axis',(0.,0.,-1.));
#31575=DIRECTION('ref_axis',(-1.,0.,0.));
#31576=DIRECTION('center_axis',(0.,0.,-1.));
#31577=DIRECTION('ref_axis',(1.,0.,0.));
#31578=DIRECTION('',(0.,0.,-1.));
#31579=DIRECTION('center_axis',(0.707106781186543,-0.707106781186552,0.));
#31580=DIRECTION('ref_axis',(0.707106781186552,0.707106781186543,0.));
#31581=DIRECTION('',(-0.707106781186552,-0.707106781186543,0.));
#31582=DIRECTION('',(0.,0.,-1.));
#31583=DIRECTION('center_axis',(0.,0.,-1.));
#31584=DIRECTION('ref_axis',(-1.,0.,0.));
#31585=DIRECTION('center_axis',(0.,0.,1.));
#31586=DIRECTION('ref_axis',(1.,0.,0.));
#31587=DIRECTION('',(0.,0.,-1.));
#31588=DIRECTION('center_axis',(1.,0.,0.));
#31589=DIRECTION('ref_axis',(0.,0.,-1.));
#31590=DIRECTION('',(0.,-1.,0.));
#31591=DIRECTION('',(0.,0.,-1.));
#31592=DIRECTION('center_axis',(0.,0.,-1.));
#31593=DIRECTION('ref_axis',(-1.,0.,0.));
#31594=DIRECTION('center_axis',(0.,0.,1.));
#31595=DIRECTION('ref_axis',(1.,0.,0.));
#31596=DIRECTION('',(0.,0.,-1.));
#31597=DIRECTION('center_axis',(0.707106781186549,0.707106781186546,0.));
#31598=DIRECTION('ref_axis',(-0.707106781186546,0.707106781186549,0.));
#31599=DIRECTION('',(0.707106781186546,-0.707106781186549,0.));
#31600=DIRECTION('center_axis',(-1.19636101791504E-15,1.,-1.04815936541451E-31));
#31601=DIRECTION('ref_axis',(-1.,-1.19636101791504E-15,0.));
#31602=DIRECTION('',(1.,1.19636101791504E-15,3.7386281809845E-17));
#31603=DIRECTION('',(-4.38061483832527E-16,-6.28895619248706E-31,-1.));
#31604=DIRECTION('',(-1.,-1.19636101791504E-15,0.));
#31605=DIRECTION('',(-8.76122967665054E-17,0.,1.));
#31606=DIRECTION('center_axis',(0.707106781186554,0.707106781186541,-3.09756245794624E-16));
#31607=DIRECTION('ref_axis',(4.38061483832527E-16,6.55212072256257E-31,
1.));
#31608=DIRECTION('',(-0.707106781186541,0.707106781186554,-2.64360933910924E-17));
#31609=DIRECTION('',(-4.38061483832527E-16,0.,-1.));
#31610=DIRECTION('',(0.707106781186541,-0.707106781186554,0.));
#31611=DIRECTION('center_axis',(0.,-1.,0.));
#31612=DIRECTION('ref_axis',(0.,0.,-1.));
#31613=DIRECTION('',(-1.,0.,0.));
#31614=DIRECTION('',(0.,0.,1.));
#31615=DIRECTION('',(1.,0.,0.));
#31616=DIRECTION('center_axis',(-0.707106781186533,-0.707106781186562,0.));
#31617=DIRECTION('ref_axis',(0.707106781186562,-0.707106781186533,0.));
#31618=DIRECTION('',(-0.707106781186562,0.707106781186533,0.));
#31619=DIRECTION('',(0.,0.,1.));
#31620=DIRECTION('',(0.707106781186562,-0.707106781186533,0.));
#31621=DIRECTION('center_axis',(-1.,1.26161707343768E-16,0.));
#31622=DIRECTION('ref_axis',(-1.26161707343768E-16,-1.,0.));
#31623=DIRECTION('',(1.26161707343768E-16,1.,0.));
#31624=DIRECTION('',(0.,0.,1.));
#31625=DIRECTION('',(-1.26161707343768E-16,-1.,0.));
#31626=DIRECTION('center_axis',(1.,1.26161707343768E-16,0.));
#31627=DIRECTION('ref_axis',(-1.26161707343768E-16,1.,0.));
#31628=DIRECTION('',(1.26161707343768E-16,-1.,0.));
#31629=DIRECTION('',(0.,0.,1.));
#31630=DIRECTION('',(-1.26161707343768E-16,1.,0.));
#31631=DIRECTION('',(0.,0.,1.));
#31632=DIRECTION('center_axis',(0.707106781186533,-0.707106781186562,0.));
#31633=DIRECTION('ref_axis',(0.707106781186562,0.707106781186533,0.));
#31634=DIRECTION('',(-0.707106781186562,-0.707106781186533,0.));
#31635=DIRECTION('',(0.,0.,1.));
#31636=DIRECTION('',(0.707106781186562,0.707106781186533,0.));
#31637=DIRECTION('center_axis',(0.,-1.,0.));
#31638=DIRECTION('ref_axis',(0.,0.,-1.));
#31639=DIRECTION('',(-1.,0.,0.));
#31640=DIRECTION('',(-8.76122967665054E-17,0.,1.));
#31641=DIRECTION('',(1.,0.,0.));
#31642=DIRECTION('center_axis',(-0.707106781186554,0.707106781186542,-6.19512491589247E-17));
#31643=DIRECTION('ref_axis',(8.76122967665054E-17,3.85000586821995E-33,
-1.));
#31644=DIRECTION('',(0.707106781186541,0.707106781186554,0.));
#31645=DIRECTION('',(-0.707106781186541,-0.707106781186554,-2.64360933910925E-17));
#31646=DIRECTION('center_axis',(1.,0.,0.));
#31647=DIRECTION('ref_axis',(0.,0.,-1.));
#31648=DIRECTION('',(0.,1.,0.));
#31649=DIRECTION('',(0.,0.,-1.));
#31650=DIRECTION('',(0.,1.,0.));
#31651=DIRECTION('',(0.,0.,1.));
#31652=DIRECTION('center_axis',(0.70710678118655,0.707106781186545,0.));
#31653=DIRECTION('ref_axis',(-0.707106781186545,0.70710678118655,0.));
#31654=DIRECTION('',(-0.707106781186545,0.70710678118655,0.));
#31655=DIRECTION('',(0.,0.,1.));
#31656=DIRECTION('',(-0.707106781186545,0.70710678118655,0.));
#31657=DIRECTION('center_axis',(0.,1.,0.));
#31658=DIRECTION('ref_axis',(0.,0.,1.));
#31659=DIRECTION('',(0.,0.,1.));
#31660=DIRECTION('',(-1.,0.,0.));
#31661=DIRECTION('',(-1.,0.,0.));
#31662=DIRECTION('center_axis',(0.707106781186549,-0.707106781186546,0.));
#31663=DIRECTION('ref_axis',(0.707106781186546,0.707106781186549,0.));
#31664=DIRECTION('',(0.,0.,1.));
#31665=DIRECTION('',(0.707106781186546,0.707106781186549,0.));
#31666=DIRECTION('',(0.707106781186546,0.707106781186549,0.));
#31667=DIRECTION('center_axis',(-1.62579519772897E-16,-1.,0.));
#31668=DIRECTION('ref_axis',(1.,-1.62579519772897E-16,0.));
#31669=DIRECTION('',(0.,0.,1.));
#31670=DIRECTION('',(1.,-1.62579519772897E-16,0.));
#31671=DIRECTION('',(1.,-1.62579519772897E-16,0.));
#31672=DIRECTION('center_axis',(-0.707106781186544,-0.707106781186551,0.));
#31673=DIRECTION('ref_axis',(0.707106781186551,-0.707106781186544,0.));
#31674=DIRECTION('',(0.,0.,1.));
#31675=DIRECTION('',(0.707106781186551,-0.707106781186544,0.));
#31676=DIRECTION('',(0.707106781186551,-0.707106781186544,0.));
#31677=DIRECTION('center_axis',(0.,1.,0.));
#31678=DIRECTION('ref_axis',(0.,0.,1.));
#31679=DIRECTION('',(-1.,0.,0.));
#31680=DIRECTION('',(0.,0.,1.));
#31681=DIRECTION('',(-1.,0.,0.));
#31682=DIRECTION('center_axis',(0.707106781186544,-0.707106781186551,0.));
#31683=DIRECTION('ref_axis',(0.707106781186551,0.707106781186544,0.));
#31684=DIRECTION('',(0.,0.,1.));
#31685=DIRECTION('',(0.707106781186551,0.707106781186544,0.));
#31686=DIRECTION('',(0.707106781186551,0.707106781186544,0.));
#31687=DIRECTION('center_axis',(1.62579519772897E-16,-1.,0.));
#31688=DIRECTION('ref_axis',(1.,1.62579519772897E-16,0.));
#31689=DIRECTION('',(0.,0.,1.));
#31690=DIRECTION('',(1.,1.62579519772897E-16,0.));
#31691=DIRECTION('',(1.,1.62579519772897E-16,0.));
#31692=DIRECTION('center_axis',(-0.707106781186549,-0.707106781186546,0.));
#31693=DIRECTION('ref_axis',(0.707106781186546,-0.707106781186549,0.));
#31694=DIRECTION('',(0.,0.,1.));
#31695=DIRECTION('',(0.707106781186546,-0.707106781186549,0.));
#31696=DIRECTION('',(0.707106781186546,-0.707106781186549,0.));
#31697=DIRECTION('center_axis',(0.,1.,0.));
#31698=DIRECTION('ref_axis',(0.,0.,1.));
#31699=DIRECTION('',(-1.,0.,0.));
#31700=DIRECTION('',(0.,0.,1.));
#31701=DIRECTION('',(-1.,0.,0.));
#31702=DIRECTION('center_axis',(-0.70710678118655,0.707106781186545,0.));
#31703=DIRECTION('ref_axis',(-0.707106781186545,-0.70710678118655,0.));
#31704=DIRECTION('',(-0.707106781186545,-0.70710678118655,0.));
#31705=DIRECTION('',(0.,0.,1.));
#31706=DIRECTION('',(-0.707106781186545,-0.70710678118655,0.));
#31707=DIRECTION('center_axis',(-1.,0.,0.));
#31708=DIRECTION('ref_axis',(0.,0.,1.));
#31709=DIRECTION('',(0.,-1.,0.));
#31710=DIRECTION('',(0.,0.,1.));
#31711=DIRECTION('',(0.,-1.,0.));
#31712=DIRECTION('center_axis',(-0.707106781186546,-0.707106781186549,0.));
#31713=DIRECTION('ref_axis',(0.707106781186549,-0.707106781186546,0.));
#31714=DIRECTION('',(0.707106781186549,-0.707106781186546,0.));
#31715=DIRECTION('',(0.,0.,1.));
#31716=DIRECTION('',(0.707106781186549,-0.707106781186546,0.));
#31717=DIRECTION('center_axis',(-1.,0.,0.));
#31718=DIRECTION('ref_axis',(0.,0.,1.));
#31719=DIRECTION('',(0.,-1.,0.));
#31720=DIRECTION('',(0.,0.,1.));
#31721=DIRECTION('',(0.,-1.,0.));
#31722=DIRECTION('center_axis',(1.2823896663807E-16,1.,0.));
#31723=DIRECTION('ref_axis',(-1.,1.2823896663807E-16,0.));
#31724=DIRECTION('center_axis',(-1.2823896663807E-16,-1.,0.));
#31725=DIRECTION('ref_axis',(-1.,1.2823896663807E-16,2.52323414687535E-15));
#31726=DIRECTION('',(1.,-1.2823896663807E-16,0.));
#31727=DIRECTION('',(0.,0.,-1.));
#31728=DIRECTION('center_axis',(1.,-2.04085114820801E-16,0.));
#31729=DIRECTION('ref_axis',(2.04085114820801E-16,1.,0.));
#31730=DIRECTION('',(0.,0.,1.));
#31731=DIRECTION('',(0.,1.,0.));
#31732=DIRECTION('',(-2.04085114820801E-16,-1.,0.));
#31733=DIRECTION('center_axis',(-0.965925826289069,-0.258819045102518,0.));
#31734=DIRECTION('ref_axis',(0.258819045102518,-0.965925826289069,0.));
#31735=DIRECTION('center_axis',(-0.965925826289069,-0.258819045102518,0.));
#31736=DIRECTION('ref_axis',(0.258819045102518,-0.965925826289069,0.));
#31737=DIRECTION('',(0.258819045102518,-0.965925826289069,0.));
#31738=DIRECTION('',(0.,0.,1.));
#31739=DIRECTION('center_axis',(0.965925826289069,-0.258819045102518,0.));
#31740=DIRECTION('ref_axis',(0.258819045102518,0.965925826289069,0.));
#31741=DIRECTION('center_axis',(0.965925826289069,-0.258819045102518,0.));
#31742=DIRECTION('ref_axis',(0.258819045102518,0.965925826289069,0.));
#31743=DIRECTION('',(0.258819045102518,0.965925826289069,0.));
#31744=DIRECTION('',(0.,0.,-1.));
#31745=DIRECTION('center_axis',(-1.,-2.04085114820801E-16,0.));
#31746=DIRECTION('ref_axis',(2.04085114820801E-16,-1.,0.));
#31747=DIRECTION('',(0.,0.,-1.));
#31748=DIRECTION('',(0.,-1.,0.));
#31749=DIRECTION('',(-2.04085114820801E-16,1.,0.));
#31750=DIRECTION('center_axis',(-1.2823896663807E-16,1.,0.));
#31751=DIRECTION('ref_axis',(-1.,-1.2823896663807E-16,0.));
#31752=DIRECTION('',(1.,1.2823896663807E-16,0.));
#31753=DIRECTION('center_axis',(-1.2823896663807E-16,-1.,0.));
#31754=DIRECTION('ref_axis',(-1.,1.2823896663807E-16,-2.52323414687536E-15));
#31755=DIRECTION('center_axis',(-0.61566147532566,-0.788010753606721,0.));
#31756=DIRECTION('ref_axis',(0.78801075360672,-0.61566147532566,0.));
#31757=DIRECTION('center_axis',(-0.615661475325663,-0.788010753606718,3.86575390646386E-15));
#31758=DIRECTION('ref_axis',(0.788010753606718,-0.615661475325663,-6.5758767605984E-13));
#31759=DIRECTION('',(0.78801075360672,-0.61566147532566,0.));
#31760=DIRECTION('',(0.,0.,1.));
#31761=DIRECTION('center_axis',(0.707106781186548,0.707106781186547,0.));
#31762=DIRECTION('ref_axis',(-0.707106781186547,0.707106781186548,0.));
#31763=DIRECTION('',(0.707106781186547,-0.707106781186548,0.));
#31764=DIRECTION('',(-0.707106781186547,0.707106781186548,0.));
#31765=DIRECTION('',(0.,0.,1.));
#31766=DIRECTION('center_axis',(-0.707106781186548,0.707106781186547,0.));
#31767=DIRECTION('ref_axis',(-0.707106781186547,-0.707106781186548,0.));
#31768=DIRECTION('',(0.707106781186547,0.707106781186548,0.));
#31769=DIRECTION('',(0.,0.,1.));
#31770=DIRECTION('',(-0.707106781186547,-0.707106781186548,0.));
#31771=DIRECTION('center_axis',(0.,0.,1.));
#31772=DIRECTION('ref_axis',(1.,0.,0.));
#31773=DIRECTION('',(1.,0.,0.));
#31774=DIRECTION('',(1.,-4.33680868994201E-15,0.));
#31775=DIRECTION('',(0.78801075360672,0.61566147532566,0.));
#31776=DIRECTION('center_axis',(0.61566147532566,-0.788010753606721,0.));
#31777=DIRECTION('ref_axis',(0.78801075360672,0.61566147532566,0.));
#31778=DIRECTION('center_axis',(0.615661475325666,-0.788010753606716,-4.56861825309369E-15));
#31779=DIRECTION('ref_axis',(0.788010753606716,0.615661475325665,-3.955354877202E-13));
#31780=DIRECTION('',(0.,0.,1.));
#31781=DIRECTION('center_axis',(3.7386281809845E-17,4.26676715361993E-32,
-1.));
#31782=DIRECTION('ref_axis',(-1.,4.36567830323557E-65,-3.7386281809845E-17));
#31783=DIRECTION('',(1.,0.,0.));
#31784=DIRECTION('',(0.707106781186546,0.707106781186549,0.));
#31785=DIRECTION('center_axis',(0.,0.,1.));
#31786=DIRECTION('ref_axis',(1.,0.,0.));
#31787=DIRECTION('',(0.,1.,0.));
#31788=DIRECTION('center_axis',(0.,0.,1.));
#31789=DIRECTION('ref_axis',(1.,0.,0.));
#31790=DIRECTION('',(-0.707106781186549,0.707106781186546,0.));
#31791=DIRECTION('center_axis',(0.,0.,-1.));
#31792=DIRECTION('ref_axis',(1.,0.,0.));
#31793=DIRECTION('center_axis',(0.,0.,1.));
#31794=DIRECTION('ref_axis',(1.,0.,0.));
#31795=DIRECTION('center_axis',(0.,0.,-1.));
#31796=DIRECTION('ref_axis',(1.,0.,0.));
#31797=DIRECTION('',(-0.707106781186548,0.707106781186547,0.));
#31798=DIRECTION('center_axis',(0.,0.,-1.));
#31799=DIRECTION('ref_axis',(1.,0.,0.));
#31800=DIRECTION('',(0.,1.,0.));
#31801=DIRECTION('center_axis',(0.,0.,-1.));
#31802=DIRECTION('ref_axis',(1.,0.,0.));
#31803=DIRECTION('',(0.707106781186545,0.70710678118655,0.));
#31804=DIRECTION('center_axis',(0.,0.,-1.));
#31805=DIRECTION('ref_axis',(1.,0.,0.));
#31806=DIRECTION('center_axis',(0.,0.,1.));
#31807=DIRECTION('ref_axis',(1.,0.,0.));
#31808=DIRECTION('center_axis',(0.,0.,-1.));
#31809=DIRECTION('ref_axis',(1.,0.,0.));
#31810=DIRECTION('',(0.707106781186546,0.707106781186549,0.));
#31811=DIRECTION('',(1.,1.22464679914735E-16,0.));
#31812=DIRECTION('',(0.707106781186546,-0.707106781186549,0.));
#31813=DIRECTION('center_axis',(0.,0.,-1.));
#31814=DIRECTION('ref_axis',(1.,0.,0.));
#31815=DIRECTION('center_axis',(0.,0.,1.));
#31816=DIRECTION('ref_axis',(1.,0.,0.));
#31817=DIRECTION('center_axis',(0.,0.,-1.));
#31818=DIRECTION('ref_axis',(1.,0.,0.));
#31819=DIRECTION('',(0.707106781186545,-0.70710678118655,0.));
#31820=DIRECTION('center_axis',(0.,0.,-1.));
#31821=DIRECTION('ref_axis',(1.,0.,0.));
#31822=DIRECTION('',(0.,-1.,0.));
#31823=DIRECTION('center_axis',(0.,0.,-1.));
#31824=DIRECTION('ref_axis',(1.,0.,0.));
#31825=DIRECTION('',(-0.707106781186548,-0.707106781186547,0.));
#31826=DIRECTION('center_axis',(0.,0.,-1.));
#31827=DIRECTION('ref_axis',(1.,0.,0.));
#31828=DIRECTION('center_axis',(0.,0.,1.));
#31829=DIRECTION('ref_axis',(1.,0.,0.));
#31830=DIRECTION('center_axis',(0.,0.,-1.));
#31831=DIRECTION('ref_axis',(1.,0.,0.));
#31832=DIRECTION('',(-0.707106781186549,-0.707106781186546,0.));
#31833=DIRECTION('center_axis',(0.,0.,1.));
#31834=DIRECTION('ref_axis',(1.,0.,0.));
#31835=DIRECTION('',(0.,-1.,0.));
#31836=DIRECTION('center_axis',(0.,0.,1.));
#31837=DIRECTION('ref_axis',(1.,0.,0.));
#31838=DIRECTION('',(0.707106781186546,-0.707106781186549,0.));
#31839=DIRECTION('',(1.,-3.50803534070133E-16,0.));
#31840=DIRECTION('center_axis',(0.,0.,-1.));
#31841=DIRECTION('ref_axis',(-1.,0.,0.));
#31842=DIRECTION('',(1.,-4.33680868994201E-15,0.));
#31843=DIRECTION('',(-0.707106781186547,-0.707106781186548,0.));
#31844=DIRECTION('',(-1.26161707343768E-16,-1.,0.));
#31845=DIRECTION('',(0.707106781186562,-0.707106781186533,0.));
#31846=DIRECTION('',(1.,0.,0.));
#31847=DIRECTION('',(-0.707106781186548,0.707106781186547,0.));
#31848=DIRECTION('',(1.,1.19636101791504E-15,0.));
#31849=DIRECTION('',(-0.707106781186541,-0.707106781186554,0.));
#31850=DIRECTION('',(1.,0.,0.));
#31851=DIRECTION('',(0.707106781186562,0.707106781186533,0.));
#31852=DIRECTION('',(-1.26161707343768E-16,1.,0.));
#31853=DIRECTION('',(-0.707106781186547,0.707106781186548,0.));
#31854=DIRECTION('',(1.,0.,0.));
#31855=DIRECTION('center_axis',(-0.707106781186554,0.707106781186542,1.85853747476774E-16));
#31856=DIRECTION('ref_axis',(-2.62836890299516E-16,1.6519124519235E-33,
-1.));
#31857=DIRECTION('',(0.707106781186541,0.707106781186554,0.));
#31858=DIRECTION('',(2.62836890299516E-16,0.,1.));
#31859=DIRECTION('',(2.62836890299516E-16,0.,1.));
#31860=DIRECTION('center_axis',(-0.707106781186533,-0.707106781186562,0.));
#31861=DIRECTION('ref_axis',(0.707106781186562,-0.707106781186533,0.));
#31862=DIRECTION('',(-0.707106781186562,0.707106781186533,0.));
#31863=DIRECTION('',(0.,0.,1.));
#31864=DIRECTION('',(0.,0.,1.));
#31865=DIRECTION('center_axis',(-1.,1.26161707343768E-16,0.));
#31866=DIRECTION('ref_axis',(-1.26161707343768E-16,-1.,0.));
#31867=DIRECTION('',(1.26161707343768E-16,1.,0.));
#31868=DIRECTION('',(0.,0.,1.));
#31869=DIRECTION('center_axis',(-0.707106781186548,0.707106781186547,0.));
#31870=DIRECTION('ref_axis',(-0.707106781186547,-0.707106781186548,0.));
#31871=DIRECTION('',(0.707106781186547,0.707106781186548,0.));
#31872=DIRECTION('',(0.,0.,1.));
#31873=DIRECTION('center_axis',(0.,-1.,0.));
#31874=DIRECTION('ref_axis',(0.,0.,-1.));
#31875=DIRECTION('',(-1.,0.,0.));
#31876=DIRECTION('',(2.62836890299516E-16,0.,-1.));
#31877=DIRECTION('center_axis',(0.,0.,1.));
#31878=DIRECTION('ref_axis',(1.,0.,0.));
#31879=DIRECTION('',(0.,0.,1.));
#31880=DIRECTION('center_axis',(0.,0.,1.));
#31881=DIRECTION('ref_axis',(1.,0.,0.));
#31882=DIRECTION('',(0.,0.,-1.));
#31883=DIRECTION('center_axis',(0.,0.,1.));
#31884=DIRECTION('ref_axis',(1.,0.,0.));
#31885=DIRECTION('',(0.,0.,1.));
#31886=DIRECTION('center_axis',(0.,0.,1.));
#31887=DIRECTION('ref_axis',(1.,0.,0.));
#31888=DIRECTION('',(0.,0.,-1.));
#31889=DIRECTION('center_axis',(-1.,0.,0.));
#31890=DIRECTION('ref_axis',(0.,0.,1.));
#31891=DIRECTION('',(0.,-1.,0.));
#31892=DIRECTION('center_axis',(-0.707106781186549,-0.707106781186546,0.));
#31893=DIRECTION('ref_axis',(0.707106781186546,-0.707106781186549,0.));
#31894=DIRECTION('',(0.707106781186546,-0.707106781186549,0.));
#31895=DIRECTION('',(0.,0.,1.));
#31896=DIRECTION('center_axis',(-6.49101394191508E-16,-1.,0.));
#31897=DIRECTION('ref_axis',(1.,-6.49101394191508E-16,0.));
#31898=DIRECTION('',(1.,-3.50803534070133E-16,0.));
#31899=DIRECTION('center_axis',(0.,0.,1.));
#31900=DIRECTION('ref_axis',(1.,0.,0.));
#31901=DIRECTION('center_axis',(0.,0.,-1.));
#31902=DIRECTION('ref_axis',(1.,0.,0.));
#31903=DIRECTION('',(0.,0.,-1.));
#31904=DIRECTION('',(0.,0.,1.));
#31905=DIRECTION('center_axis',(0.,0.,1.));
#31906=DIRECTION('ref_axis',(1.,0.,0.));
#31907=DIRECTION('center_axis',(0.,0.,-1.));
#31908=DIRECTION('ref_axis',(1.,0.,0.));
#31909=DIRECTION('',(0.,0.,-1.));
#31910=DIRECTION('',(0.,0.,1.));
#31911=DIRECTION('center_axis',(0.,0.,1.));
#31912=DIRECTION('ref_axis',(1.,0.,0.));
#31913=DIRECTION('center_axis',(0.,0.,1.));
#31914=DIRECTION('ref_axis',(1.,0.,0.));
#31915=DIRECTION('center_axis',(0.,0.,-1.));
#31916=DIRECTION('ref_axis',(-1.,0.,0.));
#31917=DIRECTION('center_axis',(0.,0.,-1.));
#31918=DIRECTION('ref_axis',(1.,0.,0.));
#31919=DIRECTION('',(0.,0.,-1.));
#31920=DIRECTION('',(0.,0.,1.));
#31921=DIRECTION('center_axis',(0.,0.,-1.));
#31922=DIRECTION('ref_axis',(-1.,0.,0.));
#31923=DIRECTION('center_axis',(0.,0.,-1.));
#31924=DIRECTION('ref_axis',(1.,0.,0.));
#31925=DIRECTION('',(0.,0.,-1.));
#31926=DIRECTION('',(0.,0.,1.));
#31927=DIRECTION('center_axis',(-1.,0.,0.));
#31928=DIRECTION('ref_axis',(0.,0.,1.));
#31929=DIRECTION('',(0.,-1.,0.));
#31930=DIRECTION('center_axis',(-0.707106781186546,0.707106781186549,0.));
#31931=DIRECTION('ref_axis',(-0.707106781186549,-0.707106781186546,0.));
#31932=DIRECTION('',(-0.707106781186548,-0.707106781186547,0.));
#31933=DIRECTION('center_axis',(0.,0.,1.));
#31934=DIRECTION('ref_axis',(1.,0.,0.));
#31935=DIRECTION('center_axis',(0.,0.,-1.));
#31936=DIRECTION('ref_axis',(1.,0.,0.));
#31937=DIRECTION('',(0.,0.,-1.));
#31938=DIRECTION('',(0.,0.,1.));
#31939=DIRECTION('center_axis',(0.,0.,1.));
#31940=DIRECTION('ref_axis',(1.,0.,0.));
#31941=DIRECTION('center_axis',(0.,0.,-1.));
#31942=DIRECTION('ref_axis',(1.,0.,0.));
#31943=DIRECTION('',(0.,0.,-1.));
#31944=DIRECTION('',(0.,0.,1.));
#31945=DIRECTION('center_axis',(0.,0.,1.));
#31946=DIRECTION('ref_axis',(1.,0.,0.));
#31947=DIRECTION('center_axis',(0.,0.,1.));
#31948=DIRECTION('ref_axis',(1.,0.,0.));
#31949=DIRECTION('center_axis',(1.22464679914735E-16,-1.,0.));
#31950=DIRECTION('ref_axis',(1.,1.22464679914735E-16,0.));
#31951=DIRECTION('',(0.,0.,1.));
#31952=DIRECTION('',(1.,1.22464679914735E-16,0.));
#31953=DIRECTION('',(0.,0.,1.));
#31954=DIRECTION('center_axis',(-0.707106781186549,-0.707106781186546,0.));
#31955=DIRECTION('ref_axis',(0.707106781186546,-0.707106781186549,0.));
#31956=DIRECTION('',(0.707106781186546,-0.707106781186549,0.));
#31957=DIRECTION('center_axis',(0.,0.,1.));
#31958=DIRECTION('ref_axis',(1.,0.,0.));
#31959=DIRECTION('center_axis',(0.,0.,-1.));
#31960=DIRECTION('ref_axis',(1.,0.,0.));
#31961=DIRECTION('',(0.,0.,-1.));
#31962=DIRECTION('',(0.,0.,1.));
#31963=DIRECTION('center_axis',(0.,0.,1.));
#31964=DIRECTION('ref_axis',(1.,0.,0.));
#31965=DIRECTION('center_axis',(0.,0.,-1.));
#31966=DIRECTION('ref_axis',(1.,0.,0.));
#31967=DIRECTION('',(0.,0.,-1.));
#31968=DIRECTION('',(0.,0.,1.));
#31969=DIRECTION('center_axis',(0.,0.,1.));
#31970=DIRECTION('ref_axis',(1.,0.,0.));
#31971=DIRECTION('center_axis',(0.,0.,1.));
#31972=DIRECTION('ref_axis',(1.,0.,0.));
#31973=DIRECTION('center_axis',(0.,0.,-1.));
#31974=DIRECTION('ref_axis',(-1.,0.,0.));
#31975=DIRECTION('center_axis',(0.,0.,-1.));
#31976=DIRECTION('ref_axis',(1.,0.,0.));
#31977=DIRECTION('',(0.,0.,-1.));
#31978=DIRECTION('',(0.,0.,1.));
#31979=DIRECTION('center_axis',(0.,0.,-1.));
#31980=DIRECTION('ref_axis',(-1.,0.,0.));
#31981=DIRECTION('center_axis',(0.,0.,-1.));
#31982=DIRECTION('ref_axis',(1.,0.,0.));
#31983=DIRECTION('',(0.,0.,-1.));
#31984=DIRECTION('',(0.,0.,1.));
#31985=DIRECTION('center_axis',(1.,0.,0.));
#31986=DIRECTION('ref_axis',(0.,0.,-1.));
#31987=DIRECTION('',(0.,1.,0.));
#31988=DIRECTION('center_axis',(0.707106781186549,-0.707106781186546,0.));
#31989=DIRECTION('ref_axis',(0.707106781186546,0.707106781186549,0.));
#31990=DIRECTION('',(0.707106781186545,0.70710678118655,0.));
#31991=DIRECTION('center_axis',(0.707106781186549,-0.707106781186546,0.));
#31992=DIRECTION('ref_axis',(0.707106781186546,0.707106781186549,0.));
#31993=DIRECTION('',(0.707106781186546,0.707106781186549,0.));
#31994=DIRECTION('center_axis',(0.,0.,1.));
#31995=DIRECTION('ref_axis',(1.,0.,0.));
#31996=DIRECTION('center_axis',(0.,0.,-1.));
#31997=DIRECTION('ref_axis',(1.,0.,0.));
#31998=DIRECTION('',(0.,0.,-1.));
#31999=DIRECTION('',(0.,0.,1.));
#32000=DIRECTION('center_axis',(0.,0.,1.));
#32001=DIRECTION('ref_axis',(1.,0.,0.));
#32002=DIRECTION('center_axis',(0.,0.,-1.));
#32003=DIRECTION('ref_axis',(1.,0.,0.));
#32004=DIRECTION('',(0.,0.,-1.));
#32005=DIRECTION('',(0.,0.,1.));
#32006=DIRECTION('center_axis',(0.,0.,1.));
#32007=DIRECTION('ref_axis',(1.,0.,0.));
#32008=DIRECTION('center_axis',(0.,0.,1.));
#32009=DIRECTION('ref_axis',(1.,0.,0.));
#32010=DIRECTION('center_axis',(0.,0.,1.));
#32011=DIRECTION('ref_axis',(1.,0.,0.));
#32012=DIRECTION('',(0.,0.,1.));
#32013=DIRECTION('center_axis',(0.,0.,1.));
#32014=DIRECTION('ref_axis',(1.,0.,0.));
#32015=DIRECTION('',(0.,0.,-1.));
#32016=DIRECTION('center_axis',(0.,0.,1.));
#32017=DIRECTION('ref_axis',(1.,0.,0.));
#32018=DIRECTION('',(0.,0.,1.));
#32019=DIRECTION('center_axis',(0.,0.,1.));
#32020=DIRECTION('ref_axis',(1.,0.,0.));
#32021=DIRECTION('',(0.,0.,-1.));
#32022=DIRECTION('center_axis',(0.707106781186548,0.707106781186547,0.));
#32023=DIRECTION('ref_axis',(-0.707106781186547,0.707106781186548,0.));
#32024=DIRECTION('',(0.707106781186547,-0.707106781186548,0.));
#32025=DIRECTION('',(0.,0.,1.));
#32026=DIRECTION('',(0.,0.,1.));
#32027=DIRECTION('center_axis',(1.,1.26161707343768E-16,0.));
#32028=DIRECTION('ref_axis',(-1.26161707343768E-16,1.,0.));
#32029=DIRECTION('',(1.26161707343768E-16,-1.,0.));
#32030=DIRECTION('',(0.,0.,1.));
#32031=DIRECTION('center_axis',(0.707106781186533,-0.707106781186562,0.));
#32032=DIRECTION('ref_axis',(0.707106781186562,0.707106781186533,0.));
#32033=DIRECTION('',(-0.707106781186562,-0.707106781186533,0.));
#32034=DIRECTION('',(0.,0.,1.));
#32035=DIRECTION('center_axis',(0.,-1.,0.));
#32036=DIRECTION('ref_axis',(0.,0.,-1.));
#32037=DIRECTION('',(-1.,0.,0.));
#32038=DIRECTION('center_axis',(0.,-1.,0.));
#32039=DIRECTION('ref_axis',(0.,0.,-1.));
#32040=DIRECTION('',(1.,0.,0.));
#32041=DIRECTION('',(0.,0.,1.));
#32042=DIRECTION('center_axis',(0.707106781186549,-0.707106781186546,0.));
#32043=DIRECTION('ref_axis',(0.707106781186546,0.707106781186549,0.));
#32044=DIRECTION('',(0.707106781186546,0.707106781186549,0.));
#32045=DIRECTION('center_axis',(1.,0.,0.));
#32046=DIRECTION('ref_axis',(0.,0.,-1.));
#32047=DIRECTION('',(0.,1.,0.));
#32048=DIRECTION('center_axis',(0.707106781186546,0.707106781186549,0.));
#32049=DIRECTION('ref_axis',(-0.707106781186549,0.707106781186546,0.));
#32050=DIRECTION('',(-0.707106781186549,0.707106781186546,0.));
#32051=DIRECTION('center_axis',(0.707106781186546,0.707106781186549,0.));
#32052=DIRECTION('ref_axis',(-0.707106781186549,0.707106781186546,0.));
#32053=DIRECTION('',(-0.707106781186548,0.707106781186547,0.));
#32054=DIRECTION('center_axis',(-0.707106781186549,-0.707106781186546,0.));
#32055=DIRECTION('ref_axis',(0.707106781186546,-0.707106781186549,0.));
#32056=DIRECTION('',(0.707106781186545,-0.70710678118655,0.));
#32057=DIRECTION('center_axis',(-0.707106781186546,0.707106781186549,0.));
#32058=DIRECTION('ref_axis',(-0.707106781186549,-0.707106781186546,0.));
#32059=DIRECTION('',(-0.707106781186549,-0.707106781186546,0.));
#32060=DIRECTION('center_axis',(0.707106781186547,0.707106781186548,1.85853747476773E-16));
#32061=DIRECTION('ref_axis',(-2.62836890299516E-16,-6.09040047468605E-31,
1.));
#32062=DIRECTION('',(0.707106781186548,-0.707106781186547,0.));
#32063=DIRECTION('',(2.62836890299516E-16,6.28895619248706E-31,-1.));
#32064=DIRECTION('center_axis',(-1.19636101791504E-15,1.,3.14447809624353E-31));
#32065=DIRECTION('ref_axis',(-1.,-1.19636101791504E-15,0.));
#32066=DIRECTION('',(-1.,-1.19636101791504E-15,0.));
#32067=DIRECTION('center_axis',(0.,0.,1.));
#32068=DIRECTION('ref_axis',(1.,0.,0.));
#32069=DIRECTION('center_axis',(1.,1.73472347597681E-16,0.));
#32070=DIRECTION('ref_axis',(-1.73472347597681E-16,1.,0.));
#32071=DIRECTION('',(-1.73472347597681E-16,1.,0.));
#32072=DIRECTION('',(0.,0.,1.));
#32073=DIRECTION('center_axis',(0.,0.,1.));
#32074=DIRECTION('ref_axis',(1.,0.,0.));
#32075=DIRECTION('center_axis',(0.,0.,1.));
#32076=DIRECTION('ref_axis',(1.,0.,0.));
#32077=DIRECTION('',(0.,0.,1.));
#32078=DIRECTION('center_axis',(-1.,1.73472347597681E-16,0.));
#32079=DIRECTION('ref_axis',(-1.73472347597681E-16,-1.,0.));
#32080=DIRECTION('',(-1.73472347597681E-16,-1.,0.));
#32081=DIRECTION('center_axis',(0.,0.,1.));
#32082=DIRECTION('ref_axis',(1.,0.,0.));
#32083=DIRECTION('center_axis',(0.,-1.,0.));
#32084=DIRECTION('ref_axis',(0.,0.,-1.));
#32085=DIRECTION('center_axis',(0.,-1.,0.));
#32086=DIRECTION('ref_axis',(0.,0.,-1.));
#32087=DIRECTION('center_axis',(0.,-1.,0.));
#32088=DIRECTION('ref_axis',(0.,0.,-1.));
#32089=DIRECTION('center_axis',(0.,-1.,0.));
#32090=DIRECTION('ref_axis',(0.,0.,-1.));
#37495=CARTESIAN_POINT('',(0.,0.,0.));
#37496=CARTESIAN_POINT('Origin',(23.2,9.00000000000001,-77.4));
#37497=CARTESIAN_POINT('',(17.28,9.00000000000001,-74.9));
#37498=CARTESIAN_POINT('Origin',(17.28,9.00000000000001,-77.4));
#37499=CARTESIAN_POINT('',(23.2,9.00000000000001,-74.9));
#37500=CARTESIAN_POINT('',(23.2,9.00000000000001,-74.9));
#37501=CARTESIAN_POINT('Origin',(23.2,9.00000000000001,-77.4));
#37502=CARTESIAN_POINT('Origin',(-23.2,9.00000000000001,-77.4));
#37503=CARTESIAN_POINT('',(-17.28,9.00000000000001,-79.9));
#37504=CARTESIAN_POINT('Origin',(-17.28,9.00000000000001,-77.4));
#37505=CARTESIAN_POINT('',(-23.2,9.00000000000001,-79.9));
#37506=CARTESIAN_POINT('',(-23.2,9.00000000000001,-79.9));
#37507=CARTESIAN_POINT('Origin',(-23.2,9.00000000000001,-77.4));
#37508=CARTESIAN_POINT('Origin',(-1.54689479616415E-14,13.,-76.7));
#37509=CARTESIAN_POINT('',(3.64999999999998,13.,-76.7));
#37510=CARTESIAN_POINT('Origin',(-1.54689479616415E-14,13.,-76.7));
#37511=CARTESIAN_POINT('',(3.64999999999998,13.8,-76.7));
#37512=CARTESIAN_POINT('',(3.64999999999998,13.,-76.7));
#37513=CARTESIAN_POINT('Origin',(-1.65097820472275E-14,13.8,-76.7));
#37514=CARTESIAN_POINT('Origin',(17.28,9.00000000000001,-77.4));
#37515=CARTESIAN_POINT('',(15.7778484524311,9.,-77.4));
#37516=CARTESIAN_POINT('',(17.28,9.00000000000001,-74.9));
#37517=CARTESIAN_POINT('Origin',(-17.28,9.00000000000001,-77.4));
#37518=CARTESIAN_POINT('',(-15.7778484524311,9.,-77.4));
#37519=CARTESIAN_POINT('',(-17.28,9.00000000000001,-79.9));
#37520=CARTESIAN_POINT('Origin',(28.5,14.,-64.9));
#37521=CARTESIAN_POINT('',(28.5,0.500000000000005,-68.2235));
#37522=CARTESIAN_POINT('Origin',(28.5,0.500000000000006,-64.9));
#37523=CARTESIAN_POINT('',(28.5,14.,-68.2235));
#37524=CARTESIAN_POINT('',(28.5,14.,-68.2235));
#37525=CARTESIAN_POINT('Origin',(28.5,14.,-64.9));
#37526=CARTESIAN_POINT('Origin',(28.5,14.,-19.9));
#37527=CARTESIAN_POINT('',(28.5,0.500000000000005,-23.2235));
#37528=CARTESIAN_POINT('Origin',(28.5,0.500000000000006,-19.9));
#37529=CARTESIAN_POINT('',(28.5,14.,-23.2235));
#37530=CARTESIAN_POINT('',(28.5,14.,-23.2235));
#37531=CARTESIAN_POINT('Origin',(28.5,14.,-19.9));
#37532=CARTESIAN_POINT('Origin',(-28.5,14.,-64.9));
#37533=CARTESIAN_POINT('',(-28.5,0.500000000000005,-68.2235));
#37534=CARTESIAN_POINT('Origin',(-28.5,0.500000000000006,-64.9));
#37535=CARTESIAN_POINT('',(-28.5,14.,-68.2235));
#37536=CARTESIAN_POINT('',(-28.5,14.,-68.2235));
#37537=CARTESIAN_POINT('Origin',(-28.5,14.,-64.9));
#37538=CARTESIAN_POINT('Origin',(-28.5,14.,-19.9));
#37539=CARTESIAN_POINT('',(-28.5,0.500000000000003,-23.2235));
#37540=CARTESIAN_POINT('Origin',(-28.5,0.500000000000004,-19.9));
#37541=CARTESIAN_POINT('',(-28.5,14.,-23.2235));
#37542=CARTESIAN_POINT('',(-28.5,14.,-23.2235));
#37543=CARTESIAN_POINT('Origin',(-28.5,14.,-19.9));
#37544=CARTESIAN_POINT('Origin',(-23.2,9.00000000000001,-7.4));
#37545=CARTESIAN_POINT('',(-17.28,9.00000000000001,-9.9));
#37546=CARTESIAN_POINT('Origin',(-17.28,9.00000000000001,-7.4));
#37547=CARTESIAN_POINT('',(-23.2,9.00000000000001,-9.9));
#37548=CARTESIAN_POINT('',(-23.2,9.00000000000001,-9.9));
#37549=CARTESIAN_POINT('Origin',(-23.2,9.00000000000001,-7.4));
#37550=CARTESIAN_POINT('Origin',(23.2,9.00000000000001,-7.4));
#37551=CARTESIAN_POINT('',(17.28,9.00000000000001,-4.90000000000001));
#37552=CARTESIAN_POINT('Origin',(17.28,9.00000000000001,-7.4));
#37553=CARTESIAN_POINT('',(23.2,9.00000000000001,-4.90000000000001));
#37554=CARTESIAN_POINT('',(23.2,9.00000000000001,-4.90000000000001));
#37555=CARTESIAN_POINT('Origin',(23.2,9.00000000000001,-7.4));
#37556=CARTESIAN_POINT('Origin',(-1.54689479616415E-14,13.,-8.1));
#37557=CARTESIAN_POINT('',(3.64999999999998,13.,-8.1));
#37558=CARTESIAN_POINT('Origin',(-1.54689479616415E-14,13.,-8.1));
#37559=CARTESIAN_POINT('',(3.64999999999998,13.8,-8.1));
#37560=CARTESIAN_POINT('',(3.64999999999998,13.,-8.1));
#37561=CARTESIAN_POINT('Origin',(-1.65097820472275E-14,13.8,-8.1));
#37562=CARTESIAN_POINT('Origin',(-1.90276438129354E-14,12.7,-74.2));
#37563=CARTESIAN_POINT('',(0.499999999999987,12.5,-74.2));
#37564=CARTESIAN_POINT('Origin',(-1.87674352915389E-14,12.5,-74.2));
#37565=CARTESIAN_POINT('',(0.499999999999987,12.7,-74.2));
#37566=CARTESIAN_POINT('',(0.499999999999987,12.7,-74.2));
#37567=CARTESIAN_POINT('',(-0.500000000000023,12.7,-74.2));
#37568=CARTESIAN_POINT('Origin',(-1.90276438129354E-14,12.7,-74.2));
#37569=CARTESIAN_POINT('',(-0.500000000000025,13.,-74.2));
#37570=CARTESIAN_POINT('',(-0.500000000000025,12.7,-74.2));
#37571=CARTESIAN_POINT('',(0.499999999999986,13.,-74.2));
#37572=CARTESIAN_POINT('Origin',(-1.94179565950302E-14,13.,-74.2));
#37573=CARTESIAN_POINT('',(0.499999999999987,12.7,-74.2));
#37574=CARTESIAN_POINT('Origin',(-17.28,9.00000000000001,-7.4));
#37575=CARTESIAN_POINT('',(-15.7778484524311,9.,-7.4));
#37576=CARTESIAN_POINT('',(-17.28,9.00000000000001,-9.9));
#37577=CARTESIAN_POINT('Origin',(17.28,9.00000000000001,-7.4));
#37578=CARTESIAN_POINT('',(15.7778484524311,9.,-7.4));
#37579=CARTESIAN_POINT('',(17.28,9.00000000000001,-4.90000000000001));
#37580=CARTESIAN_POINT('Origin',(-1.65232411086791E-14,12.7,-10.6));
#37581=CARTESIAN_POINT('',(0.499999999999984,12.5,-10.6));
#37582=CARTESIAN_POINT('Origin',(-1.62630325872826E-14,12.5,-10.6));
#37583=CARTESIAN_POINT('',(0.499999999999984,12.7,-10.6));
#37584=CARTESIAN_POINT('',(0.499999999999984,12.7,-10.6));
#37585=CARTESIAN_POINT('',(0.499999999999983,13.,-10.6));
#37586=CARTESIAN_POINT('',(0.499999999999984,12.7,-10.6));
#37587=CARTESIAN_POINT('',(-0.500000000000017,13.,-10.6));
#37588=CARTESIAN_POINT('Origin',(-1.69135538907739E-14,13.,-10.6));
#37589=CARTESIAN_POINT('',(-0.500000000000017,12.7,-10.6));
#37590=CARTESIAN_POINT('',(-0.500000000000017,12.7,-10.6));
#37591=CARTESIAN_POINT('Origin',(-1.65232411086791E-14,12.7,-10.6));
#37592=CARTESIAN_POINT('Ctrl Pts',(4.,8.,-84.5));
#37593=CARTESIAN_POINT('Ctrl Pts',(4.,4.,-84.5));
#37594=CARTESIAN_POINT('Ctrl Pts',(0.,4.,-84.5));
#37595=CARTESIAN_POINT('Ctrl Pts',(-4.,4.,-84.5));
#37596=CARTESIAN_POINT('Ctrl Pts',(-4.,8.,-84.5));
#37597=CARTESIAN_POINT('Ctrl Pts',(-4.,12.,-84.5));
#37598=CARTESIAN_POINT('Ctrl Pts',(0.,12.,-84.5));
#37599=CARTESIAN_POINT('Ctrl Pts',(4.,12.,-84.5));
#37600=CARTESIAN_POINT('Ctrl Pts',(4.,8.,-84.5));
#37601=CARTESIAN_POINT('Ctrl Pts',(4.,8.,-86.5172334444062));
#37602=CARTESIAN_POINT('Ctrl Pts',(4.,4.,-86.5172334444062));
#37603=CARTESIAN_POINT('Ctrl Pts',(0.,4.,-86.5172334444062));
#37604=CARTESIAN_POINT('Ctrl Pts',(-4.,4.,-86.5172334444062));
#37605=CARTESIAN_POINT('Ctrl Pts',(-4.,8.,-86.5172334444062));
#37606=CARTESIAN_POINT('Ctrl Pts',(-4.,12.,-86.5172334444062));
#37607=CARTESIAN_POINT('Ctrl Pts',(0.,12.,-86.5172334444062));
#37608=CARTESIAN_POINT('Ctrl Pts',(4.,12.,-86.5172334444062));
#37609=CARTESIAN_POINT('Ctrl Pts',(4.,8.,-86.5172334444062));
#37610=CARTESIAN_POINT('Ctrl Pts',(2.,8.,-86.7803508501983));
#37611=CARTESIAN_POINT('Ctrl Pts',(2.,6.,-86.7803508501983));
#37612=CARTESIAN_POINT('Ctrl Pts',(0.,6.,-86.7803508501983));
#37613=CARTESIAN_POINT('Ctrl Pts',(-2.,6.,-86.7803508501983));
#37614=CARTESIAN_POINT('Ctrl Pts',(-2.,8.,-86.7803508501983));
#37615=CARTESIAN_POINT('Ctrl Pts',(-2.,10.,-86.7803508501983));
#37616=CARTESIAN_POINT('Ctrl Pts',(0.,10.,-86.7803508501983));
#37617=CARTESIAN_POINT('Ctrl Pts',(2.,10.,-86.7803508501983));
#37618=CARTESIAN_POINT('Ctrl Pts',(2.,8.,-86.7803508501983));
#37619=CARTESIAN_POINT('',(-1.15470053837925,6.,-86.7177985317981));
#37620=CARTESIAN_POINT('',(-2.3094010767585,8.,-86.7177985317981));
#37621=CARTESIAN_POINT('Ctrl Pts',(-1.15470053837925,6.,-86.7177985317981));
#37622=CARTESIAN_POINT('Ctrl Pts',(-1.16052376017366,6.01008611601166,-86.7193986219689));
#37623=CARTESIAN_POINT('Ctrl Pts',(-1.16635206467311,6.02018103552669,-86.7209572835343));
#37624=CARTESIAN_POINT('Ctrl Pts',(-1.36167110655042,6.35848353974387,-86.7717992509189));
#37625=CARTESIAN_POINT('Ctrl Pts',(-1.5557141858025,6.69457601186558,-86.7803508501983));
#37626=CARTESIAN_POINT('Ctrl Pts',(-1.90838742933526,7.30542398813443,-86.7803508501983));
#37627=CARTESIAN_POINT('Ctrl Pts',(-2.10243050858733,7.64151646025614,-86.7717992509189));
#37628=CARTESIAN_POINT('Ctrl Pts',(-2.29774955046464,7.97981896447331,-86.7209572835343));
#37629=CARTESIAN_POINT('Ctrl Pts',(-2.3035778549641,7.98991388398835,-86.7193986219689));
#37630=CARTESIAN_POINT('Ctrl Pts',(-2.30940107675851,8.00000000000001,-86.7177985317981));
#37631=CARTESIAN_POINT('',(1.15470053837925,6.,-86.7177985317981));
#37632=CARTESIAN_POINT('Ctrl Pts',(1.15470053837925,6.,-86.7177985317981));
#37633=CARTESIAN_POINT('Ctrl Pts',(1.14305409479044,6.,-86.7193986219689));
#37634=CARTESIAN_POINT('Ctrl Pts',(1.13139748579153,6.,-86.7209572835343));
#37635=CARTESIAN_POINT('Ctrl Pts',(0.740759402036912,6.,-86.7717992509189));
#37636=CARTESIAN_POINT('Ctrl Pts',(0.352673243532761,6.,-86.7803508501983));
#37637=CARTESIAN_POINT('Ctrl Pts',(-0.352673243532758,6.,-86.7803508501983));
#37638=CARTESIAN_POINT('Ctrl Pts',(-0.740759402036907,6.,-86.7717992509189));
#37639=CARTESIAN_POINT('Ctrl Pts',(-1.13139748579153,6.,-86.7209572835343));
#37640=CARTESIAN_POINT('Ctrl Pts',(-1.14305409479043,6.,-86.7193986219689));
#37641=CARTESIAN_POINT('Ctrl Pts',(-1.15470053837925,6.,-86.7177985317981));
#37642=CARTESIAN_POINT('',(2.3094010767585,8.,-86.7177985317981));
#37643=CARTESIAN_POINT('Ctrl Pts',(2.3094010767585,8.,-86.7177985317981));
#37644=CARTESIAN_POINT('Ctrl Pts',(2.30357785496409,7.98991388398834,-86.7193986219689));
#37645=CARTESIAN_POINT('Ctrl Pts',(2.29774955046465,7.97981896447331,-86.7209572835343));
#37646=CARTESIAN_POINT('Ctrl Pts',(2.10243050858733,7.64151646025614,-86.7717992509189));
#37647=CARTESIAN_POINT('Ctrl Pts',(1.90838742933526,7.30542398813443,-86.7803508501983));
#37648=CARTESIAN_POINT('Ctrl Pts',(1.5557141858025,6.69457601186558,-86.7803508501983));
#37649=CARTESIAN_POINT('Ctrl Pts',(1.36167110655042,6.35848353974387,-86.7717992509189));
#37650=CARTESIAN_POINT('Ctrl Pts',(1.16635206467311,6.02018103552669,-86.7209572835344));
#37651=CARTESIAN_POINT('Ctrl Pts',(1.16052376017366,6.01008611601166,-86.7193986219689));
#37652=CARTESIAN_POINT('Ctrl Pts',(1.15470053837925,6.00000000000001,-86.7177985317981));
#37653=CARTESIAN_POINT('',(4.,8.,-84.5));
#37654=CARTESIAN_POINT('Ctrl Pts',(2.3094010767585,8.,-86.7177985317981));
#37655=CARTESIAN_POINT('Ctrl Pts',(4.,8.,-86.2532600313803));
#37656=CARTESIAN_POINT('Ctrl Pts',(4.,8.,-84.5));
#37657=CARTESIAN_POINT('',(-4.,8.,-84.5));
#37658=CARTESIAN_POINT('Origin',(0.,8.,-84.5));
#37659=CARTESIAN_POINT('Origin',(0.,8.,-84.5));
#37660=CARTESIAN_POINT('',(1.15470053837925,10.,-86.7177985317981));
#37661=CARTESIAN_POINT('Ctrl Pts',(1.15470053837925,10.,-86.7177985317981));
#37662=CARTESIAN_POINT('Ctrl Pts',(1.16052376017366,9.98991388398835,-86.7193986219689));
#37663=CARTESIAN_POINT('Ctrl Pts',(1.16635206467311,9.97981896447332,-86.7209572835343));
#37664=CARTESIAN_POINT('Ctrl Pts',(1.36167110655042,9.64151646025614,-86.7717992509189));
#37665=CARTESIAN_POINT('Ctrl Pts',(1.5557141858025,9.30542398813443,-86.7803508501983));
#37666=CARTESIAN_POINT('Ctrl Pts',(1.90838742933526,8.69457601186558,-86.7803508501983));
#37667=CARTESIAN_POINT('Ctrl Pts',(2.10243050858733,8.35848353974387,-86.7717992509189));
#37668=CARTESIAN_POINT('Ctrl Pts',(2.29774955046465,8.02018103552669,-86.7209572835343));
#37669=CARTESIAN_POINT('Ctrl Pts',(2.3035778549641,8.01008611601166,-86.7193986219689));
#37670=CARTESIAN_POINT('Ctrl Pts',(2.30940107675851,8.,-86.7177985317981));
#37671=CARTESIAN_POINT('',(-1.15470053837925,10.,-86.7177985317981));
#37672=CARTESIAN_POINT('Ctrl Pts',(-1.15470053837925,10.,-86.7177985317981));
#37673=CARTESIAN_POINT('Ctrl Pts',(-1.14305409479043,10.,-86.7193986219689));
#37674=CARTESIAN_POINT('Ctrl Pts',(-1.13139748579153,10.,-86.7209572835343));
#37675=CARTESIAN_POINT('Ctrl Pts',(-0.740759402036911,10.,-86.7717992509189));
#37676=CARTESIAN_POINT('Ctrl Pts',(-0.352673243532759,10.,-86.7803508501983));
#37677=CARTESIAN_POINT('Ctrl Pts',(0.352673243532759,10.,-86.7803508501983));
#37678=CARTESIAN_POINT('Ctrl Pts',(0.740759402036911,10.,-86.7717992509189));
#37679=CARTESIAN_POINT('Ctrl Pts',(1.13139748579153,10.,-86.7209572835343));
#37680=CARTESIAN_POINT('Ctrl Pts',(1.14305409479044,10.,-86.7193986219689));
#37681=CARTESIAN_POINT('Ctrl Pts',(1.15470053837925,10.,-86.7177985317981));
#37682=CARTESIAN_POINT('Ctrl Pts',(-2.3094010767585,8.,-86.7177985317981));
#37683=CARTESIAN_POINT('Ctrl Pts',(-2.3035778549641,8.01008611601166,-86.7193986219689));
#37684=CARTESIAN_POINT('Ctrl Pts',(-2.29774955046464,8.02018103552669,-86.7209572835343));
#37685=CARTESIAN_POINT('Ctrl Pts',(-2.10243050858733,8.35848353974387,-86.7717992509189));
#37686=CARTESIAN_POINT('Ctrl Pts',(-1.90838742933526,8.69457601186558,-86.7803508501983));
#37687=CARTESIAN_POINT('Ctrl Pts',(-1.5557141858025,9.30542398813443,-86.7803508501983));
#37688=CARTESIAN_POINT('Ctrl Pts',(-1.36167110655042,9.64151646025614,-86.7717992509189));
#37689=CARTESIAN_POINT('Ctrl Pts',(-1.16635206467311,9.97981896447332,-86.7209572835343));
#37690=CARTESIAN_POINT('Ctrl Pts',(-1.16052376017366,9.98991388398835,-86.7193986219689));
#37691=CARTESIAN_POINT('Ctrl Pts',(-1.15470053837925,10.,-86.7177985317981));
#37692=CARTESIAN_POINT('Origin',(0.,8.,-86.8));
#37693=CARTESIAN_POINT('',(-4.,8.,-83.8));
#37694=CARTESIAN_POINT('Origin',(0.,8.,-83.8));
#37695=CARTESIAN_POINT('',(-4.,8.,-86.8));
#37696=CARTESIAN_POINT('Origin',(0.,8.,-83.8));
#37697=CARTESIAN_POINT('',(4.99995,8.,-83.8));
#37698=CARTESIAN_POINT('Origin',(0.,8.,-83.8));
#37699=CARTESIAN_POINT('',(4.99995,8.,-84.8));
#37700=CARTESIAN_POINT('',(4.99995,8.,-83.8));
#37701=CARTESIAN_POINT('Origin',(0.,8.,-84.8));
#37702=CARTESIAN_POINT('Origin',(25.4958861827765,-14.55,-104.175753233145));
#37703=CARTESIAN_POINT('',(23.,-16.5,-64.9));
#37704=CARTESIAN_POINT('',(25.4958861827765,-14.55,-69.5070923773207));
#37705=CARTESIAN_POINT('Origin',(28.4999999999971,-12.2029290542153,-64.9000000000014));
#37706=CARTESIAN_POINT('',(23.,-16.5,-71.4));
#37707=CARTESIAN_POINT('',(23.,-16.5,-84.8));
#37708=CARTESIAN_POINT('',(25.4958861827765,-14.55,-71.4));
#37709=CARTESIAN_POINT('',(25.4958861827765,-14.55,-71.4));
#37710=CARTESIAN_POINT('',(25.4958861827765,-14.55,-104.175753233145));
#37711=CARTESIAN_POINT('Origin',(25.4958861827765,-14.55,-104.175753233145));
#37712=CARTESIAN_POINT('',(25.4958861827765,-14.55,-60.2929076226793));
#37713=CARTESIAN_POINT('Origin',(28.5000000000002,-12.2029290542129,-64.9000000000003));
#37714=CARTESIAN_POINT('',(25.4958861827765,-14.55,-24.5070923773207));
#37715=CARTESIAN_POINT('',(25.4958861827765,-14.55,-104.175753233145));
#37716=CARTESIAN_POINT('',(23.,-16.5,-19.9));
#37717=CARTESIAN_POINT('Origin',(28.4999999999964,-12.2029290542158,-19.900000000002));
#37718=CARTESIAN_POINT('',(23.,-16.5,-84.8));
#37719=CARTESIAN_POINT('Origin',(-25.4958861827765,-14.55,-104.175753233145));
#37720=CARTESIAN_POINT('',(-23.,-16.5,-64.9));
#37721=CARTESIAN_POINT('',(-25.4958861827765,-14.55,-60.2929076226793));
#37722=CARTESIAN_POINT('Origin',(-28.5000000000003,-12.2029290542127,-64.9000000000003));
#37723=CARTESIAN_POINT('',(-23.,-16.5,-19.9));
#37724=CARTESIAN_POINT('',(-23.,-16.5,-84.8));
#37725=CARTESIAN_POINT('',(-25.4958861827765,-14.55,-24.5070923773207));
#37726=CARTESIAN_POINT('Origin',(-28.4999999999988,-12.2029290542139,-19.9000000000006));
#37727=CARTESIAN_POINT('',(-25.4958861827765,-14.55,-104.175753233145));
#37728=CARTESIAN_POINT('Origin',(-25.4958861827765,-14.55,-104.175753233145));
#37729=CARTESIAN_POINT('',(-25.4958861827765,-14.55,-15.2929076226793));
#37730=CARTESIAN_POINT('Origin',(-28.4999999999998,-12.2029290542132,-19.8999999999999));
#37731=CARTESIAN_POINT('',(-23.,-16.5,-13.4));
#37732=CARTESIAN_POINT('',(-23.,-16.5,-84.8));
#37733=CARTESIAN_POINT('',(-25.4958861827765,-14.55,-13.4));
#37734=CARTESIAN_POINT('',(-25.4958861827765,-14.55,-13.4));
#37735=CARTESIAN_POINT('',(-25.4958861827765,-14.55,-104.175753233145));
#37736=CARTESIAN_POINT('Origin',(8.05,-8.2,-84.8));
#37737=CARTESIAN_POINT('',(8.57259699813413,-7.67740300186587,-81.35));
#37738=CARTESIAN_POINT('',(8.19644660940673,-8.05355339059327,-81.35));
#37739=CARTESIAN_POINT('',(8.57259699813413,-7.67740300186587,-81.35));
#37740=CARTESIAN_POINT('',(8.57259699813413,-7.67740300186587,-84.8));
#37741=CARTESIAN_POINT('',(8.57259699813413,-7.67740300186587,-84.8));
#37742=CARTESIAN_POINT('',(8.19644660940673,-8.05355339059327,-84.8));
#37743=CARTESIAN_POINT('',(8.05,-8.2,-84.8));
#37744=CARTESIAN_POINT('',(8.19644660940673,-8.05355339059327,-84.8));
#37745=CARTESIAN_POINT('Origin',(8.05,3.67394039744206E-16,-84.8));
#37746=CARTESIAN_POINT('',(10.9824030018659,-2.93240300186586,-81.35));
#37747=CARTESIAN_POINT('',(11.3535533905933,-3.30355339059329,-81.35));
#37748=CARTESIAN_POINT('',(10.9824030018659,-2.93240300186586,-81.35));
#37749=CARTESIAN_POINT('',(10.9824030018659,-2.93240300186586,-84.8));
#37750=CARTESIAN_POINT('',(10.9824030018659,-2.93240300186586,-84.8));
#37751=CARTESIAN_POINT('',(11.3535533905933,-3.30355339059329,-84.8));
#37752=CARTESIAN_POINT('',(8.05,3.67394039744206E-16,-84.8));
#37753=CARTESIAN_POINT('',(11.3535533905933,-3.30355339059329,0.));
#37754=CARTESIAN_POINT('Origin',(-8.05,-8.2,-84.8));
#37755=CARTESIAN_POINT('',(-10.9824030018659,-5.26759699813413,-81.35));
#37756=CARTESIAN_POINT('',(-11.3535533905933,-4.89644660940674,-81.35));
#37757=CARTESIAN_POINT('',(-10.9824030018659,-5.26759699813413,-81.35));
#37758=CARTESIAN_POINT('',(-10.9824030018659,-5.26759699813413,-84.8));
#37759=CARTESIAN_POINT('',(-10.9824030018659,-5.26759699813413,-84.8));
#37760=CARTESIAN_POINT('',(-11.3535533905933,-4.89644660940674,-84.8));
#37761=CARTESIAN_POINT('',(-8.05,-8.2,-84.8));
#37762=CARTESIAN_POINT('',(-11.3535533905933,-4.89644660940674,0.));
#37763=CARTESIAN_POINT('Origin',(-8.05,-1.60428730688303E-15,-84.8));
#37764=CARTESIAN_POINT('',(-8.57259699813413,-0.522596998134137,-81.35));
#37765=CARTESIAN_POINT('',(-8.05,-1.60428730688303E-15,-81.35));
#37766=CARTESIAN_POINT('',(-8.57259699813413,-0.522596998134137,-81.35));
#37767=CARTESIAN_POINT('',(-8.57259699813413,-0.522596998134137,-84.8));
#37768=CARTESIAN_POINT('',(-8.57259699813413,-0.522596998134137,-84.8));
#37769=CARTESIAN_POINT('',(-8.05,-1.60428730688303E-15,-84.8));
#37770=CARTESIAN_POINT('',(-8.05,-1.60428730688303E-15,-84.8));
#37771=CARTESIAN_POINT('',(-8.05,-1.60428730688303E-15,-84.8));
#37772=CARTESIAN_POINT('Origin',(-8.05,-1.60428730688303E-15,-84.8));
#37773=CARTESIAN_POINT('',(-11.3535533905933,-3.30355339059329,-81.35));
#37774=CARTESIAN_POINT('',(-10.9824030018659,-2.93240300186587,-81.35));
#37775=CARTESIAN_POINT('',(-11.3535533905933,-3.30355339059329,-81.35));
#37776=CARTESIAN_POINT('',(-11.3535533905933,-3.30355339059329,-84.8));
#37777=CARTESIAN_POINT('',(-11.3535533905933,-3.30355339059329,-84.8));
#37778=CARTESIAN_POINT('',(-10.9824030018659,-2.93240300186587,-84.8));
#37779=CARTESIAN_POINT('',(-8.05,-1.60428730688303E-15,-84.8));
#37780=CARTESIAN_POINT('',(-10.9824030018659,-2.93240300186587,0.));
#37781=CARTESIAN_POINT('Origin',(-11.5,-4.75000000000001,-84.8));
#37782=CARTESIAN_POINT('',(-11.5,-4.54289321881346,-81.35));
#37783=CARTESIAN_POINT('',(-11.5,-3.65710678118656,-81.35));
#37784=CARTESIAN_POINT('',(-11.5,-4.54289321881346,-81.35));
#37785=CARTESIAN_POINT('',(-11.5,-4.54289321881346,-84.8));
#37786=CARTESIAN_POINT('',(-11.5,-4.54289321881346,-84.8));
#37787=CARTESIAN_POINT('',(-11.5,-3.65710678118656,-84.8));
#37788=CARTESIAN_POINT('',(-11.5,-4.75000000000001,-84.8));
#37789=CARTESIAN_POINT('',(-11.5,-3.65710678118656,0.));
#37790=CARTESIAN_POINT('Origin',(-8.05,-8.2,-84.8));
#37791=CARTESIAN_POINT('',(-8.19644660940673,-8.05355339059327,-81.35));
#37792=CARTESIAN_POINT('',(-8.57259699813413,-7.67740300186587,-81.35));
#37793=CARTESIAN_POINT('',(-8.19644660940673,-8.05355339059327,-81.35));
#37794=CARTESIAN_POINT('',(-8.19644660940673,-8.05355339059327,-84.8));
#37795=CARTESIAN_POINT('',(-8.19644660940673,-8.05355339059327,-84.8));
#37796=CARTESIAN_POINT('',(-8.57259699813413,-7.67740300186587,-84.8));
#37797=CARTESIAN_POINT('',(-8.05,-8.2,-84.8));
#37798=CARTESIAN_POINT('',(-8.57259699813413,-7.67740300186587,0.));
#37799=CARTESIAN_POINT('Origin',(-8.05,-12.24,-84.8));
#37800=CARTESIAN_POINT('',(-8.05,-12.0328932188134,-81.35));
#37801=CARTESIAN_POINT('',(-8.05,-8.40710678118654,-81.35));
#37802=CARTESIAN_POINT('',(-8.05,-12.0328932188134,-81.35));
#37803=CARTESIAN_POINT('',(-8.05,-12.0328932188134,-84.8));
#37804=CARTESIAN_POINT('',(-8.05,-12.0328932188134,-84.8));
#37805=CARTESIAN_POINT('',(-8.05,-8.40710678118654,-84.8));
#37806=CARTESIAN_POINT('',(-8.05,-12.24,-84.8));
#37807=CARTESIAN_POINT('',(-8.05,-8.40710678118654,-84.8));
#37808=CARTESIAN_POINT('Origin',(-12.31,-16.5,-84.8));
#37809=CARTESIAN_POINT('',(-12.31,-16.5,-81.35));
#37810=CARTESIAN_POINT('',(-8.19644660940672,-12.3864466094067,-81.35));
#37811=CARTESIAN_POINT('',(-12.31,-16.5,-81.35));
#37812=CARTESIAN_POINT('',(-12.31,-16.5,-84.8));
#37813=CARTESIAN_POINT('',(-12.31,-16.5,-84.8));
#37814=CARTESIAN_POINT('',(-8.19644660940672,-12.3864466094067,-84.8));
#37815=CARTESIAN_POINT('',(-12.31,-16.5,-84.8));
#37816=CARTESIAN_POINT('',(-8.19644660940672,-12.3864466094067,-84.8));
#37817=CARTESIAN_POINT('Origin',(-23.,-16.5,-84.8));
#37818=CARTESIAN_POINT('',(-22.2,-16.5,-81.35));
#37819=CARTESIAN_POINT('',(-22.2,-16.5,-81.35));
#37820=CARTESIAN_POINT('',(-22.2,-16.5,-84.8));
#37821=CARTESIAN_POINT('',(-22.2,-16.5,-84.8));
#37822=CARTESIAN_POINT('',(-23.,-16.5,-84.8));
#37823=CARTESIAN_POINT('Origin',(12.31,-16.5,-84.8));
#37824=CARTESIAN_POINT('',(12.31,-16.5,-81.35));
#37825=CARTESIAN_POINT('',(22.2,-16.5,-81.35));
#37826=CARTESIAN_POINT('',(12.31,-16.5,-81.35));
#37827=CARTESIAN_POINT('',(12.31,-16.5,-84.8));
#37828=CARTESIAN_POINT('',(12.31,-16.5,-84.8));
#37829=CARTESIAN_POINT('',(22.2,-16.5,-84.8));
#37830=CARTESIAN_POINT('',(12.31,-16.5,-84.8));
#37831=CARTESIAN_POINT('',(22.2,-16.5,-84.8));
#37832=CARTESIAN_POINT('Origin',(12.31,-16.5,-84.8));
#37833=CARTESIAN_POINT('',(8.19644660940673,-12.3864466094067,-81.35));
#37834=CARTESIAN_POINT('',(8.19644660940673,-12.3864466094067,-81.35));
#37835=CARTESIAN_POINT('',(8.19644660940673,-12.3864466094067,-84.8));
#37836=CARTESIAN_POINT('',(8.19644660940673,-12.3864466094067,-84.8));
#37837=CARTESIAN_POINT('',(12.31,-16.5,-84.8));
#37838=CARTESIAN_POINT('Origin',(8.05,-12.24,-84.8));
#37839=CARTESIAN_POINT('',(8.05,-8.40710678118654,-81.35));
#37840=CARTESIAN_POINT('',(8.05,-12.0328932188134,-81.35));
#37841=CARTESIAN_POINT('',(8.05,-8.40710678118654,-81.35));
#37842=CARTESIAN_POINT('',(8.05,-8.40710678118654,-84.8));
#37843=CARTESIAN_POINT('',(8.05,-8.40710678118654,-84.8));
#37844=CARTESIAN_POINT('',(8.05,-12.0328932188134,-84.8));
#37845=CARTESIAN_POINT('',(8.05,-12.24,-84.8));
#37846=CARTESIAN_POINT('',(8.05,-12.0328932188134,-84.8));
#37847=CARTESIAN_POINT('Origin',(8.05,-8.2,-84.8));
#37848=CARTESIAN_POINT('',(11.3535533905933,-4.89644660940673,-81.35));
#37849=CARTESIAN_POINT('',(10.9824030018659,-5.26759699813413,-81.35));
#37850=CARTESIAN_POINT('',(11.3535533905933,-4.89644660940673,-81.35));
#37851=CARTESIAN_POINT('',(11.3535533905933,-4.89644660940673,-84.8));
#37852=CARTESIAN_POINT('',(11.3535533905933,-4.89644660940673,-84.8));
#37853=CARTESIAN_POINT('',(10.9824030018659,-5.26759699813413,-84.8));
#37854=CARTESIAN_POINT('',(8.05,-8.2,-84.8));
#37855=CARTESIAN_POINT('',(10.9824030018659,-5.26759699813413,0.));
#37856=CARTESIAN_POINT('Origin',(11.5,-4.75000000000001,-84.8));
#37857=CARTESIAN_POINT('',(11.5,-3.65710678118656,-81.35));
#37858=CARTESIAN_POINT('',(11.5,-4.54289321881346,-81.35));
#37859=CARTESIAN_POINT('',(11.5,-3.65710678118656,-81.35));
#37860=CARTESIAN_POINT('',(11.5,-3.65710678118656,-84.8));
#37861=CARTESIAN_POINT('',(11.5,-3.65710678118656,-84.8));
#37862=CARTESIAN_POINT('',(11.5,-4.54289321881346,-84.8));
#37863=CARTESIAN_POINT('',(11.5,-4.75000000000001,-84.8));
#37864=CARTESIAN_POINT('',(11.5,-4.54289321881346,0.));
#37865=CARTESIAN_POINT('Origin',(8.05,3.67394039744206E-16,-84.8));
#37866=CARTESIAN_POINT('',(8.05,3.67394039744206E-16,-81.35));
#37867=CARTESIAN_POINT('',(8.57259699813413,-0.522596998134133,-81.35));
#37868=CARTESIAN_POINT('',(8.05,3.67394039744206E-16,-81.35));
#37869=CARTESIAN_POINT('',(8.05,3.67394039744206E-16,-84.8));
#37870=CARTESIAN_POINT('',(8.05,3.67394039744206E-16,-84.8));
#37871=CARTESIAN_POINT('',(8.57259699813413,-0.522596998134133,-84.8));
#37872=CARTESIAN_POINT('',(8.05,3.67394039744206E-16,-84.8));
#37873=CARTESIAN_POINT('',(8.57259699813413,-0.522596998134133,0.));
#37874=CARTESIAN_POINT('Origin',(8.05,3.67394039744206E-16,-84.8));
#37875=CARTESIAN_POINT('',(-8.05,-1.60428730688303E-15,-81.35));
#37876=CARTESIAN_POINT('',(8.05,3.67394039744206E-16,-84.8));
#37877=CARTESIAN_POINT('Origin',(-10.995,-0.510000000000002,-84.8));
#37878=CARTESIAN_POINT('',(-10.6942336092596,-2.79024989380572,-81.35));
#37879=CARTESIAN_POINT('',(-8.71475010619428,-0.810766390740372,-81.35));
#37880=CARTESIAN_POINT('Origin',(-10.995,-0.510000000000002,-81.35));
#37881=CARTESIAN_POINT('',(-10.6942336092596,-2.79024989380572,-84.8));
#37882=CARTESIAN_POINT('',(-10.6942336092596,-2.79024989380572,-84.8));
#37883=CARTESIAN_POINT('',(-8.71475010619428,-0.810766390740372,-84.8));
#37884=CARTESIAN_POINT('Origin',(-10.995,-0.510000000000002,-84.8));
#37885=CARTESIAN_POINT('',(-8.71475010619428,-0.810766390740372,-84.8));
#37886=CARTESIAN_POINT('Origin',(-10.995,-7.69,-84.8));
#37887=CARTESIAN_POINT('',(-8.71475010619428,-7.38923360925963,-81.35));
#37888=CARTESIAN_POINT('',(-10.6942336092596,-5.40975010619428,-81.35));
#37889=CARTESIAN_POINT('Origin',(-10.995,-7.69,-81.35));
#37890=CARTESIAN_POINT('',(-8.71475010619428,-7.38923360925963,-84.8));
#37891=CARTESIAN_POINT('',(-8.71475010619428,-7.38923360925963,-84.8));
#37892=CARTESIAN_POINT('',(-10.6942336092596,-5.40975010619428,-84.8));
#37893=CARTESIAN_POINT('Origin',(-10.995,-7.69,-84.8));
#37894=CARTESIAN_POINT('',(-10.6942336092596,-5.40975010619428,-84.8));
#37895=CARTESIAN_POINT('Origin',(10.995,-0.509999999999999,-84.8));
#37896=CARTESIAN_POINT('',(8.71475010619428,-0.81076639074037,-81.35));
#37897=CARTESIAN_POINT('',(10.6942336092596,-2.79024989380572,-81.35));
#37898=CARTESIAN_POINT('Origin',(10.995,-0.509999999999999,-81.35));
#37899=CARTESIAN_POINT('',(8.71475010619428,-0.81076639074037,-84.8));
#37900=CARTESIAN_POINT('',(8.71475010619428,-0.81076639074037,-84.8));
#37901=CARTESIAN_POINT('',(10.6942336092596,-2.79024989380572,-84.8));
#37902=CARTESIAN_POINT('Origin',(10.995,-0.509999999999999,-84.8));
#37903=CARTESIAN_POINT('',(10.6942336092596,-2.79024989380572,-84.8));
#37904=CARTESIAN_POINT('Origin',(10.995,-7.69,-84.8));
#37905=CARTESIAN_POINT('',(10.6942336092596,-5.40975010619428,-81.35));
#37906=CARTESIAN_POINT('',(8.71475010619428,-7.38923360925963,-81.35));
#37907=CARTESIAN_POINT('Origin',(10.995,-7.69,-81.35));
#37908=CARTESIAN_POINT('',(10.6942336092596,-5.40975010619428,-84.8));
#37909=CARTESIAN_POINT('',(10.6942336092596,-5.40975010619428,-84.8));
#37910=CARTESIAN_POINT('',(8.71475010619428,-7.38923360925963,-84.8));
#37911=CARTESIAN_POINT('Origin',(10.995,-7.69,-84.8));
#37912=CARTESIAN_POINT('',(8.71475010619428,-7.38923360925963,-84.8));
#37913=CARTESIAN_POINT('Origin',(8.55,-12.0328932188134,-84.8));
#37914=CARTESIAN_POINT('Origin',(8.55,-12.0328932188134,-81.35));
#37915=CARTESIAN_POINT('Origin',(8.55,-12.0328932188134,-84.8));
#37916=CARTESIAN_POINT('Origin',(-8.55,-12.0328932188134,-84.8));
#37917=CARTESIAN_POINT('Origin',(-8.55,-12.0328932188134,-81.35));
#37918=CARTESIAN_POINT('Origin',(-8.55,-12.0328932188134,-84.8));
#37919=CARTESIAN_POINT('Origin',(11.,-4.54289321881346,-84.8));
#37920=CARTESIAN_POINT('Origin',(11.,-4.54289321881346,-81.35));
#37921=CARTESIAN_POINT('Origin',(11.,-4.54289321881346,-84.8));
#37922=CARTESIAN_POINT('Origin',(11.,-3.65710678118656,-84.8));
#37923=CARTESIAN_POINT('Origin',(11.,-3.65710678118656,-81.35));
#37924=CARTESIAN_POINT('Origin',(11.,-3.65710678118656,-84.8));
#37925=CARTESIAN_POINT('Origin',(10.6288496112726,-3.28595639245914,-84.8));
#37926=CARTESIAN_POINT('Origin',(10.6288496112726,-3.28595639245914,-81.35));
#37927=CARTESIAN_POINT('Origin',(10.6288496112726,-3.28595639245914,-84.8));
#37928=CARTESIAN_POINT('Origin',(8.21904360754086,-0.876150388727407,-84.8));
#37929=CARTESIAN_POINT('Origin',(8.21904360754086,-0.876150388727407,-81.35));
#37930=CARTESIAN_POINT('Origin',(8.21904360754086,-0.876150388727407,-84.8));
#37931=CARTESIAN_POINT('Origin',(10.6288496112726,-4.91404360754086,-84.8));
#37932=CARTESIAN_POINT('Origin',(10.6288496112726,-4.91404360754086,-81.35));
#37933=CARTESIAN_POINT('Origin',(10.6288496112726,-4.91404360754086,-84.8));
#37934=CARTESIAN_POINT('Origin',(8.21904360754086,-7.32384961127259,-84.8));
#37935=CARTESIAN_POINT('Origin',(8.21904360754086,-7.32384961127259,-81.35));
#37936=CARTESIAN_POINT('Origin',(8.21904360754086,-7.32384961127259,-84.8));
#37937=CARTESIAN_POINT('Origin',(8.55,-8.40710678118654,-84.8));
#37938=CARTESIAN_POINT('Origin',(8.55,-8.40710678118654,-81.35));
#37939=CARTESIAN_POINT('Origin',(8.55,-8.40710678118654,-84.8));
#37940=CARTESIAN_POINT('Origin',(-8.55,-8.40710678118654,-84.8));
#37941=CARTESIAN_POINT('Origin',(-8.55,-8.40710678118654,-81.35));
#37942=CARTESIAN_POINT('Origin',(-8.55,-8.40710678118654,-84.8));
#37943=CARTESIAN_POINT('Origin',(-8.21904360754086,-7.32384961127259,-84.8));
#37944=CARTESIAN_POINT('Origin',(-8.21904360754086,-7.32384961127259,-81.35));
#37945=CARTESIAN_POINT('Origin',(-8.21904360754086,-7.32384961127259,-84.8));
#37946=CARTESIAN_POINT('Origin',(-10.6288496112726,-4.91404360754086,-84.8));
#37947=CARTESIAN_POINT('Origin',(-10.6288496112726,-4.91404360754086,-81.35));
#37948=CARTESIAN_POINT('Origin',(-10.6288496112726,-4.91404360754086,-84.8));
#37949=CARTESIAN_POINT('Origin',(-11.,-4.54289321881346,-84.8));
#37950=CARTESIAN_POINT('Origin',(-11.,-4.54289321881346,-81.35));
#37951=CARTESIAN_POINT('Origin',(-11.,-4.54289321881346,-84.8));
#37952=CARTESIAN_POINT('Origin',(-11.,-3.65710678118656,-84.8));
#37953=CARTESIAN_POINT('Origin',(-11.,-3.65710678118656,-81.35));
#37954=CARTESIAN_POINT('Origin',(-11.,-3.65710678118656,-84.8));
#37955=CARTESIAN_POINT('Origin',(-10.6288496112726,-3.28595639245914,-84.8));
#37956=CARTESIAN_POINT('Origin',(-10.6288496112726,-3.28595639245914,-81.35));
#37957=CARTESIAN_POINT('Origin',(-10.6288496112726,-3.28595639245914,-84.8));
#37958=CARTESIAN_POINT('Origin',(-8.21904360754086,-0.87615038872741,-84.8));
#37959=CARTESIAN_POINT('Origin',(-8.21904360754086,-0.87615038872741,-81.35));
#37960=CARTESIAN_POINT('Origin',(-8.21904360754086,-0.87615038872741,-84.8));
#37961=CARTESIAN_POINT('Origin',(0.,8.,-83.8));
#37962=CARTESIAN_POINT('Origin',(-22.2,13.,-84.8));
#37963=CARTESIAN_POINT('',(-22.2,13.,-84.8));
#37964=CARTESIAN_POINT('',(-22.2,13.,-81.35));
#37965=CARTESIAN_POINT('',(-22.2,13.,-84.8));
#37966=CARTESIAN_POINT('',(22.2,13.,-81.35));
#37967=CARTESIAN_POINT('',(22.2,13.,-81.35));
#37968=CARTESIAN_POINT('',(22.2,13.,-84.8));
#37969=CARTESIAN_POINT('',(22.2,13.,-84.8));
#37970=CARTESIAN_POINT('',(-22.2,13.,-84.8));
#37971=CARTESIAN_POINT('Origin',(0.,0.,-84.8));
#37972=CARTESIAN_POINT('',(-23.2,-15.5,-84.8));
#37973=CARTESIAN_POINT('',(-22.2,-16.5,-84.8));
#37974=CARTESIAN_POINT('',(-23.2,12.,-84.8));
#37975=CARTESIAN_POINT('',(-23.2,-15.5,-84.8));
#37976=CARTESIAN_POINT('',(-23.2,12.,-84.8));
#37977=CARTESIAN_POINT('',(23.2,12.,-84.8));
#37978=CARTESIAN_POINT('',(22.2,13.,-84.8));
#37979=CARTESIAN_POINT('',(23.2,-15.5,-84.8));
#37980=CARTESIAN_POINT('',(23.2,12.,-84.8));
#37981=CARTESIAN_POINT('',(23.2,-15.5,-84.8));
#37982=CARTESIAN_POINT('Origin',(-23.2,12.,-84.8));
#37983=CARTESIAN_POINT('',(-23.2,12.,-81.35));
#37984=CARTESIAN_POINT('',(-23.2,12.,-84.8));
#37985=CARTESIAN_POINT('',(-22.2,13.,-81.35));
#37986=CARTESIAN_POINT('Origin',(-23.2,-15.5,-84.8));
#37987=CARTESIAN_POINT('',(-23.2,-15.5,-81.35));
#37988=CARTESIAN_POINT('',(-23.2,-15.5,-84.8));
#37989=CARTESIAN_POINT('',(-23.2,12.,-81.35));
#37990=CARTESIAN_POINT('Origin',(-22.2,-16.5,-84.8));
#37991=CARTESIAN_POINT('',(-23.2,-15.5,-81.35));
#37992=CARTESIAN_POINT('Origin',(23.2,-15.5,-84.8));
#37993=CARTESIAN_POINT('',(23.2,-15.5,-81.35));
#37994=CARTESIAN_POINT('',(23.2,-15.5,-84.8));
#37995=CARTESIAN_POINT('',(22.2,-16.5,-81.35));
#37996=CARTESIAN_POINT('Origin',(23.2,12.,-84.8));
#37997=CARTESIAN_POINT('',(23.2,12.,-81.35));
#37998=CARTESIAN_POINT('',(23.2,12.,-84.8));
#37999=CARTESIAN_POINT('',(23.2,-15.5,-81.35));
#38000=CARTESIAN_POINT('Origin',(22.2,13.,-84.8));
#38001=CARTESIAN_POINT('',(23.2,12.,-81.35));
#38002=CARTESIAN_POINT('Origin',(-2.3094010767585,8.,-84.4));
#38003=CARTESIAN_POINT('',(-2.3094010767585,8.,-84.4));
#38004=CARTESIAN_POINT('',(-2.3094010767585,8.,-84.4));
#38005=CARTESIAN_POINT('',(-1.15470053837925,10.,-84.4));
#38006=CARTESIAN_POINT('',(-1.15470053837925,10.,-84.4));
#38007=CARTESIAN_POINT('',(-2.3094010767585,8.,-84.4));
#38008=CARTESIAN_POINT('Origin',(-1.15470053837925,6.,-84.4));
#38009=CARTESIAN_POINT('',(-1.15470053837925,6.,-84.4));
#38010=CARTESIAN_POINT('',(-1.15470053837925,6.,-84.4));
#38011=CARTESIAN_POINT('',(-1.15470053837925,6.,-84.4));
#38012=CARTESIAN_POINT('Origin',(1.15470053837925,6.,-84.4));
#38013=CARTESIAN_POINT('',(1.15470053837925,6.,-84.4));
#38014=CARTESIAN_POINT('',(1.15470053837925,6.,-84.4));
#38015=CARTESIAN_POINT('',(1.15470053837925,6.,-84.4));
#38016=CARTESIAN_POINT('Origin',(2.3094010767585,8.,-84.4));
#38017=CARTESIAN_POINT('',(2.3094010767585,8.,-84.4));
#38018=CARTESIAN_POINT('',(2.3094010767585,8.,-84.4));
#38019=CARTESIAN_POINT('',(2.3094010767585,8.,-84.4));
#38020=CARTESIAN_POINT('Origin',(1.15470053837925,10.,-84.4));
#38021=CARTESIAN_POINT('',(1.15470053837925,10.,-84.4));
#38022=CARTESIAN_POINT('',(1.15470053837925,10.,-84.4));
#38023=CARTESIAN_POINT('',(1.15470053837925,10.,-84.4));
#38024=CARTESIAN_POINT('Origin',(-1.15470053837925,10.,-84.4));
#38025=CARTESIAN_POINT('',(-1.15470053837925,10.,-84.4));
#38026=CARTESIAN_POINT('Origin',(0.,0.,-84.4));
#38027=CARTESIAN_POINT('Origin',(-8.55,-12.0328932188134,-81.35));
#38028=CARTESIAN_POINT('',(8.23180194846605,-12.3510912703474,-81.35));
#38029=CARTESIAN_POINT('',(12.3307106781187,-16.45,-81.35));
#38030=CARTESIAN_POINT('',(8.23180194846605,-12.3510912703474,-81.35));
#38031=CARTESIAN_POINT('',(8.1,-12.0328932188134,-81.35));
#38032=CARTESIAN_POINT('Origin',(8.55,-12.0328932188134,-81.35));
#38033=CARTESIAN_POINT('',(8.1,-8.40710678118654,-81.35));
#38034=CARTESIAN_POINT('',(8.1,-8.40710678118654,-81.35));
#38035=CARTESIAN_POINT('',(8.23180194846606,-8.08890872965259,-81.35));
#38036=CARTESIAN_POINT('Origin',(8.55,-8.40710678118654,-81.35));
#38037=CARTESIAN_POINT('',(8.60795233719346,-7.71275834092519,-81.35));
#38038=CARTESIAN_POINT('',(8.60795233719346,-7.71275834092519,-81.35));
#38039=CARTESIAN_POINT('',(8.76432075605962,-7.39577200905833,-81.35));
#38040=CARTESIAN_POINT('Origin',(8.21904360754086,-7.32384961127259,-81.35));
#38041=CARTESIAN_POINT('',(10.7007720090583,-5.45932075605962,-81.35));
#38042=CARTESIAN_POINT('Origin',(10.995,-7.69,-81.35));
#38043=CARTESIAN_POINT('',(11.0177583409252,-5.30295233719346,-81.35));
#38044=CARTESIAN_POINT('Origin',(10.6288496112726,-4.91404360754086,-81.35));
#38045=CARTESIAN_POINT('',(11.3889087296526,-4.93180194846606,-81.35));
#38046=CARTESIAN_POINT('',(11.3889087296526,-4.93180194846606,-81.35));
#38047=CARTESIAN_POINT('',(11.55,-4.54289321881346,-81.35));
#38048=CARTESIAN_POINT('Origin',(11.,-4.54289321881346,-81.35));
#38049=CARTESIAN_POINT('',(11.55,-3.65710678118656,-81.35));
#38050=CARTESIAN_POINT('',(11.55,-3.65710678118656,-81.35));
#38051=CARTESIAN_POINT('',(11.3889087296526,-3.26819805153396,-81.35));
#38052=CARTESIAN_POINT('Origin',(11.,-3.65710678118656,-81.35));
#38053=CARTESIAN_POINT('',(11.0177583409252,-2.89704766280654,-81.35));
#38054=CARTESIAN_POINT('',(11.0177583409252,-2.89704766280654,-81.35));
#38055=CARTESIAN_POINT('',(10.7007720090583,-2.74067924394038,-81.35));
#38056=CARTESIAN_POINT('Origin',(10.6288496112726,-3.28595639245914,-81.35));
#38057=CARTESIAN_POINT('',(8.76432075605962,-0.804227990941667,-81.35));
#38058=CARTESIAN_POINT('Origin',(10.995,-0.509999999999999,-81.35));
#38059=CARTESIAN_POINT('',(8.60795233719346,-0.487241659074806,-81.35));
#38060=CARTESIAN_POINT('Origin',(8.21904360754086,-0.876150388727407,-81.35));
#38061=CARTESIAN_POINT('',(8.07071067811865,0.0500000000000006,-81.35));
#38062=CARTESIAN_POINT('',(8.07071067811865,0.0500000000000006,-81.35));
#38063=CARTESIAN_POINT('',(-8.07071067811865,0.0499999999999998,-81.35));
#38064=CARTESIAN_POINT('',(-8.07071067811865,0.0499999999999998,-81.35));
#38065=CARTESIAN_POINT('',(-8.60795233719346,-0.48724165907481,-81.35));
#38066=CARTESIAN_POINT('',(-8.60795233719346,-0.487241659074809,-81.35));
#38067=CARTESIAN_POINT('',(-8.76432075605962,-0.804227990941668,-81.35));
#38068=CARTESIAN_POINT('Origin',(-8.21904360754086,-0.87615038872741,-81.35));
#38069=CARTESIAN_POINT('',(-10.7007720090583,-2.74067924394038,-81.35));
#38070=CARTESIAN_POINT('Origin',(-10.995,-0.510000000000002,-81.35));
#38071=CARTESIAN_POINT('',(-11.0177583409252,-2.89704766280654,-81.35));
#38072=CARTESIAN_POINT('Origin',(-10.6288496112726,-3.28595639245914,-81.35));
#38073=CARTESIAN_POINT('',(-11.3889087296526,-3.26819805153396,-81.35));
#38074=CARTESIAN_POINT('',(-11.3889087296526,-3.26819805153396,-81.35));
#38075=CARTESIAN_POINT('',(-11.55,-3.65710678118656,-81.35));
#38076=CARTESIAN_POINT('Origin',(-11.,-3.65710678118656,-81.35));
#38077=CARTESIAN_POINT('',(-11.55,-4.54289321881346,-81.35));
#38078=CARTESIAN_POINT('',(-11.55,-4.54289321881346,-81.35));
#38079=CARTESIAN_POINT('',(-11.3889087296526,-4.93180194846607,-81.35));
#38080=CARTESIAN_POINT('Origin',(-11.,-4.54289321881346,-81.35));
#38081=CARTESIAN_POINT('',(-11.0177583409252,-5.30295233719346,-81.35));
#38082=CARTESIAN_POINT('',(-11.0177583409252,-5.30295233719346,-81.35));
#38083=CARTESIAN_POINT('',(-10.7007720090583,-5.45932075605962,-81.35));
#38084=CARTESIAN_POINT('Origin',(-10.6288496112726,-4.91404360754086,-81.35));
#38085=CARTESIAN_POINT('',(-8.76432075605962,-7.39577200905833,-81.35));
#38086=CARTESIAN_POINT('Origin',(-10.995,-7.69,-81.35));
#38087=CARTESIAN_POINT('',(-8.60795233719346,-7.7127583409252,-81.35));
#38088=CARTESIAN_POINT('Origin',(-8.21904360754086,-7.32384961127259,-81.35));
#38089=CARTESIAN_POINT('',(-8.23180194846605,-8.0889087296526,-81.35));
#38090=CARTESIAN_POINT('',(-8.23180194846605,-8.0889087296526,-81.35));
#38091=CARTESIAN_POINT('',(-8.1,-8.40710678118654,-81.35));
#38092=CARTESIAN_POINT('Origin',(-8.55,-8.40710678118654,-81.35));
#38093=CARTESIAN_POINT('',(-8.1,-12.0328932188134,-81.35));
#38094=CARTESIAN_POINT('',(-8.1,-12.0328932188134,-81.35));
#38095=CARTESIAN_POINT('',(-8.23180194846605,-12.3510912703474,-81.35));
#38096=CARTESIAN_POINT('Origin',(-8.55,-12.0328932188134,-81.35));
#38097=CARTESIAN_POINT('',(-12.3307106781186,-16.45,-81.35));
#38098=CARTESIAN_POINT('',(-12.3307106781186,-16.45,-81.35));
#38099=CARTESIAN_POINT('',(-22.1792893218814,-16.45,-81.35));
#38100=CARTESIAN_POINT('',(-22.1792893218814,-16.45,-81.35));
#38101=CARTESIAN_POINT('',(-23.15,-15.4792893218813,-81.35));
#38102=CARTESIAN_POINT('',(-23.15,-15.4792893218813,-81.35));
#38103=CARTESIAN_POINT('',(-23.15,11.9792893218814,-81.35));
#38104=CARTESIAN_POINT('',(-23.15,11.9792893218814,-81.35));
#38105=CARTESIAN_POINT('',(-22.1792893218813,12.95,-81.35));
#38106=CARTESIAN_POINT('',(-22.1792893218813,12.95,-81.35));
#38107=CARTESIAN_POINT('',(22.1792893218813,12.95,-81.35));
#38108=CARTESIAN_POINT('',(22.1792893218813,12.95,-81.35));
#38109=CARTESIAN_POINT('',(23.15,11.9792893218814,-81.35));
#38110=CARTESIAN_POINT('',(23.15,11.9792893218814,-81.35));
#38111=CARTESIAN_POINT('',(23.15,-15.4792893218813,-81.35));
#38112=CARTESIAN_POINT('',(23.15,-15.4792893218813,-81.35));
#38113=CARTESIAN_POINT('',(22.1792893218814,-16.45,-81.35));
#38114=CARTESIAN_POINT('',(22.1792893218814,-16.45,-81.35));
#38115=CARTESIAN_POINT('',(12.3307106781187,-16.45,-81.35));
#38116=CARTESIAN_POINT('Origin',(8.23180194846605,-12.3510912703474,-81.35));
#38117=CARTESIAN_POINT('',(8.23180194846605,-12.3510912703474,-81.3));
#38118=CARTESIAN_POINT('',(12.3307106781187,-16.45,-81.3));
#38119=CARTESIAN_POINT('',(8.23180194846605,-12.3510912703474,-81.3));
#38120=CARTESIAN_POINT('',(8.23180194846605,-12.3510912703474,-81.35));
#38121=CARTESIAN_POINT('',(12.3307106781187,-16.45,-81.35));
#38122=CARTESIAN_POINT('Origin',(8.55,-12.0328932188134,-81.35));
#38123=CARTESIAN_POINT('',(8.1,-12.0328932188134,-81.3));
#38124=CARTESIAN_POINT('Origin',(8.55,-12.0328932188134,-81.3));
#38125=CARTESIAN_POINT('',(8.1,-12.0328932188134,-81.35));
#38126=CARTESIAN_POINT('Origin',(8.1,-8.40710678118654,-81.35));
#38127=CARTESIAN_POINT('',(8.1,-8.40710678118654,-81.3));
#38128=CARTESIAN_POINT('',(8.1,-8.40710678118654,-81.3));
#38129=CARTESIAN_POINT('',(8.1,-8.40710678118654,-81.35));
#38130=CARTESIAN_POINT('Origin',(8.55,-8.40710678118654,-81.35));
#38131=CARTESIAN_POINT('',(8.23180194846606,-8.08890872965259,-81.3));
#38132=CARTESIAN_POINT('Origin',(8.55,-8.40710678118654,-81.3));
#38133=CARTESIAN_POINT('',(8.23180194846606,-8.08890872965259,-81.35));
#38134=CARTESIAN_POINT('Origin',(8.60795233719346,-7.71275834092519,-81.35));
#38135=CARTESIAN_POINT('',(8.60795233719346,-7.71275834092519,-81.3));
#38136=CARTESIAN_POINT('',(8.60795233719346,-7.71275834092519,-81.3));
#38137=CARTESIAN_POINT('',(8.60795233719346,-7.71275834092519,-81.35));
#38138=CARTESIAN_POINT('Origin',(8.21904360754086,-7.32384961127259,-81.35));
#38139=CARTESIAN_POINT('',(8.76432075605962,-7.39577200905833,-81.3));
#38140=CARTESIAN_POINT('Origin',(8.21904360754086,-7.32384961127259,-81.3));
#38141=CARTESIAN_POINT('',(8.76432075605962,-7.39577200905833,-81.35));
#38142=CARTESIAN_POINT('Origin',(10.995,-7.69,-81.35));
#38143=CARTESIAN_POINT('',(10.7007720090583,-5.45932075605962,-81.3));
#38144=CARTESIAN_POINT('Origin',(10.995,-7.69,-81.3));
#38145=CARTESIAN_POINT('',(10.7007720090583,-5.45932075605962,-81.35));
#38146=CARTESIAN_POINT('Origin',(10.6288496112726,-4.91404360754086,-81.35));
#38147=CARTESIAN_POINT('',(11.0177583409252,-5.30295233719346,-81.3));
#38148=CARTESIAN_POINT('Origin',(10.6288496112726,-4.91404360754086,-81.3));
#38149=CARTESIAN_POINT('',(11.0177583409252,-5.30295233719346,-81.35));
#38150=CARTESIAN_POINT('Origin',(11.3889087296526,-4.93180194846606,-81.35));
#38151=CARTESIAN_POINT('',(11.3889087296526,-4.93180194846606,-81.3));
#38152=CARTESIAN_POINT('',(11.3889087296526,-4.93180194846606,-81.3));
#38153=CARTESIAN_POINT('',(11.3889087296526,-4.93180194846606,-81.35));
#38154=CARTESIAN_POINT('Origin',(11.,-4.54289321881346,-81.35));
#38155=CARTESIAN_POINT('',(11.55,-4.54289321881346,-81.3));
#38156=CARTESIAN_POINT('Origin',(11.,-4.54289321881346,-81.3));
#38157=CARTESIAN_POINT('',(11.55,-4.54289321881346,-81.35));
#38158=CARTESIAN_POINT('Origin',(11.55,-3.65710678118656,-81.35));
#38159=CARTESIAN_POINT('',(11.55,-3.65710678118656,-81.3));
#38160=CARTESIAN_POINT('',(11.55,-3.65710678118656,-81.3));
#38161=CARTESIAN_POINT('',(11.55,-3.65710678118656,-81.35));
#38162=CARTESIAN_POINT('Origin',(11.,-3.65710678118656,-81.35));
#38163=CARTESIAN_POINT('',(11.3889087296526,-3.26819805153396,-81.3));
#38164=CARTESIAN_POINT('Origin',(11.,-3.65710678118656,-81.3));
#38165=CARTESIAN_POINT('',(11.3889087296526,-3.26819805153396,-81.35));
#38166=CARTESIAN_POINT('Origin',(11.0177583409252,-2.89704766280654,-81.35));
#38167=CARTESIAN_POINT('',(11.0177583409252,-2.89704766280654,-81.3));
#38168=CARTESIAN_POINT('',(11.0177583409252,-2.89704766280654,-81.3));
#38169=CARTESIAN_POINT('',(11.0177583409252,-2.89704766280654,-81.35));
#38170=CARTESIAN_POINT('Origin',(10.6288496112726,-3.28595639245914,-81.35));
#38171=CARTESIAN_POINT('',(10.7007720090583,-2.74067924394038,-81.3));
#38172=CARTESIAN_POINT('Origin',(10.6288496112726,-3.28595639245914,-81.3));
#38173=CARTESIAN_POINT('',(10.7007720090583,-2.74067924394038,-81.35));
#38174=CARTESIAN_POINT('Origin',(10.995,-0.509999999999999,-81.35));
#38175=CARTESIAN_POINT('',(8.76432075605962,-0.804227990941667,-81.3));
#38176=CARTESIAN_POINT('Origin',(10.995,-0.509999999999999,-81.3));
#38177=CARTESIAN_POINT('',(8.76432075605962,-0.804227990941667,-81.35));
#38178=CARTESIAN_POINT('Origin',(8.21904360754086,-0.876150388727407,-81.35));
#38179=CARTESIAN_POINT('',(8.60795233719346,-0.487241659074806,-81.3));
#38180=CARTESIAN_POINT('Origin',(8.21904360754086,-0.876150388727407,-81.3));
#38181=CARTESIAN_POINT('',(8.60795233719346,-0.487241659074806,-81.35));
#38182=CARTESIAN_POINT('Origin',(8.07071067811865,0.0500000000000006,-81.35));
#38183=CARTESIAN_POINT('',(8.07071067811865,0.0500000000000006,-81.3));
#38184=CARTESIAN_POINT('',(8.07071067811865,0.0500000000000006,-81.3));
#38185=CARTESIAN_POINT('',(8.07071067811865,0.0500000000000006,-81.35));
#38186=CARTESIAN_POINT('Origin',(-8.07071067811865,0.0499999999999998,-81.35));
#38187=CARTESIAN_POINT('',(-8.07071067811865,0.0499999999999998,-81.3));
#38188=CARTESIAN_POINT('',(-8.07071067811865,0.0499999999999998,-81.3));
#38189=CARTESIAN_POINT('',(-8.07071067811865,0.0499999999999998,-81.35));
#38190=CARTESIAN_POINT('Origin',(-8.60795233719346,-0.487241659074809,-81.35));
#38191=CARTESIAN_POINT('',(-8.60795233719346,-0.48724165907481,-81.3));
#38192=CARTESIAN_POINT('',(-8.60795233719346,-0.487241659074809,-81.3));
#38193=CARTESIAN_POINT('',(-8.60795233719346,-0.48724165907481,-81.35));
#38194=CARTESIAN_POINT('Origin',(-8.21904360754086,-0.87615038872741,-81.35));
#38195=CARTESIAN_POINT('',(-8.76432075605962,-0.804227990941668,-81.3));
#38196=CARTESIAN_POINT('Origin',(-8.21904360754086,-0.87615038872741,-81.3));
#38197=CARTESIAN_POINT('',(-8.76432075605962,-0.804227990941668,-81.35));
#38198=CARTESIAN_POINT('Origin',(-10.995,-0.510000000000002,-81.35));
#38199=CARTESIAN_POINT('',(-10.7007720090583,-2.74067924394038,-81.3));
#38200=CARTESIAN_POINT('Origin',(-10.995,-0.510000000000002,-81.3));
#38201=CARTESIAN_POINT('',(-10.7007720090583,-2.74067924394038,-81.35));
#38202=CARTESIAN_POINT('Origin',(-10.6288496112726,-3.28595639245914,-81.35));
#38203=CARTESIAN_POINT('',(-11.0177583409252,-2.89704766280654,-81.3));
#38204=CARTESIAN_POINT('Origin',(-10.6288496112726,-3.28595639245914,-81.3));
#38205=CARTESIAN_POINT('',(-11.0177583409252,-2.89704766280654,-81.35));
#38206=CARTESIAN_POINT('Origin',(-11.3889087296526,-3.26819805153396,-81.35));
#38207=CARTESIAN_POINT('',(-11.3889087296526,-3.26819805153396,-81.3));
#38208=CARTESIAN_POINT('',(-11.3889087296526,-3.26819805153396,-81.3));
#38209=CARTESIAN_POINT('',(-11.3889087296526,-3.26819805153396,-81.35));
#38210=CARTESIAN_POINT('Origin',(-11.,-3.65710678118656,-81.35));
#38211=CARTESIAN_POINT('',(-11.55,-3.65710678118656,-81.3));
#38212=CARTESIAN_POINT('Origin',(-11.,-3.65710678118656,-81.3));
#38213=CARTESIAN_POINT('',(-11.55,-3.65710678118656,-81.35));
#38214=CARTESIAN_POINT('Origin',(-11.55,-4.54289321881346,-81.35));
#38215=CARTESIAN_POINT('',(-11.55,-4.54289321881346,-81.3));
#38216=CARTESIAN_POINT('',(-11.55,-4.54289321881346,-81.3));
#38217=CARTESIAN_POINT('',(-11.55,-4.54289321881346,-81.35));
#38218=CARTESIAN_POINT('Origin',(-11.,-4.54289321881346,-81.35));
#38219=CARTESIAN_POINT('',(-11.3889087296526,-4.93180194846607,-81.3));
#38220=CARTESIAN_POINT('Origin',(-11.,-4.54289321881346,-81.3));
#38221=CARTESIAN_POINT('',(-11.3889087296526,-4.93180194846607,-81.35));
#38222=CARTESIAN_POINT('Origin',(-11.0177583409252,-5.30295233719346,-81.35));
#38223=CARTESIAN_POINT('',(-11.0177583409252,-5.30295233719346,-81.3));
#38224=CARTESIAN_POINT('',(-11.0177583409252,-5.30295233719346,-81.3));
#38225=CARTESIAN_POINT('',(-11.0177583409252,-5.30295233719346,-81.35));
#38226=CARTESIAN_POINT('Origin',(-10.6288496112726,-4.91404360754086,-81.35));
#38227=CARTESIAN_POINT('',(-10.7007720090583,-5.45932075605962,-81.3));
#38228=CARTESIAN_POINT('Origin',(-10.6288496112726,-4.91404360754086,-81.3));
#38229=CARTESIAN_POINT('',(-10.7007720090583,-5.45932075605962,-81.35));
#38230=CARTESIAN_POINT('Origin',(-10.995,-7.69,-81.35));
#38231=CARTESIAN_POINT('',(-8.76432075605962,-7.39577200905833,-81.3));
#38232=CARTESIAN_POINT('Origin',(-10.995,-7.69,-81.3));
#38233=CARTESIAN_POINT('',(-8.76432075605962,-7.39577200905833,-81.35));
#38234=CARTESIAN_POINT('Origin',(-8.21904360754086,-7.32384961127259,-81.35));
#38235=CARTESIAN_POINT('',(-8.60795233719346,-7.7127583409252,-81.3));
#38236=CARTESIAN_POINT('Origin',(-8.21904360754086,-7.32384961127259,-81.3));
#38237=CARTESIAN_POINT('',(-8.60795233719346,-7.7127583409252,-81.35));
#38238=CARTESIAN_POINT('Origin',(-8.23180194846605,-8.0889087296526,-81.35));
#38239=CARTESIAN_POINT('',(-8.23180194846605,-8.0889087296526,-81.3));
#38240=CARTESIAN_POINT('',(-8.23180194846605,-8.0889087296526,-81.3));
#38241=CARTESIAN_POINT('',(-8.23180194846605,-8.0889087296526,-81.35));
#38242=CARTESIAN_POINT('Origin',(-8.55,-8.40710678118654,-81.35));
#38243=CARTESIAN_POINT('',(-8.1,-8.40710678118654,-81.3));
#38244=CARTESIAN_POINT('Origin',(-8.55,-8.40710678118654,-81.3));
#38245=CARTESIAN_POINT('',(-8.1,-8.40710678118654,-81.35));
#38246=CARTESIAN_POINT('Origin',(-8.1,-12.0328932188134,-81.35));
#38247=CARTESIAN_POINT('',(-8.1,-12.0328932188134,-81.3));
#38248=CARTESIAN_POINT('',(-8.1,-12.0328932188134,-81.3));
#38249=CARTESIAN_POINT('',(-8.1,-12.0328932188134,-81.35));
#38250=CARTESIAN_POINT('Origin',(-8.55,-12.0328932188134,-81.35));
#38251=CARTESIAN_POINT('',(-8.23180194846605,-12.3510912703474,-81.3));
#38252=CARTESIAN_POINT('Origin',(-8.55,-12.0328932188134,-81.3));
#38253=CARTESIAN_POINT('',(-8.23180194846605,-12.3510912703474,-81.35));
#38254=CARTESIAN_POINT('Origin',(-12.3307106781186,-16.45,-81.35));
#38255=CARTESIAN_POINT('',(-12.3307106781186,-16.45,-81.3));
#38256=CARTESIAN_POINT('',(-12.3307106781186,-16.45,-81.3));
#38257=CARTESIAN_POINT('',(-12.3307106781186,-16.45,-81.35));
#38258=CARTESIAN_POINT('Origin',(-22.1792893218814,-16.45,-81.35));
#38259=CARTESIAN_POINT('',(-22.1792893218814,-16.45,-81.3));
#38260=CARTESIAN_POINT('',(-22.1792893218814,-16.45,-81.3));
#38261=CARTESIAN_POINT('',(-22.1792893218814,-16.45,-81.35));
#38262=CARTESIAN_POINT('Origin',(-23.15,-15.4792893218813,-81.35));
#38263=CARTESIAN_POINT('',(-23.15,-15.4792893218813,-81.3));
#38264=CARTESIAN_POINT('',(-23.15,-15.4792893218813,-81.3));
#38265=CARTESIAN_POINT('',(-23.15,-15.4792893218813,-81.35));
#38266=CARTESIAN_POINT('Origin',(-23.15,11.9792893218814,-81.35));
#38267=CARTESIAN_POINT('',(-23.15,11.9792893218814,-81.3));
#38268=CARTESIAN_POINT('',(-23.15,11.9792893218814,-81.3));
#38269=CARTESIAN_POINT('',(-23.15,11.9792893218814,-81.35));
#38270=CARTESIAN_POINT('Origin',(-22.1792893218813,12.95,-81.35));
#38271=CARTESIAN_POINT('',(-22.1792893218813,12.95,-81.3));
#38272=CARTESIAN_POINT('',(-22.1792893218813,12.95,-81.3));
#38273=CARTESIAN_POINT('',(-22.1792893218813,12.95,-81.35));
#38274=CARTESIAN_POINT('Origin',(22.1792893218813,12.95,-81.35));
#38275=CARTESIAN_POINT('',(22.1792893218813,12.95,-81.3));
#38276=CARTESIAN_POINT('',(22.1792893218813,12.95,-81.3));
#38277=CARTESIAN_POINT('',(22.1792893218813,12.95,-81.35));
#38278=CARTESIAN_POINT('Origin',(23.15,11.9792893218814,-81.35));
#38279=CARTESIAN_POINT('',(23.15,11.9792893218814,-81.3));
#38280=CARTESIAN_POINT('',(23.15,11.9792893218814,-81.3));
#38281=CARTESIAN_POINT('',(23.15,11.9792893218814,-81.35));
#38282=CARTESIAN_POINT('Origin',(23.15,-15.4792893218813,-81.35));
#38283=CARTESIAN_POINT('',(23.15,-15.4792893218813,-81.3));
#38284=CARTESIAN_POINT('',(23.15,-15.4792893218813,-81.3));
#38285=CARTESIAN_POINT('',(23.15,-15.4792893218813,-81.35));
#38286=CARTESIAN_POINT('Origin',(22.1792893218814,-16.45,-81.35));
#38287=CARTESIAN_POINT('',(22.1792893218814,-16.45,-81.3));
#38288=CARTESIAN_POINT('',(22.1792893218814,-16.45,-81.3));
#38289=CARTESIAN_POINT('',(22.1792893218814,-16.45,-81.35));
#38290=CARTESIAN_POINT('Origin',(12.3307106781187,-16.45,-81.35));
#38291=CARTESIAN_POINT('',(12.3307106781187,-16.45,-81.3));
#38292=CARTESIAN_POINT('Origin',(-1.62630325872826E-14,12.5,-10.6));
#38293=CARTESIAN_POINT('Origin',(-1.50786351795467E-14,12.7,-8.1));
#38294=CARTESIAN_POINT('',(-0.500000000000016,12.7,-8.1));
#38295=CARTESIAN_POINT('',(-0.500000000000016,12.7,-8.1));
#38296=CARTESIAN_POINT('',(0.499999999999983,12.7,-8.1));
#38297=CARTESIAN_POINT('Origin',(-1.50786351795467E-14,12.7,-8.1));
#38298=CARTESIAN_POINT('',(0.499999999999983,12.7,-8.1));
#38299=CARTESIAN_POINT('Origin',(0.,0.,0.));
#38300=CARTESIAN_POINT('',(4.99995,13.,0.));
#38301=CARTESIAN_POINT('',(22.2,13.,0.));
#38302=CARTESIAN_POINT('',(-22.2,13.,0.));
#38303=CARTESIAN_POINT('',(4.99995,8.,0.));
#38304=CARTESIAN_POINT('',(4.99995,13.,0.));
#38305=CARTESIAN_POINT('',(-4.99995,8.,0.));
#38306=CARTESIAN_POINT('Origin',(0.,8.,0.));
#38307=CARTESIAN_POINT('',(-4.99995,13.,0.));
#38308=CARTESIAN_POINT('',(-4.99995,13.,0.));
#38309=CARTESIAN_POINT('',(-22.2,13.,0.));
#38310=CARTESIAN_POINT('',(-22.2,13.,0.));
#38311=CARTESIAN_POINT('',(-23.2,12.,0.));
#38312=CARTESIAN_POINT('',(-22.2,13.,0.));
#38313=CARTESIAN_POINT('',(-23.2,-15.5,0.));
#38314=CARTESIAN_POINT('',(-23.2,12.,0.));
#38315=CARTESIAN_POINT('',(-22.2,-16.5,0.));
#38316=CARTESIAN_POINT('',(-23.2,-15.5,0.));
#38317=CARTESIAN_POINT('',(-12.31,-16.5,0.));
#38318=CARTESIAN_POINT('',(-23.,-16.5,0.));
#38319=CARTESIAN_POINT('',(-8.19644660940672,-12.3864466094067,0.));
#38320=CARTESIAN_POINT('',(-12.31,-16.5,0.));
#38321=CARTESIAN_POINT('',(-8.05,-12.0328932188134,0.));
#38322=CARTESIAN_POINT('Origin',(-8.55,-12.0328932188134,0.));
#38323=CARTESIAN_POINT('',(-8.05,-8.40710678118654,0.));
#38324=CARTESIAN_POINT('',(-8.05,-12.24,0.));
#38325=CARTESIAN_POINT('',(-8.19644660940673,-8.05355339059327,0.));
#38326=CARTESIAN_POINT('Origin',(-8.55,-8.40710678118654,0.));
#38327=CARTESIAN_POINT('',(-8.57259699813413,-7.67740300186587,0.));
#38328=CARTESIAN_POINT('',(-8.05,-8.2,0.));
#38329=CARTESIAN_POINT('',(-8.71475010619428,-7.38923360925963,0.));
#38330=CARTESIAN_POINT('Origin',(-8.21904360754086,-7.32384961127259,0.));
#38331=CARTESIAN_POINT('',(-10.6942336092596,-5.40975010619428,0.));
#38332=CARTESIAN_POINT('Origin',(-10.995,-7.69,0.));
#38333=CARTESIAN_POINT('',(-10.9824030018659,-5.26759699813413,0.));
#38334=CARTESIAN_POINT('Origin',(-10.6288496112726,-4.91404360754086,0.));
#38335=CARTESIAN_POINT('',(-11.3535533905933,-4.89644660940674,0.));
#38336=CARTESIAN_POINT('',(-8.05,-8.2,0.));
#38337=CARTESIAN_POINT('',(-11.5,-4.54289321881346,0.));
#38338=CARTESIAN_POINT('Origin',(-11.,-4.54289321881346,0.));
#38339=CARTESIAN_POINT('',(-11.5,-3.65710678118656,0.));
#38340=CARTESIAN_POINT('',(-11.5,-4.75000000000001,0.));
#38341=CARTESIAN_POINT('',(-11.3535533905933,-3.30355339059329,0.));
#38342=CARTESIAN_POINT('Origin',(-11.,-3.65710678118656,0.));
#38343=CARTESIAN_POINT('',(-10.9824030018659,-2.93240300186587,0.));
#38344=CARTESIAN_POINT('',(-8.05,-1.60428730688303E-15,0.));
#38345=CARTESIAN_POINT('',(-10.6942336092596,-2.79024989380572,0.));
#38346=CARTESIAN_POINT('Origin',(-10.6288496112726,-3.28595639245914,0.));
#38347=CARTESIAN_POINT('',(-8.71475010619428,-0.810766390740372,0.));
#38348=CARTESIAN_POINT('Origin',(-10.995,-0.510000000000002,0.));
#38349=CARTESIAN_POINT('',(-8.57259699813413,-0.522596998134137,0.));
#38350=CARTESIAN_POINT('Origin',(-8.21904360754086,-0.87615038872741,0.));
#38351=CARTESIAN_POINT('',(-8.05,-1.60428730688303E-15,0.));
#38352=CARTESIAN_POINT('',(-8.05,-1.60428730688303E-15,0.));
#38353=CARTESIAN_POINT('',(8.05,3.67394039744206E-16,0.));
#38354=CARTESIAN_POINT('',(8.05,3.67394039744206E-16,0.));
#38355=CARTESIAN_POINT('',(8.57259699813413,-0.522596998134133,0.));
#38356=CARTESIAN_POINT('',(8.05,3.67394039744206E-16,0.));
#38357=CARTESIAN_POINT('',(8.71475010619428,-0.81076639074037,0.));
#38358=CARTESIAN_POINT('Origin',(8.21904360754086,-0.876150388727407,0.));
#38359=CARTESIAN_POINT('',(10.6942336092596,-2.79024989380572,0.));
#38360=CARTESIAN_POINT('Origin',(10.995,-0.509999999999999,0.));
#38361=CARTESIAN_POINT('',(10.9824030018659,-2.93240300186586,0.));
#38362=CARTESIAN_POINT('Origin',(10.6288496112726,-3.28595639245914,0.));
#38363=CARTESIAN_POINT('',(11.3535533905933,-3.30355339059329,0.));
#38364=CARTESIAN_POINT('',(8.05,3.67394039744206E-16,0.));
#38365=CARTESIAN_POINT('',(11.5,-3.65710678118656,0.));
#38366=CARTESIAN_POINT('Origin',(11.,-3.65710678118656,0.));
#38367=CARTESIAN_POINT('',(11.5,-4.54289321881346,0.));
#38368=CARTESIAN_POINT('',(11.5,-4.75000000000001,0.));
#38369=CARTESIAN_POINT('',(11.3535533905933,-4.89644660940673,0.));
#38370=CARTESIAN_POINT('Origin',(11.,-4.54289321881346,0.));
#38371=CARTESIAN_POINT('',(10.9824030018659,-5.26759699813413,0.));
#38372=CARTESIAN_POINT('',(8.05,-8.2,0.));
#38373=CARTESIAN_POINT('',(10.6942336092596,-5.40975010619428,0.));
#38374=CARTESIAN_POINT('Origin',(10.6288496112726,-4.91404360754086,0.));
#38375=CARTESIAN_POINT('',(8.71475010619428,-7.38923360925963,0.));
#38376=CARTESIAN_POINT('Origin',(10.995,-7.69,0.));
#38377=CARTESIAN_POINT('',(8.57259699813413,-7.67740300186587,0.));
#38378=CARTESIAN_POINT('Origin',(8.21904360754086,-7.32384961127259,0.));
#38379=CARTESIAN_POINT('',(8.19644660940673,-8.05355339059327,0.));
#38380=CARTESIAN_POINT('',(8.05,-8.2,0.));
#38381=CARTESIAN_POINT('',(8.05,-8.40710678118654,0.));
#38382=CARTESIAN_POINT('Origin',(8.55,-8.40710678118654,0.));
#38383=CARTESIAN_POINT('',(8.05,-12.0328932188134,0.));
#38384=CARTESIAN_POINT('',(8.05,-12.24,0.));
#38385=CARTESIAN_POINT('',(8.19644660940673,-12.3864466094067,0.));
#38386=CARTESIAN_POINT('Origin',(8.55,-12.0328932188134,0.));
#38387=CARTESIAN_POINT('',(12.31,-16.5,0.));
#38388=CARTESIAN_POINT('',(12.31,-16.5,0.));
#38389=CARTESIAN_POINT('',(22.2,-16.5,0.));
#38390=CARTESIAN_POINT('',(12.31,-16.5,0.));
#38391=CARTESIAN_POINT('',(23.2,-15.5,0.));
#38392=CARTESIAN_POINT('',(23.2,-15.5,0.));
#38393=CARTESIAN_POINT('',(23.2,12.,0.));
#38394=CARTESIAN_POINT('',(23.2,12.,0.));
#38395=CARTESIAN_POINT('',(22.2,13.,0.));
#38396=CARTESIAN_POINT('Origin',(0.499999999999983,12.7,-8.1));
#38397=CARTESIAN_POINT('',(0.499999999999983,13.,-8.1));
#38398=CARTESIAN_POINT('',(0.499999999999983,13.,-8.1));
#38399=CARTESIAN_POINT('',(0.499999999999983,12.7,-8.1));
#38400=CARTESIAN_POINT('Origin',(-0.500000000000016,12.7,-8.1));
#38401=CARTESIAN_POINT('',(-0.500000000000017,13.,-8.1));
#38402=CARTESIAN_POINT('',(-0.500000000000017,13.,-8.1));
#38403=CARTESIAN_POINT('',(-0.500000000000016,12.7,-8.1));
#38404=CARTESIAN_POINT('Origin',(-1.50786351795467E-14,12.7,-8.1));
#38405=CARTESIAN_POINT('Origin',(-1.54689479616415E-14,13.,-8.1));
#38406=CARTESIAN_POINT('Origin',(-1.87674352915389E-14,12.5,-74.2));
#38407=CARTESIAN_POINT('Origin',(-1.50786351795467E-14,12.7,-76.7));
#38408=CARTESIAN_POINT('',(0.499999999999986,12.7,-76.7));
#38409=CARTESIAN_POINT('',(0.499999999999986,12.7,-76.7));
#38410=CARTESIAN_POINT('',(-0.500000000000025,12.7,-76.7));
#38411=CARTESIAN_POINT('Origin',(-1.50786351795467E-14,12.7,-76.7));
#38412=CARTESIAN_POINT('',(-0.500000000000025,12.7,-76.7));
#38413=CARTESIAN_POINT('Origin',(12.31,-16.5,-84.8));
#38414=CARTESIAN_POINT('',(12.31,-16.5,-3.45));
#38415=CARTESIAN_POINT('',(22.2,-16.5,-3.45));
#38416=CARTESIAN_POINT('',(12.31,-16.5,-3.45));
#38417=CARTESIAN_POINT('',(22.2,-16.5,-13.4));
#38418=CARTESIAN_POINT('',(12.31,-16.5,-84.8));
#38419=CARTESIAN_POINT('Origin',(23.2,-15.5,-13.4));
#38420=CARTESIAN_POINT('',(23.2,-15.5,-3.45));
#38421=CARTESIAN_POINT('',(22.2,-16.5,-3.45));
#38422=CARTESIAN_POINT('',(23.2,-15.5,-13.4));
#38423=CARTESIAN_POINT('Origin',(23.2,12.,-13.4));
#38424=CARTESIAN_POINT('',(23.2,12.,-3.45));
#38425=CARTESIAN_POINT('',(23.2,-15.5,-3.45));
#38426=CARTESIAN_POINT('',(23.2,12.,-13.4));
#38427=CARTESIAN_POINT('Origin',(22.2,13.,-13.4));
#38428=CARTESIAN_POINT('',(22.2,13.,-3.45));
#38429=CARTESIAN_POINT('',(23.2,12.,-3.45));
#38430=CARTESIAN_POINT('',(22.2,13.,-13.4));
#38431=CARTESIAN_POINT('Origin',(-22.2,13.,-13.4));
#38432=CARTESIAN_POINT('',(4.99995,13.,-0.999999999999999));
#38433=CARTESIAN_POINT('',(-4.99995,13.,-1.));
#38434=CARTESIAN_POINT('',(-4.99995,13.,-1.));
#38435=CARTESIAN_POINT('',(4.99995,13.,-1.));
#38436=CARTESIAN_POINT('',(-22.2,13.,-3.45));
#38437=CARTESIAN_POINT('',(22.2,13.,-3.45));
#38438=CARTESIAN_POINT('',(-22.2,13.,-13.4));
#38439=CARTESIAN_POINT('',(-4.99995,13.,-1.));
#38440=CARTESIAN_POINT('Origin',(-22.2,13.,-13.4));
#38441=CARTESIAN_POINT('',(-23.2,12.,-3.45));
#38442=CARTESIAN_POINT('',(-22.2,13.,-3.45));
#38443=CARTESIAN_POINT('',(-23.2,12.,-13.4));
#38444=CARTESIAN_POINT('Origin',(-23.2,12.,-13.4));
#38445=CARTESIAN_POINT('',(-23.2,-15.5,-3.45));
#38446=CARTESIAN_POINT('',(-23.2,12.,-3.45));
#38447=CARTESIAN_POINT('',(-23.2,-15.5,-13.4));
#38448=CARTESIAN_POINT('Origin',(-23.2,-15.5,-13.4));
#38449=CARTESIAN_POINT('',(-22.2,-16.5,-3.45));
#38450=CARTESIAN_POINT('',(-23.2,-15.5,-3.45));
#38451=CARTESIAN_POINT('',(-22.2,-16.5,-13.4));
#38452=CARTESIAN_POINT('Origin',(-23.,-16.5,-84.8));
#38453=CARTESIAN_POINT('',(-12.31,-16.5,-3.45));
#38454=CARTESIAN_POINT('',(-22.2,-16.5,-3.45));
#38455=CARTESIAN_POINT('',(-12.31,-16.5,-84.8));
#38456=CARTESIAN_POINT('Origin',(-12.31,-16.5,-84.8));
#38457=CARTESIAN_POINT('',(-8.19644660940672,-12.3864466094067,-3.45));
#38458=CARTESIAN_POINT('',(-12.31,-16.5,-3.45));
#38459=CARTESIAN_POINT('',(-8.19644660940672,-12.3864466094067,-84.8));
#38460=CARTESIAN_POINT('Origin',(-8.55,-12.0328932188134,-84.8));
#38461=CARTESIAN_POINT('',(-8.05,-12.0328932188134,-3.45));
#38462=CARTESIAN_POINT('Origin',(-8.55,-12.0328932188134,-3.45));
#38463=CARTESIAN_POINT('',(-8.05,-12.0328932188134,-84.8));
#38464=CARTESIAN_POINT('Origin',(-8.05,-12.24,-84.8));
#38465=CARTESIAN_POINT('',(-8.05,-8.40710678118654,-3.45));
#38466=CARTESIAN_POINT('',(-8.05,-12.0328932188134,-3.45));
#38467=CARTESIAN_POINT('',(-8.05,-8.40710678118654,-84.8));
#38468=CARTESIAN_POINT('Origin',(-8.55,-8.40710678118654,-84.8));
#38469=CARTESIAN_POINT('',(-8.19644660940673,-8.05355339059327,-3.45));
#38470=CARTESIAN_POINT('Origin',(-8.55,-8.40710678118654,-3.45));
#38471=CARTESIAN_POINT('',(-8.19644660940673,-8.05355339059327,-84.8));
#38472=CARTESIAN_POINT('Origin',(-8.05,-8.2,-84.8));
#38473=CARTESIAN_POINT('',(-8.57259699813413,-7.67740300186587,-3.45));
#38474=CARTESIAN_POINT('',(-8.19644660940673,-8.05355339059327,-3.45));
#38475=CARTESIAN_POINT('',(-8.57259699813413,-7.67740300186587,0.));
#38476=CARTESIAN_POINT('Origin',(-8.21904360754086,-7.32384961127259,-84.8));
#38477=CARTESIAN_POINT('',(-8.71475010619428,-7.38923360925963,-3.45));
#38478=CARTESIAN_POINT('Origin',(-8.21904360754086,-7.32384961127259,-3.45));
#38479=CARTESIAN_POINT('',(-8.71475010619428,-7.38923360925963,-84.8));
#38480=CARTESIAN_POINT('Origin',(-10.995,-7.69,-84.8));
#38481=CARTESIAN_POINT('',(-10.6942336092596,-5.40975010619428,-3.45));
#38482=CARTESIAN_POINT('Origin',(-10.995,-7.69,-3.45));
#38483=CARTESIAN_POINT('',(-10.6942336092596,-5.40975010619428,-84.8));
#38484=CARTESIAN_POINT('Origin',(-10.6288496112726,-4.91404360754086,-84.8));
#38485=CARTESIAN_POINT('',(-10.9824030018659,-5.26759699813413,-3.45));
#38486=CARTESIAN_POINT('Origin',(-10.6288496112726,-4.91404360754086,-3.45));
#38487=CARTESIAN_POINT('',(-10.9824030018659,-5.26759699813413,-84.8));
#38488=CARTESIAN_POINT('Origin',(-8.05,-8.2,-84.8));
#38489=CARTESIAN_POINT('',(-11.3535533905933,-4.89644660940674,-3.45));
#38490=CARTESIAN_POINT('',(-10.9824030018659,-5.26759699813413,-3.45));
#38491=CARTESIAN_POINT('',(-11.3535533905933,-4.89644660940674,0.));
#38492=CARTESIAN_POINT('Origin',(-11.,-4.54289321881346,-84.8));
#38493=CARTESIAN_POINT('',(-11.5,-4.54289321881346,-3.45));
#38494=CARTESIAN_POINT('Origin',(-11.,-4.54289321881346,-3.45));
#38495=CARTESIAN_POINT('',(-11.5,-4.54289321881346,-84.8));
#38496=CARTESIAN_POINT('Origin',(-11.5,-4.75000000000001,-84.8));
#38497=CARTESIAN_POINT('',(-11.5,-3.65710678118656,-3.45));
#38498=CARTESIAN_POINT('',(-11.5,-4.54289321881346,-3.45));
#38499=CARTESIAN_POINT('',(-11.5,-3.65710678118656,0.));
#38500=CARTESIAN_POINT('Origin',(-11.,-3.65710678118656,-84.8));
#38501=CARTESIAN_POINT('',(-11.3535533905933,-3.30355339059329,-3.45));
#38502=CARTESIAN_POINT('Origin',(-11.,-3.65710678118656,-3.45));
#38503=CARTESIAN_POINT('',(-11.3535533905933,-3.30355339059329,-84.8));
#38504=CARTESIAN_POINT('Origin',(-8.05,-1.60428730688303E-15,-84.8));
#38505=CARTESIAN_POINT('',(-10.9824030018659,-2.93240300186587,-3.45));
#38506=CARTESIAN_POINT('',(-11.3535533905933,-3.30355339059329,-3.45));
#38507=CARTESIAN_POINT('',(-10.9824030018659,-2.93240300186587,0.));
#38508=CARTESIAN_POINT('Origin',(-10.6288496112726,-3.28595639245914,-84.8));
#38509=CARTESIAN_POINT('',(-10.6942336092596,-2.79024989380572,-3.45));
#38510=CARTESIAN_POINT('Origin',(-10.6288496112726,-3.28595639245914,-3.45));
#38511=CARTESIAN_POINT('',(-10.6942336092596,-2.79024989380572,-84.8));
#38512=CARTESIAN_POINT('Origin',(-10.995,-0.510000000000002,-84.8));
#38513=CARTESIAN_POINT('',(-8.71475010619428,-0.810766390740372,-3.45));
#38514=CARTESIAN_POINT('Origin',(-10.995,-0.510000000000002,-3.45));
#38515=CARTESIAN_POINT('',(-8.71475010619428,-0.810766390740372,-84.8));
#38516=CARTESIAN_POINT('Origin',(-8.21904360754086,-0.87615038872741,-84.8));
#38517=CARTESIAN_POINT('',(-8.57259699813413,-0.522596998134137,-3.45));
#38518=CARTESIAN_POINT('Origin',(-8.21904360754086,-0.87615038872741,-3.45));
#38519=CARTESIAN_POINT('',(-8.57259699813413,-0.522596998134137,-84.8));
#38520=CARTESIAN_POINT('Origin',(-8.05,-1.60428730688303E-15,-84.8));
#38521=CARTESIAN_POINT('',(-8.05,-1.60428730688303E-15,-3.45));
#38522=CARTESIAN_POINT('',(-8.57259699813413,-0.522596998134137,-3.45));
#38523=CARTESIAN_POINT('',(-8.05,-1.60428730688303E-15,-84.8));
#38524=CARTESIAN_POINT('Origin',(8.05,3.67394039744206E-16,-84.8));
#38525=CARTESIAN_POINT('',(8.05,3.67394039744206E-16,-3.45));
#38526=CARTESIAN_POINT('',(-8.05,-1.60428730688303E-15,-3.45));
#38527=CARTESIAN_POINT('',(8.05,3.67394039744206E-16,-84.8));
#38528=CARTESIAN_POINT('Origin',(8.05,3.67394039744206E-16,-84.8));
#38529=CARTESIAN_POINT('',(8.57259699813413,-0.522596998134133,-3.45));
#38530=CARTESIAN_POINT('',(8.05,3.67394039744206E-16,-3.45));
#38531=CARTESIAN_POINT('',(8.57259699813413,-0.522596998134133,0.));
#38532=CARTESIAN_POINT('Origin',(8.21904360754086,-0.876150388727407,-84.8));
#38533=CARTESIAN_POINT('',(8.71475010619428,-0.81076639074037,-3.45));
#38534=CARTESIAN_POINT('Origin',(8.21904360754086,-0.876150388727407,-3.45));
#38535=CARTESIAN_POINT('',(8.71475010619428,-0.81076639074037,-84.8));
#38536=CARTESIAN_POINT('Origin',(10.995,-0.509999999999999,-84.8));
#38537=CARTESIAN_POINT('',(10.6942336092596,-2.79024989380572,-3.45));
#38538=CARTESIAN_POINT('Origin',(10.995,-0.509999999999999,-3.45));
#38539=CARTESIAN_POINT('',(10.6942336092596,-2.79024989380572,-84.8));
#38540=CARTESIAN_POINT('Origin',(10.6288496112726,-3.28595639245914,-84.8));
#38541=CARTESIAN_POINT('',(10.9824030018659,-2.93240300186586,-3.45));
#38542=CARTESIAN_POINT('Origin',(10.6288496112726,-3.28595639245914,-3.45));
#38543=CARTESIAN_POINT('',(10.9824030018659,-2.93240300186586,-84.8));
#38544=CARTESIAN_POINT('Origin',(8.05,3.67394039744206E-16,-84.8));
#38545=CARTESIAN_POINT('',(11.3535533905933,-3.30355339059329,-3.45));
#38546=CARTESIAN_POINT('',(10.9824030018659,-2.93240300186586,-3.45));
#38547=CARTESIAN_POINT('',(11.3535533905933,-3.30355339059329,0.));
#38548=CARTESIAN_POINT('Origin',(11.,-3.65710678118656,-84.8));
#38549=CARTESIAN_POINT('',(11.5,-3.65710678118656,-3.45));
#38550=CARTESIAN_POINT('Origin',(11.,-3.65710678118656,-3.45));
#38551=CARTESIAN_POINT('',(11.5,-3.65710678118656,-84.8));
#38552=CARTESIAN_POINT('Origin',(11.5,-4.75000000000001,-84.8));
#38553=CARTESIAN_POINT('',(11.5,-4.54289321881346,-3.45));
#38554=CARTESIAN_POINT('',(11.5,-3.65710678118656,-3.45));
#38555=CARTESIAN_POINT('',(11.5,-4.54289321881346,0.));
#38556=CARTESIAN_POINT('Origin',(11.,-4.54289321881346,-84.8));
#38557=CARTESIAN_POINT('',(11.3535533905933,-4.89644660940673,-3.45));
#38558=CARTESIAN_POINT('Origin',(11.,-4.54289321881346,-3.45));
#38559=CARTESIAN_POINT('',(11.3535533905933,-4.89644660940673,-84.8));
#38560=CARTESIAN_POINT('Origin',(8.05,-8.2,-84.8));
#38561=CARTESIAN_POINT('',(10.9824030018659,-5.26759699813413,-3.45));
#38562=CARTESIAN_POINT('',(11.3535533905933,-4.89644660940673,-3.45));
#38563=CARTESIAN_POINT('',(10.9824030018659,-5.26759699813413,0.));
#38564=CARTESIAN_POINT('Origin',(10.6288496112726,-4.91404360754086,-84.8));
#38565=CARTESIAN_POINT('',(10.6942336092596,-5.40975010619428,-3.45));
#38566=CARTESIAN_POINT('Origin',(10.6288496112726,-4.91404360754086,-3.45));
#38567=CARTESIAN_POINT('',(10.6942336092596,-5.40975010619428,-84.8));
#38568=CARTESIAN_POINT('Origin',(10.995,-7.69,-84.8));
#38569=CARTESIAN_POINT('',(8.71475010619428,-7.38923360925963,-3.45));
#38570=CARTESIAN_POINT('Origin',(10.995,-7.69,-3.45));
#38571=CARTESIAN_POINT('',(8.71475010619428,-7.38923360925963,-84.8));
#38572=CARTESIAN_POINT('Origin',(8.21904360754086,-7.32384961127259,-84.8));
#38573=CARTESIAN_POINT('',(8.57259699813413,-7.67740300186587,-3.45));
#38574=CARTESIAN_POINT('Origin',(8.21904360754086,-7.32384961127259,-3.45));
#38575=CARTESIAN_POINT('',(8.57259699813413,-7.67740300186587,-84.8));
#38576=CARTESIAN_POINT('Origin',(8.05,-8.2,-84.8));
#38577=CARTESIAN_POINT('',(8.19644660940673,-8.05355339059327,-3.45));
#38578=CARTESIAN_POINT('',(8.57259699813413,-7.67740300186587,-3.45));
#38579=CARTESIAN_POINT('',(8.19644660940673,-8.05355339059327,-84.8));
#38580=CARTESIAN_POINT('Origin',(8.55,-8.40710678118654,-84.8));
#38581=CARTESIAN_POINT('',(8.05,-8.40710678118654,-3.45));
#38582=CARTESIAN_POINT('Origin',(8.55,-8.40710678118654,-3.45));
#38583=CARTESIAN_POINT('',(8.05,-8.40710678118654,-84.8));
#38584=CARTESIAN_POINT('Origin',(8.05,-12.24,-84.8));
#38585=CARTESIAN_POINT('',(8.05,-12.0328932188134,-3.45));
#38586=CARTESIAN_POINT('',(8.05,-8.40710678118654,-3.45));
#38587=CARTESIAN_POINT('',(8.05,-12.0328932188134,-84.8));
#38588=CARTESIAN_POINT('Origin',(8.55,-12.0328932188134,-84.8));
#38589=CARTESIAN_POINT('',(8.19644660940673,-12.3864466094067,-3.45));
#38590=CARTESIAN_POINT('Origin',(8.55,-12.0328932188134,-3.45));
#38591=CARTESIAN_POINT('',(8.19644660940673,-12.3864466094067,-84.8));
#38592=CARTESIAN_POINT('Origin',(12.31,-16.5,-84.8));
#38593=CARTESIAN_POINT('',(8.19644660940673,-12.3864466094067,-3.45));
#38594=CARTESIAN_POINT('Origin',(-1.54689479616415E-14,13.,-8.1));
#38595=CARTESIAN_POINT('Origin',(-34.5,4.40457132572236E-15,-104.175753233145));
#38596=CARTESIAN_POINT('',(-30.9292009086072,4.33680868994202E-15,-59.4));
#38597=CARTESIAN_POINT('',(-30.9292009086072,4.33680868994202E-15,-25.4));
#38598=CARTESIAN_POINT('',(-30.9292009086072,4.37613505316247E-15,-13.4));
#38599=CARTESIAN_POINT('',(-34.,4.4005895457577E-15,-25.4));
#38600=CARTESIAN_POINT('',(-34.5,4.40457132572236E-15,-25.4));
#38601=CARTESIAN_POINT('',(-34.,4.4005895457577E-15,-59.4));
#38602=CARTESIAN_POINT('',(-34.,4.4005895457577E-15,-104.175753233145));
#38603=CARTESIAN_POINT('',(-34.5,4.40457132572236E-15,-59.4));
#38604=CARTESIAN_POINT('Origin',(35.,6.66784336078585E-15,-104.175753233145));
#38605=CARTESIAN_POINT('',(34.5,6.46233547508513E-15,-59.4));
#38606=CARTESIAN_POINT('',(34.5,6.46233547508513E-15,-25.4));
#38607=CARTESIAN_POINT('',(34.5,6.46233547508513E-15,-104.175753233145));
#38608=CARTESIAN_POINT('',(30.9292009086072,4.77048955893622E-15,-25.4));
#38609=CARTESIAN_POINT('',(35.,6.66784336078585E-15,-25.4));
#38610=CARTESIAN_POINT('',(30.9292009086072,4.99468073201678E-15,-59.4));
#38611=CARTESIAN_POINT('',(30.9292009086072,4.99468073201678E-15,-71.4));
#38612=CARTESIAN_POINT('',(35.,6.66784336078585E-15,-59.4));
#38613=CARTESIAN_POINT('Origin',(-0.500000000000025,12.7,-76.7));
#38614=CARTESIAN_POINT('',(-0.500000000000025,13.,-76.7));
#38615=CARTESIAN_POINT('',(-0.500000000000025,13.,-76.7));
#38616=CARTESIAN_POINT('',(-0.500000000000025,12.7,-76.7));
#38617=CARTESIAN_POINT('Origin',(0.499999999999986,12.7,-76.7));
#38618=CARTESIAN_POINT('',(0.499999999999986,13.,-76.7));
#38619=CARTESIAN_POINT('',(0.499999999999986,13.,-76.7));
#38620=CARTESIAN_POINT('',(0.499999999999986,12.7,-76.7));
#38621=CARTESIAN_POINT('Origin',(-1.50786351795467E-14,12.7,-76.7));
#38622=CARTESIAN_POINT('Origin',(-1.54689479616415E-14,13.,-76.7));
#38623=CARTESIAN_POINT('Origin',(-30.9292009086072,-2.,-104.175753233145));
#38624=CARTESIAN_POINT('',(-28.9973492560291,-1.48236190979496,-25.4));
#38625=CARTESIAN_POINT('Origin',(-30.9292009086072,-2.,-25.4));
#38626=CARTESIAN_POINT('',(-28.9973492560291,-1.48236190979496,-59.4));
#38627=CARTESIAN_POINT('Origin',(-30.9292009086072,-2.,-59.4));
#38628=CARTESIAN_POINT('',(-28.9973492560291,-1.48236190979496,-71.4));
#38629=CARTESIAN_POINT('Origin',(0.,0.,-25.4));
#38630=CARTESIAN_POINT('',(-25.7,-13.788236863595,-25.4));
#38631=CARTESIAN_POINT('',(-29.3945469326493,4.36391374425416E-15,-25.4));
#38632=CARTESIAN_POINT('',(-25.7,0.500000000000004,-25.4));
#38633=CARTESIAN_POINT('',(-25.7,-16.5,-25.4));
#38634=CARTESIAN_POINT('',(-34.5,0.500000000000005,-25.4));
#38635=CARTESIAN_POINT('',(-25.7,0.500000000000004,-25.4));
#38636=CARTESIAN_POINT('',(-34.5,0.500000000000005,-25.4));
#38637=CARTESIAN_POINT('Origin',(-25.7,-16.5,-25.4));
#38638=CARTESIAN_POINT('',(-25.7,-13.788236863595,-24.6339201514178));
#38639=CARTESIAN_POINT('',(-25.7,-13.788236863595,-104.175753233145));
#38640=CARTESIAN_POINT('',(-25.7,0.500000000000004,-24.6339201514178));
#38641=CARTESIAN_POINT('',(-25.7,24.2065391822594,-24.6339201514178));
#38642=CARTESIAN_POINT('',(-25.7,0.500000000000004,-25.4));
#38643=CARTESIAN_POINT('Origin',(25.7,0.500000000000004,-25.4));
#38644=CARTESIAN_POINT('',(25.7,0.500000000000004,-25.4));
#38645=CARTESIAN_POINT('',(25.7,0.499999999999997,-24.6339201514179));
#38646=CARTESIAN_POINT('',(25.7,0.500000000000004,-25.4));
#38647=CARTESIAN_POINT('',(25.7,-13.788236863595,-24.6339201514178));
#38648=CARTESIAN_POINT('',(25.7,24.2065391822594,-24.6339201514179));
#38649=CARTESIAN_POINT('',(25.7,-13.788236863595,-25.4));
#38650=CARTESIAN_POINT('',(25.7,-13.788236863595,-104.175753233145));
#38651=CARTESIAN_POINT('',(25.7,0.500000000000004,-25.4));
#38652=CARTESIAN_POINT('Origin',(0.,0.,-25.4));
#38653=CARTESIAN_POINT('',(28.9973492560291,-1.48236190979496,-25.4));
#38654=CARTESIAN_POINT('',(29.3945469326493,4.36391374425416E-15,-25.4));
#38655=CARTESIAN_POINT('Origin',(30.9292009086072,-2.,-25.4));
#38656=CARTESIAN_POINT('',(35.,0.500000000000005,-25.4));
#38657=CARTESIAN_POINT('',(34.5,6.46233547508513E-15,-25.4));
#38658=CARTESIAN_POINT('',(35.,0.500000000000005,-25.4));
#38659=CARTESIAN_POINT('Origin',(30.9292009086072,-2.,-104.175753233145));
#38660=CARTESIAN_POINT('',(28.9973492560291,-1.48236190979496,-59.4));
#38661=CARTESIAN_POINT('',(28.9973492560291,-1.48236190979496,-13.4));
#38662=CARTESIAN_POINT('Origin',(30.9292009086072,-2.,-59.4));
#38663=CARTESIAN_POINT('Origin',(-8.55,-12.0328932188134,-3.45));
#38664=CARTESIAN_POINT('',(12.3307106781187,-16.45,-3.45));
#38665=CARTESIAN_POINT('',(22.1792893218814,-16.45,-3.45));
#38666=CARTESIAN_POINT('',(12.3307106781187,-16.45,-3.45));
#38667=CARTESIAN_POINT('',(23.15,-15.4792893218813,-3.45));
#38668=CARTESIAN_POINT('',(22.1792893218814,-16.45,-3.45));
#38669=CARTESIAN_POINT('',(23.15,11.9792893218814,-3.45));
#38670=CARTESIAN_POINT('',(23.15,-15.4792893218813,-3.45));
#38671=CARTESIAN_POINT('',(22.1792893218813,12.95,-3.45));
#38672=CARTESIAN_POINT('',(23.15,11.9792893218814,-3.45));
#38673=CARTESIAN_POINT('',(-22.1792893218813,12.95,-3.45));
#38674=CARTESIAN_POINT('',(22.1792893218813,12.95,-3.45));
#38675=CARTESIAN_POINT('',(-23.15,11.9792893218814,-3.45));
#38676=CARTESIAN_POINT('',(-22.1792893218813,12.95,-3.45));
#38677=CARTESIAN_POINT('',(-23.15,-15.4792893218813,-3.45));
#38678=CARTESIAN_POINT('',(-23.15,11.9792893218814,-3.45));
#38679=CARTESIAN_POINT('',(-22.1792893218814,-16.45,-3.45));
#38680=CARTESIAN_POINT('',(-23.15,-15.4792893218813,-3.45));
#38681=CARTESIAN_POINT('',(-12.3307106781186,-16.45,-3.45));
#38682=CARTESIAN_POINT('',(-22.1792893218814,-16.45,-3.45));
#38683=CARTESIAN_POINT('',(-8.23180194846605,-12.3510912703474,-3.45));
#38684=CARTESIAN_POINT('',(-12.3307106781186,-16.45,-3.45));
#38685=CARTESIAN_POINT('',(-8.1,-12.0328932188134,-3.45));
#38686=CARTESIAN_POINT('Origin',(-8.55,-12.0328932188134,-3.45));
#38687=CARTESIAN_POINT('',(-8.1,-8.40710678118654,-3.45));
#38688=CARTESIAN_POINT('',(-8.1,-12.0328932188134,-3.45));
#38689=CARTESIAN_POINT('',(-8.23180194846605,-8.0889087296526,-3.45));
#38690=CARTESIAN_POINT('Origin',(-8.55,-8.40710678118654,-3.45));
#38691=CARTESIAN_POINT('',(-8.60795233719346,-7.7127583409252,-3.45));
#38692=CARTESIAN_POINT('',(-8.23180194846605,-8.0889087296526,-3.45));
#38693=CARTESIAN_POINT('',(-8.76432075605962,-7.39577200905833,-3.45));
#38694=CARTESIAN_POINT('Origin',(-8.21904360754086,-7.32384961127259,-3.45));
#38695=CARTESIAN_POINT('',(-10.7007720090583,-5.45932075605962,-3.45));
#38696=CARTESIAN_POINT('Origin',(-10.995,-7.69,-3.45));
#38697=CARTESIAN_POINT('',(-11.0177583409252,-5.30295233719346,-3.45));
#38698=CARTESIAN_POINT('Origin',(-10.6288496112726,-4.91404360754086,-3.45));
#38699=CARTESIAN_POINT('',(-11.3889087296526,-4.93180194846607,-3.45));
#38700=CARTESIAN_POINT('',(-11.0177583409252,-5.30295233719346,-3.45));
#38701=CARTESIAN_POINT('',(-11.55,-4.54289321881346,-3.45));
#38702=CARTESIAN_POINT('Origin',(-11.,-4.54289321881346,-3.45));
#38703=CARTESIAN_POINT('',(-11.55,-3.65710678118656,-3.45));
#38704=CARTESIAN_POINT('',(-11.55,-4.54289321881346,-3.45));
#38705=CARTESIAN_POINT('',(-11.3889087296526,-3.26819805153396,-3.45));
#38706=CARTESIAN_POINT('Origin',(-11.,-3.65710678118656,-3.45));
#38707=CARTESIAN_POINT('',(-11.0177583409252,-2.89704766280654,-3.45));
#38708=CARTESIAN_POINT('',(-11.3889087296526,-3.26819805153396,-3.45));
#38709=CARTESIAN_POINT('',(-10.7007720090583,-2.74067924394038,-3.45));
#38710=CARTESIAN_POINT('Origin',(-10.6288496112726,-3.28595639245914,-3.45));
#38711=CARTESIAN_POINT('',(-8.76432075605962,-0.804227990941668,-3.45));
#38712=CARTESIAN_POINT('Origin',(-10.995,-0.510000000000002,-3.45));
#38713=CARTESIAN_POINT('',(-8.60795233719346,-0.48724165907481,-3.45));
#38714=CARTESIAN_POINT('Origin',(-8.21904360754086,-0.87615038872741,-3.45));
#38715=CARTESIAN_POINT('',(-8.07071067811865,0.0499999999999998,-3.45));
#38716=CARTESIAN_POINT('',(-8.60795233719346,-0.487241659074809,-3.45));
#38717=CARTESIAN_POINT('',(8.07071067811865,0.0500000000000006,-3.45));
#38718=CARTESIAN_POINT('',(-8.07071067811865,0.0499999999999998,-3.45));
#38719=CARTESIAN_POINT('',(8.60795233719346,-0.487241659074806,-3.45));
#38720=CARTESIAN_POINT('',(8.07071067811865,0.0500000000000006,-3.45));
#38721=CARTESIAN_POINT('',(8.76432075605962,-0.804227990941667,-3.45));
#38722=CARTESIAN_POINT('Origin',(8.21904360754086,-0.876150388727407,-3.45));
#38723=CARTESIAN_POINT('',(10.7007720090583,-2.74067924394038,-3.45));
#38724=CARTESIAN_POINT('Origin',(10.995,-0.509999999999999,-3.45));
#38725=CARTESIAN_POINT('',(11.0177583409252,-2.89704766280654,-3.45));
#38726=CARTESIAN_POINT('Origin',(10.6288496112726,-3.28595639245914,-3.45));
#38727=CARTESIAN_POINT('',(11.3889087296526,-3.26819805153396,-3.45));
#38728=CARTESIAN_POINT('',(11.0177583409252,-2.89704766280654,-3.45));
#38729=CARTESIAN_POINT('',(11.55,-3.65710678118656,-3.45));
#38730=CARTESIAN_POINT('Origin',(11.,-3.65710678118656,-3.45));
#38731=CARTESIAN_POINT('',(11.55,-4.54289321881346,-3.45));
#38732=CARTESIAN_POINT('',(11.55,-3.65710678118656,-3.45));
#38733=CARTESIAN_POINT('',(11.3889087296526,-4.93180194846606,-3.45));
#38734=CARTESIAN_POINT('Origin',(11.,-4.54289321881346,-3.45));
#38735=CARTESIAN_POINT('',(11.0177583409252,-5.30295233719346,-3.45));
#38736=CARTESIAN_POINT('',(11.3889087296526,-4.93180194846606,-3.45));
#38737=CARTESIAN_POINT('',(10.7007720090583,-5.45932075605962,-3.45));
#38738=CARTESIAN_POINT('Origin',(10.6288496112726,-4.91404360754086,-3.45));
#38739=CARTESIAN_POINT('',(8.76432075605962,-7.39577200905833,-3.45));
#38740=CARTESIAN_POINT('Origin',(10.995,-7.69,-3.45));
#38741=CARTESIAN_POINT('',(8.60795233719346,-7.71275834092519,-3.45));
#38742=CARTESIAN_POINT('Origin',(8.21904360754086,-7.32384961127259,-3.45));
#38743=CARTESIAN_POINT('',(8.23180194846606,-8.08890872965259,-3.45));
#38744=CARTESIAN_POINT('',(8.60795233719346,-7.71275834092519,-3.45));
#38745=CARTESIAN_POINT('',(8.1,-8.40710678118654,-3.45));
#38746=CARTESIAN_POINT('Origin',(8.55,-8.40710678118654,-3.45));
#38747=CARTESIAN_POINT('',(8.1,-12.0328932188134,-3.45));
#38748=CARTESIAN_POINT('',(8.1,-8.40710678118654,-3.45));
#38749=CARTESIAN_POINT('',(8.23180194846605,-12.3510912703474,-3.45));
#38750=CARTESIAN_POINT('Origin',(8.55,-12.0328932188134,-3.45));
#38751=CARTESIAN_POINT('',(8.23180194846605,-12.3510912703474,-3.45));
#38752=CARTESIAN_POINT('Origin',(34.5,6.46233547508513E-15,-104.175753233145));
#38753=CARTESIAN_POINT('',(35.,0.500000000000005,-59.4));
#38754=CARTESIAN_POINT('',(35.,0.500000000000007,-104.175753233145));
#38755=CARTESIAN_POINT('',(34.5,6.46233547508513E-15,-59.4));
#38756=CARTESIAN_POINT('Origin',(-34.5,0.500000000000005,-104.175753233145));
#38757=CARTESIAN_POINT('',(-34.5,0.500000000000005,-59.4));
#38758=CARTESIAN_POINT('',(-34.5,0.500000000000005,-104.175753233145));
#38759=CARTESIAN_POINT('',(-34.5,0.500000000000005,-59.4));
#38760=CARTESIAN_POINT('Origin',(0.,0.,-59.4));
#38761=CARTESIAN_POINT('',(-25.7,0.500000000000004,-59.4));
#38762=CARTESIAN_POINT('',(-25.7,-13.788236863595,-59.4));
#38763=CARTESIAN_POINT('',(-25.7,0.500000000000004,-59.4));
#38764=CARTESIAN_POINT('',(-29.3945469326493,4.36391374425416E-15,-59.4));
#38765=CARTESIAN_POINT('',(-35.,0.500000000000005,-59.4));
#38766=CARTESIAN_POINT('Origin',(-25.7,0.500000000000004,-59.4));
#38767=CARTESIAN_POINT('',(-25.7,0.500000000000004,-60.1660798485821));
#38768=CARTESIAN_POINT('',(-25.7,0.500000000000004,-59.4));
#38769=CARTESIAN_POINT('',(-25.7,-13.788236863595,-60.1660798485821));
#38770=CARTESIAN_POINT('',(-25.7,24.2065391822594,-60.1660798485822));
#38771=CARTESIAN_POINT('',(-25.7,-13.788236863595,-104.175753233145));
#38772=CARTESIAN_POINT('Origin',(0.,0.,-59.4));
#38773=CARTESIAN_POINT('',(25.7,0.500000000000004,-59.4));
#38774=CARTESIAN_POINT('',(35.,0.500000000000005,-59.4));
#38775=CARTESIAN_POINT('',(25.7,-13.788236863595,-59.4));
#38776=CARTESIAN_POINT('',(29.3945469326493,4.36391374425416E-15,-59.4));
#38777=CARTESIAN_POINT('',(25.7,0.500000000000004,-59.4));
#38778=CARTESIAN_POINT('Origin',(25.7,0.500000000000004,-59.4));
#38779=CARTESIAN_POINT('',(25.7,-13.788236863595,-60.1660798485821));
#38780=CARTESIAN_POINT('',(25.7,-13.788236863595,-104.175753233145));
#38781=CARTESIAN_POINT('',(25.7,0.499999999999997,-60.1660798485821));
#38782=CARTESIAN_POINT('',(25.7,24.2065391822594,-60.1660798485821));
#38783=CARTESIAN_POINT('',(25.7,0.500000000000004,-59.4));
#38784=CARTESIAN_POINT('Origin',(-1.54689479616415E-14,13.,-76.7));
#38785=CARTESIAN_POINT('Origin',(-29.3945469326493,4.36391374425416E-15,
-104.175753233145));
#38786=CARTESIAN_POINT('Origin',(-28.5,-3.33849460240199,-64.9));
#38787=CARTESIAN_POINT('Origin',(-28.5,-3.33849460240201,-19.9));
#38788=CARTESIAN_POINT('Origin',(35.,0.500000000000005,-25.4));
#38789=CARTESIAN_POINT('',(25.7,0.499999999999997,-15.1660798485821));
#38790=CARTESIAN_POINT('Origin',(28.5,0.499999999999997,-19.9));
#38791=CARTESIAN_POINT('',(35.,0.500000000000005,-13.4));
#38792=CARTESIAN_POINT('',(35.,0.500000000000007,-104.175753233145));
#38793=CARTESIAN_POINT('',(25.7,0.500000000000004,-13.4));
#38794=CARTESIAN_POINT('',(35.,0.500000000000005,-13.4));
#38795=CARTESIAN_POINT('',(25.7,0.500000000000004,-25.4));
#38796=CARTESIAN_POINT('Origin',(25.7,0.500000000000004,-25.4));
#38797=CARTESIAN_POINT('',(25.7,-13.788236863595,-13.4));
#38798=CARTESIAN_POINT('',(25.7,-13.788236863595,-15.1660798485821));
#38799=CARTESIAN_POINT('',(25.7,-13.788236863595,-104.175753233145));
#38800=CARTESIAN_POINT('',(25.7,24.2065391822594,-15.1660798485821));
#38801=CARTESIAN_POINT('',(25.7,0.500000000000004,-13.4));
#38802=CARTESIAN_POINT('Origin',(-29.3945469326493,4.36391374425416E-15,
-104.175753233145));
#38803=CARTESIAN_POINT('',(-25.7,-13.788236863595,-15.1660798485821));
#38804=CARTESIAN_POINT('Origin',(-28.5,-3.33849460240201,-19.9));
#38805=CARTESIAN_POINT('',(-25.7,-13.788236863595,-13.4));
#38806=CARTESIAN_POINT('',(-29.3945469326493,4.36391374425416E-15,-13.4));
#38807=CARTESIAN_POINT('',(-25.7,-13.788236863595,-104.175753233145));
#38808=CARTESIAN_POINT('Origin',(-25.7,-16.5,-25.4));
#38809=CARTESIAN_POINT('',(-25.7,0.500000000000004,-15.1660798485822));
#38810=CARTESIAN_POINT('',(-25.7,0.500000000000004,-13.4));
#38811=CARTESIAN_POINT('',(-25.7,0.500000000000004,-25.4));
#38812=CARTESIAN_POINT('',(-25.7,24.2065391822594,-15.1660798485822));
#38813=CARTESIAN_POINT('',(-25.7,-16.5,-13.4));
#38814=CARTESIAN_POINT('Origin',(-25.7,0.500000000000004,-25.4));
#38815=CARTESIAN_POINT('',(-34.5,0.500000000000005,-13.4));
#38816=CARTESIAN_POINT('',(-25.7,0.500000000000004,-13.4));
#38817=CARTESIAN_POINT('',(-34.5,0.500000000000005,-104.175753233145));
#38818=CARTESIAN_POINT('Origin',(-28.5,0.500000000000004,-19.9));
#38819=CARTESIAN_POINT('Origin',(29.3945469326493,4.36391374425416E-15,
-104.175753233145));
#38820=CARTESIAN_POINT('',(25.4958861827765,-14.55,-15.2929076226792));
#38821=CARTESIAN_POINT('Origin',(28.5,-3.33849460240214,-19.9));
#38822=CARTESIAN_POINT('',(25.4958861827765,-14.55,-13.4));
#38823=CARTESIAN_POINT('',(29.3945469326493,4.36391374425416E-15,-13.4));
#38824=CARTESIAN_POINT('',(25.4958861827765,-14.55,-104.175753233145));
#38825=CARTESIAN_POINT('Origin',(29.3945469326493,4.36391374425416E-15,
-104.175753233145));
#38826=CARTESIAN_POINT('Origin',(28.5,-3.33849460240214,-64.9));
#38827=CARTESIAN_POINT('Origin',(28.5,-3.33849460240214,-19.9));
#38828=CARTESIAN_POINT('Origin',(12.3307106781187,-16.45,-3.45));
#38829=CARTESIAN_POINT('',(12.3307106781187,-16.45,-3.5));
#38830=CARTESIAN_POINT('',(22.1792893218814,-16.45,-3.5));
#38831=CARTESIAN_POINT('',(12.3307106781187,-16.45,-3.5));
#38832=CARTESIAN_POINT('',(22.1792893218814,-16.45,-3.45));
#38833=CARTESIAN_POINT('',(12.3307106781187,-16.45,-3.45));
#38834=CARTESIAN_POINT('Origin',(22.1792893218814,-16.45,-3.45));
#38835=CARTESIAN_POINT('',(23.15,-15.4792893218813,-3.5));
#38836=CARTESIAN_POINT('',(22.1792893218814,-16.45,-3.5));
#38837=CARTESIAN_POINT('',(23.15,-15.4792893218813,-3.45));
#38838=CARTESIAN_POINT('Origin',(23.15,-15.4792893218813,-3.45));
#38839=CARTESIAN_POINT('',(23.15,11.9792893218814,-3.5));
#38840=CARTESIAN_POINT('',(23.15,-15.4792893218813,-3.5));
#38841=CARTESIAN_POINT('',(23.15,11.9792893218814,-3.45));
#38842=CARTESIAN_POINT('Origin',(23.15,11.9792893218814,-3.45));
#38843=CARTESIAN_POINT('',(22.1792893218813,12.95,-3.5));
#38844=CARTESIAN_POINT('',(23.15,11.9792893218814,-3.5));
#38845=CARTESIAN_POINT('',(22.1792893218813,12.95,-3.45));
#38846=CARTESIAN_POINT('Origin',(22.1792893218813,12.95,-3.45));
#38847=CARTESIAN_POINT('',(-22.1792893218813,12.95,-3.5));
#38848=CARTESIAN_POINT('',(22.1792893218813,12.95,-3.5));
#38849=CARTESIAN_POINT('',(-22.1792893218813,12.95,-3.45));
#38850=CARTESIAN_POINT('Origin',(-22.1792893218813,12.95,-3.45));
#38851=CARTESIAN_POINT('',(-23.15,11.9792893218814,-3.5));
#38852=CARTESIAN_POINT('',(-22.1792893218813,12.95,-3.5));
#38853=CARTESIAN_POINT('',(-23.15,11.9792893218814,-3.45));
#38854=CARTESIAN_POINT('Origin',(-23.15,11.9792893218814,-3.45));
#38855=CARTESIAN_POINT('',(-23.15,-15.4792893218813,-3.5));
#38856=CARTESIAN_POINT('',(-23.15,11.9792893218814,-3.5));
#38857=CARTESIAN_POINT('',(-23.15,-15.4792893218813,-3.45));
#38858=CARTESIAN_POINT('Origin',(-23.15,-15.4792893218813,-3.45));
#38859=CARTESIAN_POINT('',(-22.1792893218814,-16.45,-3.5));
#38860=CARTESIAN_POINT('',(-23.15,-15.4792893218813,-3.5));
#38861=CARTESIAN_POINT('',(-22.1792893218814,-16.45,-3.45));
#38862=CARTESIAN_POINT('Origin',(-22.1792893218814,-16.45,-3.45));
#38863=CARTESIAN_POINT('',(-12.3307106781186,-16.45,-3.5));
#38864=CARTESIAN_POINT('',(-22.1792893218814,-16.45,-3.5));
#38865=CARTESIAN_POINT('',(-12.3307106781186,-16.45,-3.45));
#38866=CARTESIAN_POINT('Origin',(-12.3307106781186,-16.45,-3.45));
#38867=CARTESIAN_POINT('',(-8.23180194846605,-12.3510912703474,-3.5));
#38868=CARTESIAN_POINT('',(-12.3307106781186,-16.45,-3.5));
#38869=CARTESIAN_POINT('',(-8.23180194846605,-12.3510912703474,-3.45));
#38870=CARTESIAN_POINT('Origin',(-8.55,-12.0328932188134,-3.45));
#38871=CARTESIAN_POINT('',(-8.1,-12.0328932188134,-3.5));
#38872=CARTESIAN_POINT('Origin',(-8.55,-12.0328932188134,-3.5));
#38873=CARTESIAN_POINT('',(-8.1,-12.0328932188134,-3.45));
#38874=CARTESIAN_POINT('Origin',(-8.1,-12.0328932188134,-3.45));
#38875=CARTESIAN_POINT('',(-8.1,-8.40710678118654,-3.5));
#38876=CARTESIAN_POINT('',(-8.1,-12.0328932188134,-3.5));
#38877=CARTESIAN_POINT('',(-8.1,-8.40710678118654,-3.45));
#38878=CARTESIAN_POINT('Origin',(-8.55,-8.40710678118654,-3.45));
#38879=CARTESIAN_POINT('',(-8.23180194846605,-8.0889087296526,-3.5));
#38880=CARTESIAN_POINT('Origin',(-8.55,-8.40710678118654,-3.5));
#38881=CARTESIAN_POINT('',(-8.23180194846605,-8.0889087296526,-3.45));
#38882=CARTESIAN_POINT('Origin',(-8.23180194846605,-8.0889087296526,-3.45));
#38883=CARTESIAN_POINT('',(-8.60795233719346,-7.7127583409252,-3.5));
#38884=CARTESIAN_POINT('',(-8.23180194846605,-8.0889087296526,-3.5));
#38885=CARTESIAN_POINT('',(-8.60795233719346,-7.7127583409252,-3.45));
#38886=CARTESIAN_POINT('Origin',(-8.21904360754086,-7.32384961127259,-3.45));
#38887=CARTESIAN_POINT('',(-8.76432075605962,-7.39577200905833,-3.5));
#38888=CARTESIAN_POINT('Origin',(-8.21904360754086,-7.32384961127259,-3.5));
#38889=CARTESIAN_POINT('',(-8.76432075605962,-7.39577200905833,-3.45));
#38890=CARTESIAN_POINT('Origin',(-10.995,-7.69,-3.45));
#38891=CARTESIAN_POINT('',(-10.7007720090583,-5.45932075605962,-3.5));
#38892=CARTESIAN_POINT('Origin',(-10.995,-7.69,-3.5));
#38893=CARTESIAN_POINT('',(-10.7007720090583,-5.45932075605962,-3.45));
#38894=CARTESIAN_POINT('Origin',(-10.6288496112726,-4.91404360754086,-3.45));
#38895=CARTESIAN_POINT('',(-11.0177583409252,-5.30295233719346,-3.5));
#38896=CARTESIAN_POINT('Origin',(-10.6288496112726,-4.91404360754086,-3.5));
#38897=CARTESIAN_POINT('',(-11.0177583409252,-5.30295233719346,-3.45));
#38898=CARTESIAN_POINT('Origin',(-11.0177583409252,-5.30295233719346,-3.45));
#38899=CARTESIAN_POINT('',(-11.3889087296526,-4.93180194846607,-3.5));
#38900=CARTESIAN_POINT('',(-11.0177583409252,-5.30295233719346,-3.5));
#38901=CARTESIAN_POINT('',(-11.3889087296526,-4.93180194846607,-3.45));
#38902=CARTESIAN_POINT('Origin',(-11.,-4.54289321881346,-3.45));
#38903=CARTESIAN_POINT('',(-11.55,-4.54289321881346,-3.5));
#38904=CARTESIAN_POINT('Origin',(-11.,-4.54289321881346,-3.5));
#38905=CARTESIAN_POINT('',(-11.55,-4.54289321881346,-3.45));
#38906=CARTESIAN_POINT('Origin',(-11.55,-4.54289321881346,-3.45));
#38907=CARTESIAN_POINT('',(-11.55,-3.65710678118656,-3.5));
#38908=CARTESIAN_POINT('',(-11.55,-4.54289321881346,-3.5));
#38909=CARTESIAN_POINT('',(-11.55,-3.65710678118656,-3.45));
#38910=CARTESIAN_POINT('Origin',(-11.,-3.65710678118656,-3.45));
#38911=CARTESIAN_POINT('',(-11.3889087296526,-3.26819805153396,-3.5));
#38912=CARTESIAN_POINT('Origin',(-11.,-3.65710678118656,-3.5));
#38913=CARTESIAN_POINT('',(-11.3889087296526,-3.26819805153396,-3.45));
#38914=CARTESIAN_POINT('Origin',(-11.3889087296526,-3.26819805153396,-3.45));
#38915=CARTESIAN_POINT('',(-11.0177583409252,-2.89704766280654,-3.5));
#38916=CARTESIAN_POINT('',(-11.3889087296526,-3.26819805153396,-3.5));
#38917=CARTESIAN_POINT('',(-11.0177583409252,-2.89704766280654,-3.45));
#38918=CARTESIAN_POINT('Origin',(-10.6288496112726,-3.28595639245914,-3.45));
#38919=CARTESIAN_POINT('',(-10.7007720090583,-2.74067924394038,-3.5));
#38920=CARTESIAN_POINT('Origin',(-10.6288496112726,-3.28595639245914,-3.5));
#38921=CARTESIAN_POINT('',(-10.7007720090583,-2.74067924394038,-3.45));
#38922=CARTESIAN_POINT('Origin',(-10.995,-0.510000000000002,-3.45));
#38923=CARTESIAN_POINT('',(-8.76432075605962,-0.804227990941668,-3.5));
#38924=CARTESIAN_POINT('Origin',(-10.995,-0.510000000000002,-3.5));
#38925=CARTESIAN_POINT('',(-8.76432075605962,-0.804227990941668,-3.45));
#38926=CARTESIAN_POINT('Origin',(-8.21904360754086,-0.87615038872741,-3.45));
#38927=CARTESIAN_POINT('',(-8.60795233719346,-0.48724165907481,-3.5));
#38928=CARTESIAN_POINT('Origin',(-8.21904360754086,-0.87615038872741,-3.5));
#38929=CARTESIAN_POINT('',(-8.60795233719346,-0.48724165907481,-3.45));
#38930=CARTESIAN_POINT('Origin',(-8.60795233719346,-0.487241659074809,-3.45));
#38931=CARTESIAN_POINT('',(-8.07071067811865,0.0499999999999998,-3.5));
#38932=CARTESIAN_POINT('',(-8.60795233719346,-0.487241659074809,-3.5));
#38933=CARTESIAN_POINT('',(-8.07071067811865,0.0499999999999998,-3.45));
#38934=CARTESIAN_POINT('Origin',(-8.07071067811865,0.0499999999999998,-3.45));
#38935=CARTESIAN_POINT('',(8.07071067811865,0.0500000000000006,-3.5));
#38936=CARTESIAN_POINT('',(-8.07071067811865,0.0499999999999998,-3.5));
#38937=CARTESIAN_POINT('',(8.07071067811865,0.0500000000000006,-3.45));
#38938=CARTESIAN_POINT('Origin',(8.07071067811865,0.0500000000000006,-3.45));
#38939=CARTESIAN_POINT('',(8.60795233719346,-0.487241659074806,-3.5));
#38940=CARTESIAN_POINT('',(8.07071067811865,0.0500000000000006,-3.5));
#38941=CARTESIAN_POINT('',(8.60795233719346,-0.487241659074806,-3.45));
#38942=CARTESIAN_POINT('Origin',(8.21904360754086,-0.876150388727407,-3.45));
#38943=CARTESIAN_POINT('',(8.76432075605962,-0.804227990941667,-3.5));
#38944=CARTESIAN_POINT('Origin',(8.21904360754086,-0.876150388727407,-3.5));
#38945=CARTESIAN_POINT('',(8.76432075605962,-0.804227990941667,-3.45));
#38946=CARTESIAN_POINT('Origin',(10.995,-0.509999999999999,-3.45));
#38947=CARTESIAN_POINT('',(10.7007720090583,-2.74067924394038,-3.5));
#38948=CARTESIAN_POINT('Origin',(10.995,-0.509999999999999,-3.5));
#38949=CARTESIAN_POINT('',(10.7007720090583,-2.74067924394038,-3.45));
#38950=CARTESIAN_POINT('Origin',(10.6288496112726,-3.28595639245914,-3.45));
#38951=CARTESIAN_POINT('',(11.0177583409252,-2.89704766280654,-3.5));
#38952=CARTESIAN_POINT('Origin',(10.6288496112726,-3.28595639245914,-3.5));
#38953=CARTESIAN_POINT('',(11.0177583409252,-2.89704766280654,-3.45));
#38954=CARTESIAN_POINT('Origin',(11.0177583409252,-2.89704766280654,-3.45));
#38955=CARTESIAN_POINT('',(11.3889087296526,-3.26819805153396,-3.5));
#38956=CARTESIAN_POINT('',(11.0177583409252,-2.89704766280654,-3.5));
#38957=CARTESIAN_POINT('',(11.3889087296526,-3.26819805153396,-3.45));
#38958=CARTESIAN_POINT('Origin',(11.,-3.65710678118656,-3.45));
#38959=CARTESIAN_POINT('',(11.55,-3.65710678118656,-3.5));
#38960=CARTESIAN_POINT('Origin',(11.,-3.65710678118656,-3.5));
#38961=CARTESIAN_POINT('',(11.55,-3.65710678118656,-3.45));
#38962=CARTESIAN_POINT('Origin',(11.55,-3.65710678118656,-3.45));
#38963=CARTESIAN_POINT('',(11.55,-4.54289321881346,-3.5));
#38964=CARTESIAN_POINT('',(11.55,-3.65710678118656,-3.5));
#38965=CARTESIAN_POINT('',(11.55,-4.54289321881346,-3.45));
#38966=CARTESIAN_POINT('Origin',(11.,-4.54289321881346,-3.45));
#38967=CARTESIAN_POINT('',(11.3889087296526,-4.93180194846606,-3.5));
#38968=CARTESIAN_POINT('Origin',(11.,-4.54289321881346,-3.5));
#38969=CARTESIAN_POINT('',(11.3889087296526,-4.93180194846606,-3.45));
#38970=CARTESIAN_POINT('Origin',(11.3889087296526,-4.93180194846606,-3.45));
#38971=CARTESIAN_POINT('',(11.0177583409252,-5.30295233719346,-3.5));
#38972=CARTESIAN_POINT('',(11.3889087296526,-4.93180194846606,-3.5));
#38973=CARTESIAN_POINT('',(11.0177583409252,-5.30295233719346,-3.45));
#38974=CARTESIAN_POINT('Origin',(10.6288496112726,-4.91404360754086,-3.45));
#38975=CARTESIAN_POINT('',(10.7007720090583,-5.45932075605962,-3.5));
#38976=CARTESIAN_POINT('Origin',(10.6288496112726,-4.91404360754086,-3.5));
#38977=CARTESIAN_POINT('',(10.7007720090583,-5.45932075605962,-3.45));
#38978=CARTESIAN_POINT('Origin',(10.995,-7.69,-3.45));
#38979=CARTESIAN_POINT('',(8.76432075605962,-7.39577200905833,-3.5));
#38980=CARTESIAN_POINT('Origin',(10.995,-7.69,-3.5));
#38981=CARTESIAN_POINT('',(8.76432075605962,-7.39577200905833,-3.45));
#38982=CARTESIAN_POINT('Origin',(8.21904360754086,-7.32384961127259,-3.45));
#38983=CARTESIAN_POINT('',(8.60795233719346,-7.71275834092519,-3.5));
#38984=CARTESIAN_POINT('Origin',(8.21904360754086,-7.32384961127259,-3.5));
#38985=CARTESIAN_POINT('',(8.60795233719346,-7.71275834092519,-3.45));
#38986=CARTESIAN_POINT('Origin',(8.60795233719346,-7.71275834092519,-3.45));
#38987=CARTESIAN_POINT('',(8.23180194846606,-8.08890872965259,-3.5));
#38988=CARTESIAN_POINT('',(8.60795233719346,-7.71275834092519,-3.5));
#38989=CARTESIAN_POINT('',(8.23180194846606,-8.08890872965259,-3.45));
#38990=CARTESIAN_POINT('Origin',(8.55,-8.40710678118654,-3.45));
#38991=CARTESIAN_POINT('',(8.1,-8.40710678118654,-3.5));
#38992=CARTESIAN_POINT('Origin',(8.55,-8.40710678118654,-3.5));
#38993=CARTESIAN_POINT('',(8.1,-8.40710678118654,-3.45));
#38994=CARTESIAN_POINT('Origin',(8.1,-8.40710678118654,-3.45));
#38995=CARTESIAN_POINT('',(8.1,-12.0328932188134,-3.5));
#38996=CARTESIAN_POINT('',(8.1,-8.40710678118654,-3.5));
#38997=CARTESIAN_POINT('',(8.1,-12.0328932188134,-3.45));
#38998=CARTESIAN_POINT('Origin',(8.55,-12.0328932188134,-3.45));
#38999=CARTESIAN_POINT('',(8.23180194846605,-12.3510912703474,-3.5));
#39000=CARTESIAN_POINT('Origin',(8.55,-12.0328932188134,-3.5));
#39001=CARTESIAN_POINT('',(8.23180194846605,-12.3510912703474,-3.45));
#39002=CARTESIAN_POINT('Origin',(8.23180194846605,-12.3510912703474,-3.45));
#39003=CARTESIAN_POINT('',(8.23180194846605,-12.3510912703474,-3.5));
#39004=CARTESIAN_POINT('Origin',(-1.64657055886728E-14,13.8,-1.36260717503886E-30));
#39005=CARTESIAN_POINT('',(-4.99999999999999,13.8,-3.5));
#39006=CARTESIAN_POINT('',(5.00000000000001,13.8,-3.5));
#39007=CARTESIAN_POINT('',(-5.8,13.8,-3.5));
#39008=CARTESIAN_POINT('',(5.,13.8,-13.4));
#39009=CARTESIAN_POINT('',(5.,13.8,-13.4));
#39010=CARTESIAN_POINT('',(-4.99999999999999,13.8,-13.4));
#39011=CARTESIAN_POINT('',(-5.8,13.8,-13.4));
#39012=CARTESIAN_POINT('',(-4.99999999999999,13.8,-3.5));
#39013=CARTESIAN_POINT('Origin',(5.00000000000001,13.8,-2.19030741916265E-15));
#39014=CARTESIAN_POINT('',(5.8,13.,-3.5));
#39015=CARTESIAN_POINT('',(5.00000000000001,13.8,-3.5));
#39016=CARTESIAN_POINT('',(5.8,13.,-13.4));
#39017=CARTESIAN_POINT('',(5.8,13.,-13.4));
#39018=CARTESIAN_POINT('',(5.00000000000001,13.8,-13.4));
#39019=CARTESIAN_POINT('Origin',(-22.2,13.,-13.4));
#39020=CARTESIAN_POINT('',(22.2,13.,-3.5));
#39021=CARTESIAN_POINT('',(22.2,13.,-3.5));
#39022=CARTESIAN_POINT('',(22.2,13.,-13.4));
#39023=CARTESIAN_POINT('',(22.2,13.,-13.4));
#39024=CARTESIAN_POINT('',(-22.2,13.,-13.4));
#39025=CARTESIAN_POINT('Origin',(22.2,13.,-13.4));
#39026=CARTESIAN_POINT('',(23.2,12.,-3.5));
#39027=CARTESIAN_POINT('',(23.2,12.,-3.5));
#39028=CARTESIAN_POINT('',(23.2,12.,-13.4));
#39029=CARTESIAN_POINT('',(23.2,12.,-13.4));
#39030=CARTESIAN_POINT('',(22.2,13.,-13.4));
#39031=CARTESIAN_POINT('Origin',(23.2,12.,-13.4));
#39032=CARTESIAN_POINT('',(23.2,-15.5,-3.5));
#39033=CARTESIAN_POINT('',(23.2,-15.5,-3.5));
#39034=CARTESIAN_POINT('',(23.2,-15.5,-13.4));
#39035=CARTESIAN_POINT('',(23.2,-15.5,-13.4));
#39036=CARTESIAN_POINT('',(23.2,12.,-13.4));
#39037=CARTESIAN_POINT('Origin',(-23.2,12.,-13.4));
#39038=CARTESIAN_POINT('',(-23.2,12.,-3.5));
#39039=CARTESIAN_POINT('',(-23.2,-15.5,-3.5));
#39040=CARTESIAN_POINT('',(-23.2,12.,-3.5));
#39041=CARTESIAN_POINT('',(-23.2,12.,-13.4));
#39042=CARTESIAN_POINT('',(-23.2,12.,-13.4));
#39043=CARTESIAN_POINT('',(-23.2,-15.5,-13.4));
#39044=CARTESIAN_POINT('',(-23.2,12.,-13.4));
#39045=CARTESIAN_POINT('',(-23.2,-15.5,-13.4));
#39046=CARTESIAN_POINT('Origin',(-22.2,13.,-13.4));
#39047=CARTESIAN_POINT('',(-22.2,13.,-3.5));
#39048=CARTESIAN_POINT('',(-22.2,13.,-3.5));
#39049=CARTESIAN_POINT('',(-22.2,13.,-13.4));
#39050=CARTESIAN_POINT('',(-22.2,13.,-13.4));
#39051=CARTESIAN_POINT('',(-22.2,13.,-13.4));
#39052=CARTESIAN_POINT('Origin',(-22.2,13.,-13.4));
#39053=CARTESIAN_POINT('',(-5.8,13.,-3.5));
#39054=CARTESIAN_POINT('',(22.2,13.,-3.5));
#39055=CARTESIAN_POINT('',(-5.8,13.,-13.4));
#39056=CARTESIAN_POINT('',(-5.8,13.,-13.4));
#39057=CARTESIAN_POINT('',(-22.2,13.,-13.4));
#39058=CARTESIAN_POINT('Origin',(-4.99999999999999,13.8,-4.38061483832526E-16));
#39059=CARTESIAN_POINT('',(-4.99999999999999,13.8,-13.4));
#39060=CARTESIAN_POINT('',(-4.99999999999999,13.8,-3.5));
#39061=CARTESIAN_POINT('Origin',(35.,13.,-104.175753233145));
#39062=CARTESIAN_POINT('',(35.,13.,-13.4));
#39063=CARTESIAN_POINT('',(35.,13.,-13.4));
#39064=CARTESIAN_POINT('',(35.,0.500000000000005,-71.4));
#39065=CARTESIAN_POINT('',(35.,0.500000000000005,-59.4));
#39066=CARTESIAN_POINT('',(35.,13.,-71.4));
#39067=CARTESIAN_POINT('',(35.,13.,-71.4));
#39068=CARTESIAN_POINT('',(35.,13.,-104.175753233145));
#39069=CARTESIAN_POINT('Origin',(34.,14.,-104.175753233145));
#39070=CARTESIAN_POINT('',(34.,14.,-71.4));
#39071=CARTESIAN_POINT('',(34.,14.,-71.4));
#39072=CARTESIAN_POINT('',(34.,14.,-13.4));
#39073=CARTESIAN_POINT('',(34.,14.,-104.175753233145));
#39074=CARTESIAN_POINT('',(34.,14.,-13.4));
#39075=CARTESIAN_POINT('Origin',(-23.,14.,-84.8));
#39076=CARTESIAN_POINT('',(17.505,14.,-71.4));
#39077=CARTESIAN_POINT('',(17.505,14.,-13.4));
#39078=CARTESIAN_POINT('',(17.505,14.,-83.0807063142603));
#39079=CARTESIAN_POINT('',(23.,14.,-13.4));
#39080=CARTESIAN_POINT('',(23.,14.,-71.4));
#39081=CARTESIAN_POINT('Origin',(17.005,13.5,-83.0807063142603));
#39082=CARTESIAN_POINT('',(17.005,13.5,-71.4));
#39083=CARTESIAN_POINT('',(17.005,13.5,-13.4));
#39084=CARTESIAN_POINT('',(17.005,13.5,-83.0807063142603));
#39085=CARTESIAN_POINT('',(17.005,13.5,-13.4));
#39086=CARTESIAN_POINT('',(17.005,13.5,-71.4));
#39087=CARTESIAN_POINT('Origin',(17.005,13.5,-83.0807063142603));
#39088=CARTESIAN_POINT('',(6.33500000000001,13.5,-71.4));
#39089=CARTESIAN_POINT('',(6.33500000000001,13.5,-13.4));
#39090=CARTESIAN_POINT('',(6.33500000000001,13.5,-83.0807063142603));
#39091=CARTESIAN_POINT('',(17.005,13.5,-13.4));
#39092=CARTESIAN_POINT('',(17.005,13.5,-71.4));
#39093=CARTESIAN_POINT('Origin',(6.33500000000001,13.5,-83.0807063142603));
#39094=CARTESIAN_POINT('',(5.835,14.,-71.4));
#39095=CARTESIAN_POINT('',(5.835,14.,-13.4));
#39096=CARTESIAN_POINT('',(5.835,14.,-83.0807063142603));
#39097=CARTESIAN_POINT('',(6.33500000000001,13.5,-13.4));
#39098=CARTESIAN_POINT('',(6.33500000000001,13.5,-71.4));
#39099=CARTESIAN_POINT('Origin',(-23.,14.,-84.8));
#39100=CARTESIAN_POINT('',(-5.835,14.,-71.4));
#39101=CARTESIAN_POINT('',(23.,14.,-71.4));
#39102=CARTESIAN_POINT('',(-5.835,14.,-13.4));
#39103=CARTESIAN_POINT('',(-5.835,14.,-83.0807063142603));
#39104=CARTESIAN_POINT('',(23.,14.,-13.4));
#39105=CARTESIAN_POINT('Origin',(-6.33500000000001,13.5,-83.0807063142603));
#39106=CARTESIAN_POINT('',(-6.33500000000001,13.5,-71.4));
#39107=CARTESIAN_POINT('',(-6.33500000000001,13.5,-13.4));
#39108=CARTESIAN_POINT('',(-6.33500000000001,13.5,-83.0807063142603));
#39109=CARTESIAN_POINT('',(-6.33500000000001,13.5,-13.4));
#39110=CARTESIAN_POINT('',(-6.33500000000001,13.5,-71.4));
#39111=CARTESIAN_POINT('Origin',(-17.005,13.5,-83.0807063142603));
#39112=CARTESIAN_POINT('',(-17.005,13.5,-71.4));
#39113=CARTESIAN_POINT('',(-17.005,13.5,-13.4));
#39114=CARTESIAN_POINT('',(-17.005,13.5,-83.0807063142603));
#39115=CARTESIAN_POINT('',(-17.005,13.5,-13.4));
#39116=CARTESIAN_POINT('',(-17.005,13.5,-71.4));
#39117=CARTESIAN_POINT('Origin',(-17.005,13.5,-83.0807063142603));
#39118=CARTESIAN_POINT('',(-17.505,14.,-71.4));
#39119=CARTESIAN_POINT('',(-17.505,14.,-13.4));
#39120=CARTESIAN_POINT('',(-17.505,14.,-83.0807063142603));
#39121=CARTESIAN_POINT('',(-17.005,13.5,-13.4));
#39122=CARTESIAN_POINT('',(-17.005,13.5,-71.4));
#39123=CARTESIAN_POINT('Origin',(-23.,14.,-84.8));
#39124=CARTESIAN_POINT('',(-34.,14.,-71.4));
#39125=CARTESIAN_POINT('',(23.,14.,-71.4));
#39126=CARTESIAN_POINT('',(-34.,14.,-13.4));
#39127=CARTESIAN_POINT('',(-34.,14.,-104.175753233145));
#39128=CARTESIAN_POINT('',(23.,14.,-13.4));
#39129=CARTESIAN_POINT('Origin',(-34.,14.,-104.175753233145));
#39130=CARTESIAN_POINT('',(-35.,13.,-71.4));
#39131=CARTESIAN_POINT('',(-34.,14.,-71.4));
#39132=CARTESIAN_POINT('',(-35.,13.,-13.4));
#39133=CARTESIAN_POINT('',(-35.,13.,-104.175753233145));
#39134=CARTESIAN_POINT('',(-34.,14.,-13.4));
#39135=CARTESIAN_POINT('Origin',(-35.,13.,-104.175753233145));
#39136=CARTESIAN_POINT('',(-35.,5.6,-71.4));
#39137=CARTESIAN_POINT('',(-35.,13.,-71.4));
#39138=CARTESIAN_POINT('',(-35.,5.6,-13.4));
#39139=CARTESIAN_POINT('',(-35.,5.6,-104.175753233145));
#39140=CARTESIAN_POINT('',(-35.,13.,-13.4));
#39141=CARTESIAN_POINT('Origin',(-35.,5.6,-104.175753233145));
#39142=CARTESIAN_POINT('',(-34.5,5.10000000000001,-71.4));
#39143=CARTESIAN_POINT('',(-35.,5.6,-71.4));
#39144=CARTESIAN_POINT('',(-34.5,5.10000000000001,-13.4));
#39145=CARTESIAN_POINT('',(-34.5,5.10000000000001,-104.175753233145));
#39146=CARTESIAN_POINT('',(-35.,5.6,-13.4));
#39147=CARTESIAN_POINT('Origin',(-34.5,5.10000000000001,-104.175753233145));
#39148=CARTESIAN_POINT('',(-34.5,0.500000000000005,-71.4));
#39149=CARTESIAN_POINT('',(-34.5,5.10000000000001,-71.4));
#39150=CARTESIAN_POINT('',(-34.5,0.500000000000005,-104.175753233145));
#39151=CARTESIAN_POINT('',(-34.5,5.10000000000001,-13.4));
#39152=CARTESIAN_POINT('Origin',(-35.,0.500000000000005,-59.4));
#39153=CARTESIAN_POINT('',(-25.7,0.500000000000004,-69.6339201514178));
#39154=CARTESIAN_POINT('Origin',(-28.5,0.500000000000004,-64.9));
#39155=CARTESIAN_POINT('',(-25.7,0.500000000000004,-71.4));
#39156=CARTESIAN_POINT('',(-35.,0.500000000000005,-71.4));
#39157=CARTESIAN_POINT('',(-25.7,0.500000000000004,-59.4));
#39158=CARTESIAN_POINT('Origin',(-25.7,0.500000000000004,-59.4));
#39159=CARTESIAN_POINT('',(-25.7,-13.788236863595,-71.4));
#39160=CARTESIAN_POINT('',(-25.7,-13.788236863595,-69.6339201514178));
#39161=CARTESIAN_POINT('',(-25.7,-13.788236863595,-104.175753233145));
#39162=CARTESIAN_POINT('',(-25.7,24.2065391822594,-69.6339201514178));
#39163=CARTESIAN_POINT('',(-25.7,0.500000000000004,-71.4));
#39164=CARTESIAN_POINT('Origin',(-29.3945469326493,4.36391374425416E-15,
-104.175753233145));
#39165=CARTESIAN_POINT('',(-25.4958861827765,-14.55,-69.5070923773207));
#39166=CARTESIAN_POINT('Origin',(-28.5,-3.33849460240199,-64.9));
#39167=CARTESIAN_POINT('',(-25.4958861827765,-14.55,-71.4));
#39168=CARTESIAN_POINT('',(-29.3945469326493,4.36391374425416E-15,-71.4));
#39169=CARTESIAN_POINT('',(-25.4958861827765,-14.55,-104.175753233145));
#39170=CARTESIAN_POINT('Origin',(29.3945469326493,4.36391374425416E-15,
-104.175753233145));
#39171=CARTESIAN_POINT('',(25.7,-13.788236863595,-69.6339201514178));
#39172=CARTESIAN_POINT('Origin',(28.5,-3.33849460240214,-64.9));
#39173=CARTESIAN_POINT('',(25.7,-13.788236863595,-71.4));
#39174=CARTESIAN_POINT('',(29.3945469326493,4.36391374425416E-15,-71.4));
#39175=CARTESIAN_POINT('',(25.7,-13.788236863595,-104.175753233145));
#39176=CARTESIAN_POINT('Origin',(25.7,0.500000000000004,-59.4));
#39177=CARTESIAN_POINT('',(25.7,0.499999999999997,-69.6339201514178));
#39178=CARTESIAN_POINT('',(25.7,0.500000000000004,-71.4));
#39179=CARTESIAN_POINT('',(25.7,0.500000000000004,-59.4));
#39180=CARTESIAN_POINT('',(25.7,24.2065391822594,-69.6339201514178));
#39181=CARTESIAN_POINT('',(25.7,0.500000000000004,-71.4));
#39182=CARTESIAN_POINT('Origin',(35.,0.500000000000005,-59.4));
#39183=CARTESIAN_POINT('',(35.,0.500000000000005,-71.4));
#39184=CARTESIAN_POINT('Origin',(28.5,0.499999999999997,-64.9));
#39185=CARTESIAN_POINT('Origin',(-25.4958861827765,-14.55,-104.175753233145));
#39186=CARTESIAN_POINT('Origin',(-28.5000000000034,-12.2029290542103,-64.8999999999982));
#39187=CARTESIAN_POINT('',(-23.,-16.5,-71.4));
#39188=CARTESIAN_POINT('',(-25.4958861827765,-14.55,-71.4));
#39189=CARTESIAN_POINT('',(-23.,-16.5,-84.8));
#39190=CARTESIAN_POINT('Origin',(-23.2,-15.5,-13.4));
#39191=CARTESIAN_POINT('',(-22.2,-16.5,-3.5));
#39192=CARTESIAN_POINT('',(-23.2,-15.5,-3.5));
#39193=CARTESIAN_POINT('',(-22.2,-16.5,-13.4));
#39194=CARTESIAN_POINT('',(-23.2,-15.5,-13.4));
#39195=CARTESIAN_POINT('',(-22.2,-16.5,-13.4));
#39196=CARTESIAN_POINT('Origin',(23.2,-15.5,-13.4));
#39197=CARTESIAN_POINT('',(22.2,-16.5,-3.5));
#39198=CARTESIAN_POINT('',(22.2,-16.5,-3.5));
#39199=CARTESIAN_POINT('',(22.2,-16.5,-13.4));
#39200=CARTESIAN_POINT('',(22.2,-16.5,-13.4));
#39201=CARTESIAN_POINT('',(23.2,-15.5,-13.4));
#39202=CARTESIAN_POINT('Origin',(0.,0.,-13.4));
#39203=CARTESIAN_POINT('',(-23.,-16.5,-13.4));
#39204=CARTESIAN_POINT('',(23.,-16.5,-13.4));
#39205=CARTESIAN_POINT('',(22.2,-16.5,-13.4));
#39206=CARTESIAN_POINT('',(25.4958861827765,-14.55,-13.4));
#39207=CARTESIAN_POINT('Origin',(25.4958861827765,-14.55,-104.175753233145));
#39208=CARTESIAN_POINT('Origin',(28.5000000000021,-12.2029290542113,-19.9000000000011));
#39209=CARTESIAN_POINT('',(23.,-16.5,-84.8));
#39210=CARTESIAN_POINT('Origin',(-5.8,13.8,-3.5));
#39211=CARTESIAN_POINT('',(-12.31,-16.5,-3.5));
#39212=CARTESIAN_POINT('',(-22.2,-16.5,-3.5));
#39213=CARTESIAN_POINT('',(-8.19644660940672,-12.3864466094067,-3.5));
#39214=CARTESIAN_POINT('',(-12.31,-16.5,-3.5));
#39215=CARTESIAN_POINT('',(-8.05,-12.0328932188134,-3.5));
#39216=CARTESIAN_POINT('Origin',(-8.55,-12.0328932188134,-3.5));
#39217=CARTESIAN_POINT('',(-8.05,-8.40710678118654,-3.5));
#39218=CARTESIAN_POINT('',(-8.05,-12.0328932188134,-3.5));
#39219=CARTESIAN_POINT('',(-8.19644660940673,-8.05355339059327,-3.5));
#39220=CARTESIAN_POINT('Origin',(-8.55,-8.40710678118654,-3.5));
#39221=CARTESIAN_POINT('',(-8.57259699813413,-7.67740300186587,-3.5));
#39222=CARTESIAN_POINT('',(-8.19644660940673,-8.05355339059327,-3.5));
#39223=CARTESIAN_POINT('',(-8.71475010619428,-7.38923360925963,-3.5));
#39224=CARTESIAN_POINT('Origin',(-8.21904360754086,-7.32384961127259,-3.5));
#39225=CARTESIAN_POINT('',(-10.6942336092596,-5.40975010619428,-3.5));
#39226=CARTESIAN_POINT('Origin',(-10.995,-7.69,-3.5));
#39227=CARTESIAN_POINT('',(-10.9824030018659,-5.26759699813413,-3.5));
#39228=CARTESIAN_POINT('Origin',(-10.6288496112726,-4.91404360754086,-3.5));
#39229=CARTESIAN_POINT('',(-11.3535533905933,-4.89644660940674,-3.5));
#39230=CARTESIAN_POINT('',(-10.9824030018659,-5.26759699813413,-3.5));
#39231=CARTESIAN_POINT('',(-11.5,-4.54289321881346,-3.5));
#39232=CARTESIAN_POINT('Origin',(-11.,-4.54289321881346,-3.5));
#39233=CARTESIAN_POINT('',(-11.5,-3.65710678118656,-3.5));
#39234=CARTESIAN_POINT('',(-11.5,-4.54289321881346,-3.5));
#39235=CARTESIAN_POINT('',(-11.3535533905933,-3.30355339059329,-3.5));
#39236=CARTESIAN_POINT('Origin',(-11.,-3.65710678118656,-3.5));
#39237=CARTESIAN_POINT('',(-10.9824030018659,-2.93240300186587,-3.5));
#39238=CARTESIAN_POINT('',(-11.3535533905933,-3.30355339059329,-3.5));
#39239=CARTESIAN_POINT('',(-10.6942336092596,-2.79024989380572,-3.5));
#39240=CARTESIAN_POINT('Origin',(-10.6288496112726,-3.28595639245914,-3.5));
#39241=CARTESIAN_POINT('',(-8.71475010619428,-0.810766390740372,-3.5));
#39242=CARTESIAN_POINT('Origin',(-10.995,-0.510000000000002,-3.5));
#39243=CARTESIAN_POINT('',(-8.57259699813413,-0.522596998134137,-3.5));
#39244=CARTESIAN_POINT('Origin',(-8.21904360754086,-0.87615038872741,-3.5));
#39245=CARTESIAN_POINT('',(-8.05,-1.60428730688303E-15,-3.5));
#39246=CARTESIAN_POINT('',(-8.57259699813413,-0.522596998134137,-3.5));
#39247=CARTESIAN_POINT('',(8.05,3.67394039744206E-16,-3.5));
#39248=CARTESIAN_POINT('',(-8.05,-1.60428730688303E-15,-3.5));
#39249=CARTESIAN_POINT('',(8.57259699813413,-0.522596998134133,-3.5));
#39250=CARTESIAN_POINT('',(8.05,3.67394039744206E-16,-3.5));
#39251=CARTESIAN_POINT('',(8.71475010619428,-0.81076639074037,-3.5));
#39252=CARTESIAN_POINT('Origin',(8.21904360754086,-0.876150388727407,-3.5));
#39253=CARTESIAN_POINT('',(10.6942336092596,-2.79024989380572,-3.5));
#39254=CARTESIAN_POINT('Origin',(10.995,-0.509999999999999,-3.5));
#39255=CARTESIAN_POINT('',(10.9824030018659,-2.93240300186586,-3.5));
#39256=CARTESIAN_POINT('Origin',(10.6288496112726,-3.28595639245914,-3.5));
#39257=CARTESIAN_POINT('',(11.3535533905933,-3.30355339059329,-3.5));
#39258=CARTESIAN_POINT('',(10.9824030018659,-2.93240300186586,-3.5));
#39259=CARTESIAN_POINT('',(11.5,-3.65710678118656,-3.5));
#39260=CARTESIAN_POINT('Origin',(11.,-3.65710678118656,-3.5));
#39261=CARTESIAN_POINT('',(11.5,-4.54289321881346,-3.5));
#39262=CARTESIAN_POINT('',(11.5,-3.65710678118656,-3.5));
#39263=CARTESIAN_POINT('',(11.3535533905933,-4.89644660940673,-3.5));
#39264=CARTESIAN_POINT('Origin',(11.,-4.54289321881346,-3.5));
#39265=CARTESIAN_POINT('',(10.9824030018659,-5.26759699813413,-3.5));
#39266=CARTESIAN_POINT('',(11.3535533905933,-4.89644660940673,-3.5));
#39267=CARTESIAN_POINT('',(10.6942336092596,-5.40975010619428,-3.5));
#39268=CARTESIAN_POINT('Origin',(10.6288496112726,-4.91404360754086,-3.5));
#39269=CARTESIAN_POINT('',(8.71475010619428,-7.38923360925963,-3.5));
#39270=CARTESIAN_POINT('Origin',(10.995,-7.69,-3.5));
#39271=CARTESIAN_POINT('',(8.57259699813413,-7.67740300186587,-3.5));
#39272=CARTESIAN_POINT('Origin',(8.21904360754086,-7.32384961127259,-3.5));
#39273=CARTESIAN_POINT('',(8.19644660940673,-8.05355339059327,-3.5));
#39274=CARTESIAN_POINT('',(8.57259699813413,-7.67740300186587,-3.5));
#39275=CARTESIAN_POINT('',(8.05,-8.40710678118654,-3.5));
#39276=CARTESIAN_POINT('Origin',(8.55,-8.40710678118654,-3.5));
#39277=CARTESIAN_POINT('',(8.05,-12.0328932188134,-3.5));
#39278=CARTESIAN_POINT('',(8.05,-8.40710678118654,-3.5));
#39279=CARTESIAN_POINT('',(8.19644660940673,-12.3864466094067,-3.5));
#39280=CARTESIAN_POINT('Origin',(8.55,-12.0328932188134,-3.5));
#39281=CARTESIAN_POINT('',(12.31,-16.5,-3.5));
#39282=CARTESIAN_POINT('',(8.19644660940673,-12.3864466094067,-3.5));
#39283=CARTESIAN_POINT('',(12.31,-16.5,-3.5));
#39284=CARTESIAN_POINT('Origin',(0.,0.,-71.4));
#39285=CARTESIAN_POINT('',(22.2,-16.5,-71.4));
#39286=CARTESIAN_POINT('',(22.2,-16.5,-71.4));
#39287=CARTESIAN_POINT('',(23.2,-15.5,-71.4));
#39288=CARTESIAN_POINT('',(23.2,-15.5,-71.4));
#39289=CARTESIAN_POINT('',(23.2,12.,-71.4));
#39290=CARTESIAN_POINT('',(23.2,12.,-71.4));
#39291=CARTESIAN_POINT('',(22.2,13.,-71.4));
#39292=CARTESIAN_POINT('',(22.2,13.,-71.4));
#39293=CARTESIAN_POINT('',(5.79999999999999,13.,-71.4));
#39294=CARTESIAN_POINT('',(-22.2,13.,-71.4));
#39295=CARTESIAN_POINT('',(4.99999999999997,13.8,-71.4));
#39296=CARTESIAN_POINT('',(4.99999999999996,13.8,-71.4));
#39297=CARTESIAN_POINT('',(-4.99999999999998,13.8,-71.4));
#39298=CARTESIAN_POINT('',(-5.79999999999999,13.8,-71.4));
#39299=CARTESIAN_POINT('',(-5.79999999999999,13.,-71.4));
#39300=CARTESIAN_POINT('',(-4.99999999999997,13.8,-71.4));
#39301=CARTESIAN_POINT('',(-22.2,13.,-71.4));
#39302=CARTESIAN_POINT('',(-22.2,13.,-71.4));
#39303=CARTESIAN_POINT('',(-23.2,12.,-71.4));
#39304=CARTESIAN_POINT('',(-23.2,12.,-71.4));
#39305=CARTESIAN_POINT('',(-23.2,-15.5,-71.4));
#39306=CARTESIAN_POINT('',(-23.2,-15.5,-71.4));
#39307=CARTESIAN_POINT('',(-22.2,-16.5,-71.4));
#39308=CARTESIAN_POINT('',(-22.2,-16.5,-71.4));
#39309=CARTESIAN_POINT('',(-23.,-16.5,-71.4));
#39310=CARTESIAN_POINT('Origin',(-4.99999999999996,13.8,1.31418445149757E-15));
#39311=CARTESIAN_POINT('',(-5.79999999999999,13.,-81.3));
#39312=CARTESIAN_POINT('',(-4.99999999999999,13.8,-81.3));
#39313=CARTESIAN_POINT('',(-4.99999999999997,13.8,-81.3));
#39314=CARTESIAN_POINT('',(-5.8,13.,-81.3));
#39315=CARTESIAN_POINT('',(-4.99999999999998,13.8,-71.4));
#39316=CARTESIAN_POINT('Origin',(22.2,13.,-84.8));
#39317=CARTESIAN_POINT('',(23.2,12.,-81.3));
#39318=CARTESIAN_POINT('',(22.2,13.,-81.3));
#39319=CARTESIAN_POINT('',(23.2,12.,-81.3));
#39320=CARTESIAN_POINT('',(22.2,13.,-84.8));
#39321=CARTESIAN_POINT('',(23.2,12.,-84.8));
#39322=CARTESIAN_POINT('Origin',(23.2,12.,-84.8));
#39323=CARTESIAN_POINT('',(23.2,-15.5,-81.3));
#39324=CARTESIAN_POINT('',(23.2,-15.5,-81.3));
#39325=CARTESIAN_POINT('',(23.2,-15.5,-84.8));
#39326=CARTESIAN_POINT('Origin',(23.2,-15.5,-84.8));
#39327=CARTESIAN_POINT('',(22.2,-16.5,-81.3));
#39328=CARTESIAN_POINT('',(22.2,-16.5,-81.3));
#39329=CARTESIAN_POINT('',(22.2,-16.5,-84.8));
#39330=CARTESIAN_POINT('Origin',(-22.2,13.,-84.8));
#39331=CARTESIAN_POINT('',(5.8,13.,-81.3));
#39332=CARTESIAN_POINT('',(22.2,13.,-81.3));
#39333=CARTESIAN_POINT('',(5.8,13.,-81.3));
#39334=CARTESIAN_POINT('Origin',(8.55,-12.0328932188134,-84.8));
#39335=CARTESIAN_POINT('',(8.05,-12.0328932188134,-81.3));
#39336=CARTESIAN_POINT('',(8.05,-12.0328932188134,-84.8));
#39337=CARTESIAN_POINT('',(8.19644660940673,-12.3864466094067,-81.3));
#39338=CARTESIAN_POINT('Origin',(8.55,-12.0328932188134,-81.3));
#39339=CARTESIAN_POINT('',(8.19644660940673,-12.3864466094067,-84.8));
#39340=CARTESIAN_POINT('Origin',(8.55,-8.40710678118654,-84.8));
#39341=CARTESIAN_POINT('',(8.19644660940673,-8.05355339059327,-81.3));
#39342=CARTESIAN_POINT('',(8.19644660940673,-8.05355339059327,-84.8));
#39343=CARTESIAN_POINT('',(8.05,-8.40710678118654,-81.3));
#39344=CARTESIAN_POINT('Origin',(8.55,-8.40710678118654,-81.3));
#39345=CARTESIAN_POINT('',(8.05,-8.40710678118654,-84.8));
#39346=CARTESIAN_POINT('Origin',(8.05,-12.24,-84.8));
#39347=CARTESIAN_POINT('',(8.05,-8.40710678118654,-81.3));
#39348=CARTESIAN_POINT('Origin',(12.31,-16.5,-84.8));
#39349=CARTESIAN_POINT('',(12.31,-16.5,-81.3));
#39350=CARTESIAN_POINT('',(8.19644660940673,-12.3864466094067,-81.3));
#39351=CARTESIAN_POINT('',(12.31,-16.5,-84.8));
#39352=CARTESIAN_POINT('Origin',(12.31,-16.5,-84.8));
#39353=CARTESIAN_POINT('',(12.31,-16.5,-81.3));
#39354=CARTESIAN_POINT('Origin',(8.21904360754086,-7.32384961127259,-84.8));
#39355=CARTESIAN_POINT('',(8.71475010619428,-7.38923360925963,-81.3));
#39356=CARTESIAN_POINT('',(8.57259699813413,-7.67740300186587,-81.3));
#39357=CARTESIAN_POINT('Origin',(8.21904360754086,-7.32384961127259,-81.3));
#39358=CARTESIAN_POINT('',(8.57259699813413,-7.67740300186587,-84.8));
#39359=CARTESIAN_POINT('',(8.71475010619428,-7.38923360925963,-84.8));
#39360=CARTESIAN_POINT('Origin',(10.6288496112726,-4.91404360754086,-84.8));
#39361=CARTESIAN_POINT('',(10.9824030018659,-5.26759699813413,-81.3));
#39362=CARTESIAN_POINT('',(10.6942336092596,-5.40975010619428,-81.3));
#39363=CARTESIAN_POINT('Origin',(10.6288496112726,-4.91404360754086,-81.3));
#39364=CARTESIAN_POINT('',(10.6942336092596,-5.40975010619428,-84.8));
#39365=CARTESIAN_POINT('',(10.9824030018659,-5.26759699813413,0.));
#39366=CARTESIAN_POINT('Origin',(10.995,-7.69,-84.8));
#39367=CARTESIAN_POINT('Origin',(10.995,-7.69,-81.3));
#39368=CARTESIAN_POINT('Origin',(11.,-4.54289321881346,-84.8));
#39369=CARTESIAN_POINT('',(11.5,-4.54289321881346,-81.3));
#39370=CARTESIAN_POINT('',(11.3535533905933,-4.89644660940673,-81.3));
#39371=CARTESIAN_POINT('Origin',(11.,-4.54289321881346,-81.3));
#39372=CARTESIAN_POINT('',(11.3535533905933,-4.89644660940673,-84.8));
#39373=CARTESIAN_POINT('',(11.5,-4.54289321881346,0.));
#39374=CARTESIAN_POINT('Origin',(11.,-3.65710678118656,-84.8));
#39375=CARTESIAN_POINT('',(11.3535533905933,-3.30355339059329,-81.3));
#39376=CARTESIAN_POINT('',(11.5,-3.65710678118656,-81.3));
#39377=CARTESIAN_POINT('Origin',(11.,-3.65710678118656,-81.3));
#39378=CARTESIAN_POINT('',(11.5,-3.65710678118656,-84.8));
#39379=CARTESIAN_POINT('',(11.3535533905933,-3.30355339059329,0.));
#39380=CARTESIAN_POINT('Origin',(11.5,-4.75000000000001,-84.8));
#39381=CARTESIAN_POINT('',(11.5,-3.65710678118656,-81.3));
#39382=CARTESIAN_POINT('Origin',(8.05,-8.2,-84.8));
#39383=CARTESIAN_POINT('',(11.3535533905933,-4.89644660940673,-81.3));
#39384=CARTESIAN_POINT('Origin',(10.6288496112726,-3.28595639245914,-84.8));
#39385=CARTESIAN_POINT('',(10.6942336092596,-2.79024989380572,-81.3));
#39386=CARTESIAN_POINT('',(10.9824030018659,-2.93240300186586,-81.3));
#39387=CARTESIAN_POINT('Origin',(10.6288496112726,-3.28595639245914,-81.3));
#39388=CARTESIAN_POINT('',(10.9824030018659,-2.93240300186586,-84.8));
#39389=CARTESIAN_POINT('',(10.6942336092596,-2.79024989380572,-84.8));
#39390=CARTESIAN_POINT('Origin',(8.21904360754086,-0.876150388727407,-84.8));
#39391=CARTESIAN_POINT('',(8.57259699813413,-0.522596998134133,-81.3));
#39392=CARTESIAN_POINT('',(8.71475010619428,-0.81076639074037,-81.3));
#39393=CARTESIAN_POINT('Origin',(8.21904360754086,-0.876150388727407,-81.3));
#39394=CARTESIAN_POINT('',(8.71475010619428,-0.81076639074037,-84.8));
#39395=CARTESIAN_POINT('',(8.57259699813413,-0.522596998134133,0.));
#39396=CARTESIAN_POINT('Origin',(10.995,-0.509999999999999,-84.8));
#39397=CARTESIAN_POINT('Origin',(10.995,-0.509999999999999,-81.3));
#39398=CARTESIAN_POINT('Origin',(8.05,3.67394039744206E-16,-84.8));
#39399=CARTESIAN_POINT('',(-8.05,-1.60428730688303E-15,-81.3));
#39400=CARTESIAN_POINT('',(-8.05,-1.60428730688303E-15,-84.8));
#39401=CARTESIAN_POINT('',(8.05,3.67394039744206E-16,-81.3));
#39402=CARTESIAN_POINT('',(-8.05,-1.60428730688303E-15,-81.3));
#39403=CARTESIAN_POINT('',(8.05,3.67394039744206E-16,-84.8));
#39404=CARTESIAN_POINT('Origin',(8.05,3.67394039744206E-16,-84.8));
#39405=CARTESIAN_POINT('',(8.05,3.67394039744206E-16,-81.3));
#39406=CARTESIAN_POINT('Origin',(-8.21904360754086,-0.87615038872741,-84.8));
#39407=CARTESIAN_POINT('',(-8.71475010619428,-0.810766390740372,-81.3));
#39408=CARTESIAN_POINT('',(-8.57259699813413,-0.522596998134137,-81.3));
#39409=CARTESIAN_POINT('Origin',(-8.21904360754086,-0.87615038872741,-81.3));
#39410=CARTESIAN_POINT('',(-8.57259699813413,-0.522596998134137,-84.8));
#39411=CARTESIAN_POINT('',(-8.71475010619428,-0.810766390740372,-84.8));
#39412=CARTESIAN_POINT('Origin',(-10.6288496112726,-3.28595639245914,-84.8));
#39413=CARTESIAN_POINT('',(-10.9824030018659,-2.93240300186587,-81.3));
#39414=CARTESIAN_POINT('',(-10.6942336092596,-2.79024989380572,-81.3));
#39415=CARTESIAN_POINT('Origin',(-10.6288496112726,-3.28595639245914,-81.3));
#39416=CARTESIAN_POINT('',(-10.6942336092596,-2.79024989380572,-84.8));
#39417=CARTESIAN_POINT('',(-10.9824030018659,-2.93240300186587,0.));
#39418=CARTESIAN_POINT('Origin',(-10.995,-0.510000000000002,-84.8));
#39419=CARTESIAN_POINT('Origin',(-10.995,-0.510000000000002,-81.3));
#39420=CARTESIAN_POINT('Origin',(-11.,-3.65710678118656,-84.8));
#39421=CARTESIAN_POINT('',(-11.5,-3.65710678118656,-81.3));
#39422=CARTESIAN_POINT('',(-11.3535533905933,-3.30355339059329,-81.3));
#39423=CARTESIAN_POINT('Origin',(-11.,-3.65710678118656,-81.3));
#39424=CARTESIAN_POINT('',(-11.3535533905933,-3.30355339059329,-84.8));
#39425=CARTESIAN_POINT('',(-11.5,-3.65710678118656,0.));
#39426=CARTESIAN_POINT('Origin',(-11.,-4.54289321881346,-84.8));
#39427=CARTESIAN_POINT('',(-11.3535533905933,-4.89644660940674,-81.3));
#39428=CARTESIAN_POINT('',(-11.5,-4.54289321881346,-81.3));
#39429=CARTESIAN_POINT('Origin',(-11.,-4.54289321881346,-81.3));
#39430=CARTESIAN_POINT('',(-11.5,-4.54289321881346,-84.8));
#39431=CARTESIAN_POINT('',(-11.3535533905933,-4.89644660940674,0.));
#39432=CARTESIAN_POINT('Origin',(-11.5,-4.75000000000001,-84.8));
#39433=CARTESIAN_POINT('',(-11.5,-4.54289321881346,-81.3));
#39434=CARTESIAN_POINT('Origin',(-8.05,-1.60428730688303E-15,-84.8));
#39435=CARTESIAN_POINT('',(-11.3535533905933,-3.30355339059329,-81.3));
#39436=CARTESIAN_POINT('Origin',(-8.05,-1.60428730688303E-15,-84.8));
#39437=CARTESIAN_POINT('',(-8.57259699813413,-0.522596998134137,-81.3));
#39438=CARTESIAN_POINT('Origin',(-10.6288496112726,-4.91404360754086,-84.8));
#39439=CARTESIAN_POINT('',(-10.6942336092596,-5.40975010619428,-81.3));
#39440=CARTESIAN_POINT('',(-10.9824030018659,-5.26759699813413,-81.3));
#39441=CARTESIAN_POINT('Origin',(-10.6288496112726,-4.91404360754086,-81.3));
#39442=CARTESIAN_POINT('',(-10.9824030018659,-5.26759699813413,-84.8));
#39443=CARTESIAN_POINT('',(-10.6942336092596,-5.40975010619428,-84.8));
#39444=CARTESIAN_POINT('Origin',(-8.21904360754086,-7.32384961127259,-84.8));
#39445=CARTESIAN_POINT('',(-8.57259699813413,-7.67740300186587,-81.3));
#39446=CARTESIAN_POINT('',(-8.71475010619428,-7.38923360925963,-81.3));
#39447=CARTESIAN_POINT('Origin',(-8.21904360754086,-7.32384961127259,-81.3));
#39448=CARTESIAN_POINT('',(-8.71475010619428,-7.38923360925963,-84.8));
#39449=CARTESIAN_POINT('',(-8.57259699813413,-7.67740300186587,0.));
#39450=CARTESIAN_POINT('Origin',(-10.995,-7.69,-84.8));
#39451=CARTESIAN_POINT('Origin',(-10.995,-7.69,-81.3));
#39452=CARTESIAN_POINT('Origin',(-8.55,-8.40710678118654,-84.8));
#39453=CARTESIAN_POINT('',(-8.05,-8.40710678118654,-81.3));
#39454=CARTESIAN_POINT('',(-8.05,-8.40710678118654,-84.8));
#39455=CARTESIAN_POINT('',(-8.19644660940673,-8.05355339059327,-81.3));
#39456=CARTESIAN_POINT('Origin',(-8.55,-8.40710678118654,-81.3));
#39457=CARTESIAN_POINT('',(-8.19644660940673,-8.05355339059327,-84.8));
#39458=CARTESIAN_POINT('Origin',(-8.55,-12.0328932188134,-84.8));
#39459=CARTESIAN_POINT('',(-8.19644660940672,-12.3864466094067,-81.3));
#39460=CARTESIAN_POINT('',(-8.19644660940672,-12.3864466094067,-84.8));
#39461=CARTESIAN_POINT('',(-8.05,-12.0328932188134,-81.3));
#39462=CARTESIAN_POINT('Origin',(-8.55,-12.0328932188134,-81.3));
#39463=CARTESIAN_POINT('',(-8.05,-12.0328932188134,-84.8));
#39464=CARTESIAN_POINT('Origin',(-22.2,-16.5,-84.8));
#39465=CARTESIAN_POINT('',(-23.2,-15.5,-81.3));
#39466=CARTESIAN_POINT('',(-22.2,-16.5,-81.3));
#39467=CARTESIAN_POINT('',(-23.2,-15.5,-81.3));
#39468=CARTESIAN_POINT('',(-22.2,-16.5,-84.8));
#39469=CARTESIAN_POINT('',(-23.2,-15.5,-84.8));
#39470=CARTESIAN_POINT('Origin',(-23.2,-15.5,-84.8));
#39471=CARTESIAN_POINT('',(-23.2,12.,-81.3));
#39472=CARTESIAN_POINT('',(-23.2,12.,-81.3));
#39473=CARTESIAN_POINT('',(-23.2,12.,-84.8));
#39474=CARTESIAN_POINT('Origin',(-23.2,12.,-84.8));
#39475=CARTESIAN_POINT('',(-22.2,13.,-81.3));
#39476=CARTESIAN_POINT('',(-22.2,13.,-81.3));
#39477=CARTESIAN_POINT('',(-22.2,13.,-84.8));
#39478=CARTESIAN_POINT('Origin',(-22.2,13.,-84.8));
#39479=CARTESIAN_POINT('',(22.2,13.,-81.3));
#39480=CARTESIAN_POINT('Origin',(-23.,-16.5,-84.8));
#39481=CARTESIAN_POINT('',(-12.31,-16.5,-81.3));
#39482=CARTESIAN_POINT('',(-22.2,-16.5,-81.3));
#39483=CARTESIAN_POINT('',(-12.31,-16.5,-84.8));
#39484=CARTESIAN_POINT('Origin',(-12.31,-16.5,-84.8));
#39485=CARTESIAN_POINT('',(-12.31,-16.5,-81.3));
#39486=CARTESIAN_POINT('Origin',(-8.05,-12.24,-84.8));
#39487=CARTESIAN_POINT('',(-8.05,-12.0328932188134,-81.3));
#39488=CARTESIAN_POINT('Origin',(-8.05,-8.2,-84.8));
#39489=CARTESIAN_POINT('',(-8.19644660940673,-8.05355339059327,-81.3));
#39490=CARTESIAN_POINT('Origin',(-8.05,-8.2,-84.8));
#39491=CARTESIAN_POINT('',(-10.9824030018659,-5.26759699813413,-81.3));
#39492=CARTESIAN_POINT('Origin',(8.05,3.67394039744206E-16,-84.8));
#39493=CARTESIAN_POINT('',(10.9824030018659,-2.93240300186586,-81.3));
#39494=CARTESIAN_POINT('Origin',(8.05,-8.2,-84.8));
#39495=CARTESIAN_POINT('',(8.57259699813413,-7.67740300186587,-81.3));
#39496=CARTESIAN_POINT('Origin',(4.99999999999995,13.8,1.31418445149758E-15));
#39497=CARTESIAN_POINT('',(4.99999999999997,13.8,-81.3));
#39498=CARTESIAN_POINT('',(4.99999999999996,13.8,-81.3));
#39499=CARTESIAN_POINT('',(4.99999999999997,13.8,-81.3));
#39500=CARTESIAN_POINT('Origin',(-1.64657055886728E-14,13.8,4.08782152511659E-30));
#39501=CARTESIAN_POINT('',(-5.8,13.8,-81.3));
#39502=CARTESIAN_POINT('Origin',(-5.8,13.8,-81.3));
#39503=CARTESIAN_POINT('Origin',(4.99995,13.,-1.));
#39504=CARTESIAN_POINT('',(4.99995,8.,-1.));
#39505=CARTESIAN_POINT('',(4.99995,13.,-1.));
#39506=CARTESIAN_POINT('',(4.99995,8.,-1.));
#39507=CARTESIAN_POINT('Origin',(0.,8.,-1.));
#39508=CARTESIAN_POINT('',(-4.99995,8.,-1.));
#39509=CARTESIAN_POINT('Origin',(0.,8.,-1.));
#39510=CARTESIAN_POINT('',(-4.99995,8.,-1.));
#39511=CARTESIAN_POINT('Origin',(-4.99995,13.,-1.));
#39512=CARTESIAN_POINT('',(-4.99995,13.,-1.));
#39513=CARTESIAN_POINT('Origin',(0.,8.,-1.));
#39514=CARTESIAN_POINT('Origin',(-28.5,24.2065391822594,-19.9));
#39515=CARTESIAN_POINT('Origin',(-28.5,24.2065391822594,-64.9));
#39516=CARTESIAN_POINT('Origin',(28.5,24.2065391822594,-19.9));
#39517=CARTESIAN_POINT('Origin',(28.5,24.2065391822594,-64.9));
#66651=UNCERTAINTY_MEASURE_WITH_UNIT(LENGTH_MEASURE(0.01),#66722,
'DISTANCE_ACCURACY_VALUE',
'Maximum model space distance between geometric entities at asserted c
onnectivities');
#66680=UNCERTAINTY_MEASURE_WITH_UNIT(LENGTH_MEASURE(0.01),#66722,
'DISTANCE_ACCURACY_VALUE',
'Maximum model space distance between geometric entities at asserted c
onnectivities');
#66692=(
GEOMETRIC_REPRESENTATION_CONTEXT(3)
GLOBAL_UNCERTAINTY_ASSIGNED_CONTEXT((#66651))
GLOBAL_UNIT_ASSIGNED_CONTEXT((#66722,#66724,#66725))
REPRESENTATION_CONTEXT('','3D')
);
#66721=(
GEOMETRIC_REPRESENTATION_CONTEXT(3)
GLOBAL_UNCERTAINTY_ASSIGNED_CONTEXT((#66680))
GLOBAL_UNIT_ASSIGNED_CONTEXT((#66722,#66724,#66725))
REPRESENTATION_CONTEXT('','3D')
);
#66722=(
LENGTH_UNIT()
NAMED_UNIT(*)
SI_UNIT(.MILLI.,.METRE.)
);
#66724=(
NAMED_UNIT(*)
PLANE_ANGLE_UNIT()
SI_UNIT($,.RADIAN.)
);
#66725=(
NAMED_UNIT(*)
SI_UNIT($,.STERADIAN.)
SOLID_ANGLE_UNIT()
);
#66737=SHAPE_DEFINITION_REPRESENTATION(#66779,#66901);
#66779=PRODUCT_DEFINITION_SHAPE('',$,#66942);
#66901=SHAPE_REPRESENTATION('',(#26592),#66692);
#66930=PRODUCT_DEFINITION_CONTEXT('part definition',#67052,'design');
#66942=PRODUCT_DEFINITION('Linear Guide Slider','Linear Guide Slider',#66982,
#66930);
#66982=PRODUCT_DEFINITION_FORMATION('',$,#67065);
#67052=APPLICATION_CONTEXT(
'Core Data for Automotive Mechanical Design Process');
#67053=PRODUCT_CONTEXT('part definition',#67052,'mechanical');
#67065=PRODUCT('Linear Guide Slider','Linear Guide Slider',$,(#67053));
#67095=PRESENTATION_STYLE_ASSIGNMENT((#67097));
#67097=SURFACE_STYLE_USAGE(.BOTH.,#67099);
#67099=SURFACE_SIDE_STYLE('',(#67101));
#67101=SURFACE_STYLE_FILL_AREA(#67103);
#67103=FILL_AREA_STYLE('Opaque(202,209,238)',(#67105));
#67105=FILL_AREA_STYLE_COLOUR('Opaque(202,209,238)',#67107);
#67107=COLOUR_RGB('Opaque(202,209,238)',0.792156862745098,0.819607843137255,
0.933333333333333);
ENDSEC;
END-ISO-10303-21;
